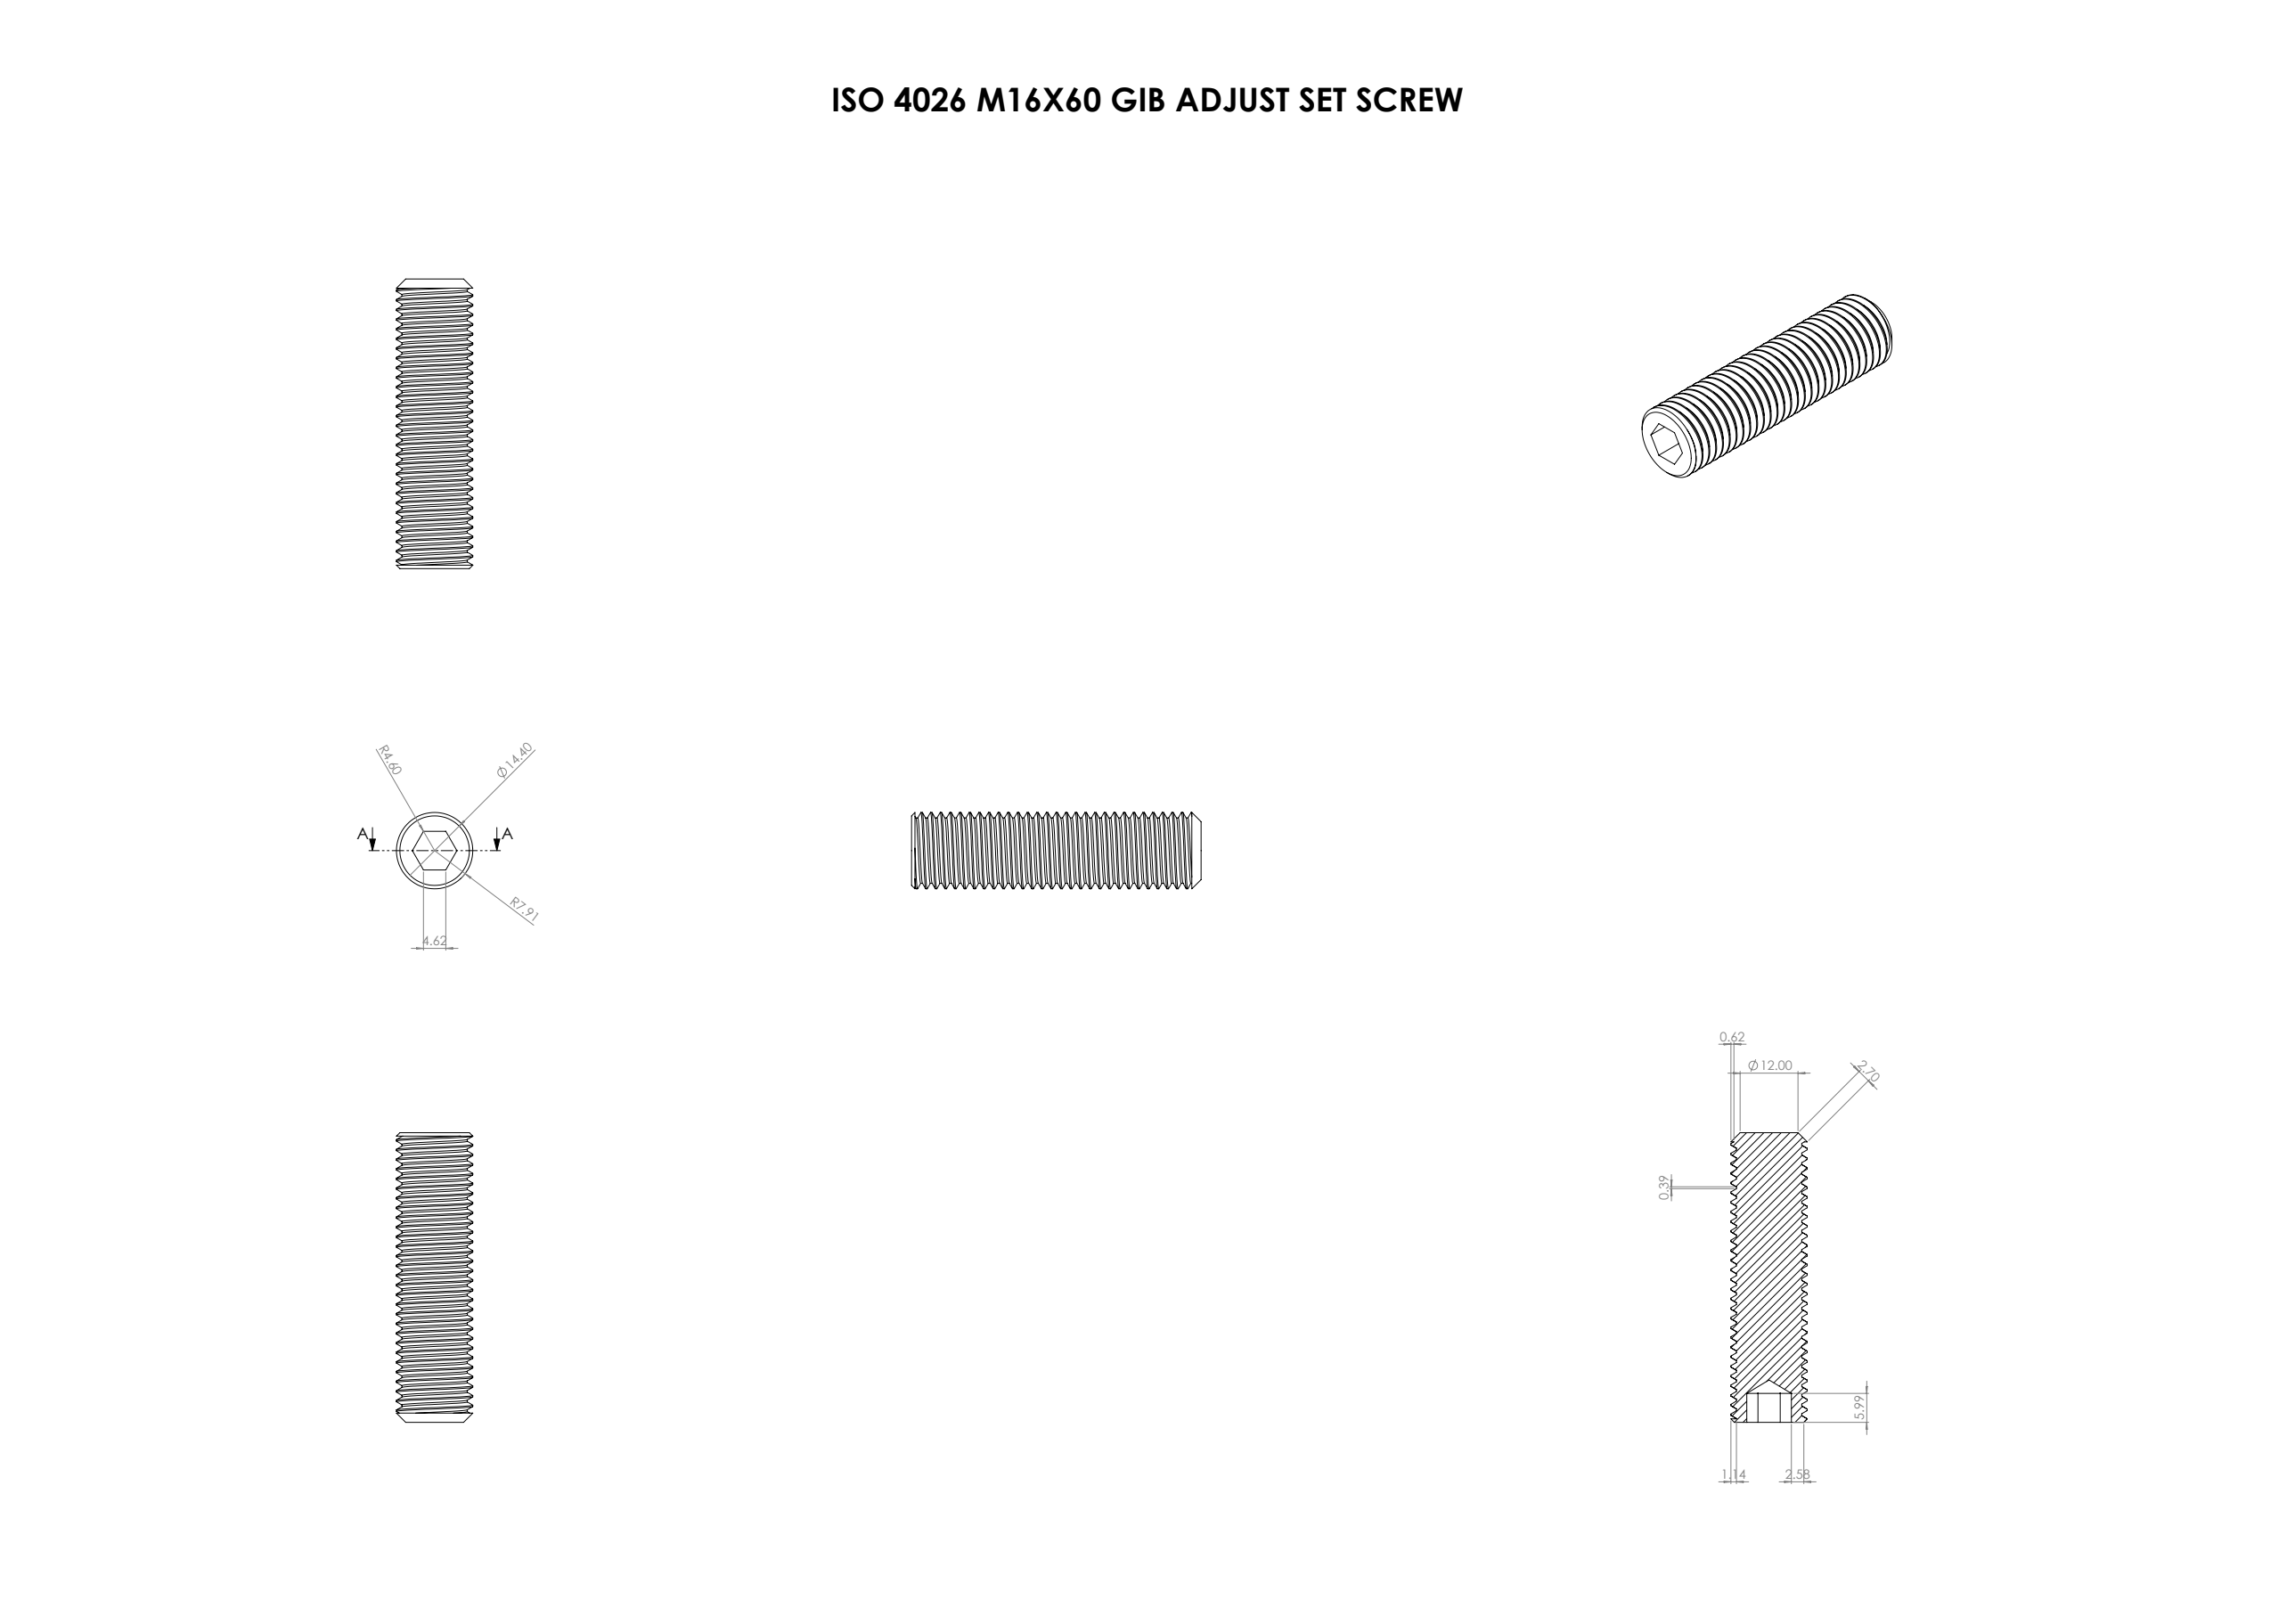
ISO-10303-21;
HEADER;
/* Generated by software containing ST-Developer
 * from STEP Tools, Inc. (www.steptools.com) 
 */

FILE_DESCRIPTION(
/* description */ (''),
/* implementation_level */ '2;1');

FILE_NAME(
/* name */ '11_ISO_4026_M16x60_Gib_Adjust_Set_Screw.step',
/* time_stamp */ '2026-10-19T23:58:09-07:00',
/* author */ (''),
/* organization */ (''),
/* preprocessor_version */ 'ST-DEVELOPER v20.2',
/* originating_system */ 'Autodesk Translation Framework v15.15.0.0',
/* authorisation */ '');

FILE_SCHEMA (('AP203_CONFIGURATION_CONTROLLED_3D_DESIGN_OF_MECHANICAL_PARTS_AND_ASSEMBLIES_MIM_LF { 1 0 10303 203 3 1 4 }',
'AUTOMOTIVE_DESIGN { 1 0 10303 214 3 1 1 }','INTEGRATED_CNC_SCHEMA','MODEL_BASED_INTEGRATED_MANUFACTURING_SCHEMA',
'PROCESS_PLANNING_SCHEMA','AP242_MANAGED_MODEL_BASED_3D_ENGINEERING_MIM_LF { 1 0 10303 442 3 1 4 }'));
ENDSEC;

DATA;
#10=MECHANICAL_DESIGN_GEOMETRIC_PRESENTATION_REPRESENTATION('',(#414),#70757);
#215=(
BOUNDED_CURVE()
B_SPLINE_CURVE(2,(#54486,#54487,#54488),.UNSPECIFIED.,.F.,.F.)
B_SPLINE_CURVE_WITH_KNOTS((3,3),(0.,0.00348603246849772),.UNSPECIFIED.)
CURVE()
GEOMETRIC_REPRESENTATION_ITEM()
RATIONAL_B_SPLINE_CURVE((1.,1.00000655818292,1.))
REPRESENTATION_ITEM('')
);
#216=(
BOUNDED_CURVE()
B_SPLINE_CURVE(2,(#54490,#54491,#54492),.UNSPECIFIED.,.F.,.F.)
B_SPLINE_CURVE_WITH_KNOTS((3,3),(0.,0.0034860324684977),.UNSPECIFIED.)
CURVE()
GEOMETRIC_REPRESENTATION_ITEM()
RATIONAL_B_SPLINE_CURVE((1.,1.00000655824651,1.))
REPRESENTATION_ITEM('')
);
#217=(
BOUNDED_CURVE()
B_SPLINE_CURVE(2,(#54495,#54496,#54497),.UNSPECIFIED.,.F.,.F.)
B_SPLINE_CURVE_WITH_KNOTS((3,3),(0.,0.00348603246849777),.UNSPECIFIED.)
CURVE()
GEOMETRIC_REPRESENTATION_ITEM()
RATIONAL_B_SPLINE_CURVE((1.,1.00000655828125,1.))
REPRESENTATION_ITEM('')
);
#218=(
BOUNDED_CURVE()
B_SPLINE_CURVE(2,(#54499,#54500,#54501),.UNSPECIFIED.,.F.,.F.)
B_SPLINE_CURVE_WITH_KNOTS((3,3),(0.,0.00348603246849785),.UNSPECIFIED.)
CURVE()
GEOMETRIC_REPRESENTATION_ITEM()
RATIONAL_B_SPLINE_CURVE((1.,1.00000655858972,1.))
REPRESENTATION_ITEM('')
);
#219=(
BOUNDED_CURVE()
B_SPLINE_CURVE(2,(#54504,#54505,#54506),.UNSPECIFIED.,.F.,.F.)
B_SPLINE_CURVE_WITH_KNOTS((3,3),(0.,0.00348603246849743),.UNSPECIFIED.)
CURVE()
GEOMETRIC_REPRESENTATION_ITEM()
RATIONAL_B_SPLINE_CURVE((1.,1.00000655826316,1.))
REPRESENTATION_ITEM('')
);
#220=(
BOUNDED_CURVE()
B_SPLINE_CURVE(2,(#54508,#54509,#54510),.UNSPECIFIED.,.F.,.F.)
B_SPLINE_CURVE_WITH_KNOTS((3,3),(0.,0.00348603246849747),.UNSPECIFIED.)
CURVE()
GEOMETRIC_REPRESENTATION_ITEM()
RATIONAL_B_SPLINE_CURVE((1.,1.00000655837246,1.))
REPRESENTATION_ITEM('')
);
#221=(
BOUNDED_CURVE()
B_SPLINE_CURVE(2,(#54513,#54514,#54515),.UNSPECIFIED.,.F.,.F.)
B_SPLINE_CURVE_WITH_KNOTS((3,3),(0.,0.00348603246849727),.UNSPECIFIED.)
CURVE()
GEOMETRIC_REPRESENTATION_ITEM()
RATIONAL_B_SPLINE_CURVE((1.,1.00000655774933,1.))
REPRESENTATION_ITEM('')
);
#222=(
BOUNDED_CURVE()
B_SPLINE_CURVE(2,(#54517,#54518,#54519),.UNSPECIFIED.,.F.,.F.)
B_SPLINE_CURVE_WITH_KNOTS((3,3),(0.,0.00348603246849747),.UNSPECIFIED.)
CURVE()
GEOMETRIC_REPRESENTATION_ITEM()
RATIONAL_B_SPLINE_CURVE((1.,1.00000655778188,1.))
REPRESENTATION_ITEM('')
);
#223=(
BOUNDED_CURVE()
B_SPLINE_CURVE(2,(#54522,#54523,#54524),.UNSPECIFIED.,.F.,.F.)
B_SPLINE_CURVE_WITH_KNOTS((3,3),(0.,0.00348603246849769),.UNSPECIFIED.)
CURVE()
GEOMETRIC_REPRESENTATION_ITEM()
RATIONAL_B_SPLINE_CURVE((1.,1.00000655825998,1.))
REPRESENTATION_ITEM('')
);
#224=(
BOUNDED_CURVE()
B_SPLINE_CURVE(2,(#54526,#54527,#54528),.UNSPECIFIED.,.F.,.F.)
B_SPLINE_CURVE_WITH_KNOTS((3,3),(0.,0.00348603246849761),.UNSPECIFIED.)
CURVE()
GEOMETRIC_REPRESENTATION_ITEM()
RATIONAL_B_SPLINE_CURVE((1.,1.00000655838487,1.))
REPRESENTATION_ITEM('')
);
#225=(
BOUNDED_CURVE()
B_SPLINE_CURVE(2,(#54531,#54532,#54533),.UNSPECIFIED.,.F.,.F.)
B_SPLINE_CURVE_WITH_KNOTS((3,3),(0.,0.00348603246849764),.UNSPECIFIED.)
CURVE()
GEOMETRIC_REPRESENTATION_ITEM()
RATIONAL_B_SPLINE_CURVE((1.,1.00000655822052,1.))
REPRESENTATION_ITEM('')
);
#226=(
BOUNDED_CURVE()
B_SPLINE_CURVE(2,(#54535,#54536,#54537),.UNSPECIFIED.,.F.,.F.)
B_SPLINE_CURVE_WITH_KNOTS((3,3),(0.,0.00348603246849749),.UNSPECIFIED.)
CURVE()
GEOMETRIC_REPRESENTATION_ITEM()
RATIONAL_B_SPLINE_CURVE((1.,1.00000655832735,1.))
REPRESENTATION_ITEM('')
);
#276=B_SPLINE_SURFACE_WITH_KNOTS('',3,3,((#51283,#51284,#51285,#51286,#51287,
#51288,#51289,#51290,#51291,#51292,#51293,#51294,#51295,#51296,#51297,#51298,
#51299,#51300,#51301,#51302,#51303,#51304,#51305,#51306,#51307,#51308,#51309,
#51310,#51311,#51312,#51313,#51314,#51315,#51316,#51317,#51318,#51319,#51320,
#51321,#51322,#51323,#51324,#51325,#51326,#51327,#51328,#51329,#51330,#51331,
#51332,#51333,#51334,#51335,#51336,#51337,#51338,#51339,#51340,#51341,#51342,
#51343,#51344,#51345,#51346,#51347,#51348,#51349,#51350,#51351,#51352,#51353,
#51354,#51355,#51356,#51357,#51358,#51359,#51360,#51361,#51362,#51363,#51364,
#51365,#51366,#51367,#51368,#51369,#51370,#51371,#51372,#51373,#51374,#51375,
#51376,#51377,#51378,#51379,#51380,#51381,#51382,#51383,#51384,#51385,#51386,
#51387,#51388,#51389,#51390,#51391,#51392,#51393,#51394,#51395,#51396,#51397,
#51398,#51399,#51400,#51401,#51402,#51403,#51404,#51405,#51406,#51407,#51408,
#51409,#51410,#51411,#51412,#51413,#51414,#51415,#51416,#51417,#51418,#51419,
#51420,#51421,#51422,#51423,#51424,#51425,#51426,#51427,#51428,#51429,#51430,
#51431,#51432,#51433,#51434,#51435,#51436,#51437,#51438,#51439,#51440,#51441,
#51442,#51443,#51444,#51445,#51446,#51447,#51448,#51449,#51450,#51451,#51452,
#51453,#51454,#51455,#51456,#51457,#51458,#51459,#51460,#51461,#51462,#51463,
#51464,#51465,#51466,#51467,#51468,#51469,#51470,#51471,#51472,#51473,#51474,
#51475,#51476,#51477,#51478,#51479,#51480,#51481,#51482,#51483,#51484,#51485,
#51486,#51487,#51488,#51489,#51490,#51491,#51492,#51493,#51494,#51495,#51496,
#51497,#51498,#51499,#51500,#51501,#51502,#51503,#51504,#51505,#51506,#51507,
#51508,#51509,#51510,#51511,#51512,#51513,#51514,#51515,#51516,#51517,#51518,
#51519,#51520,#51521,#51522,#51523,#51524,#51525,#51526,#51527,#51528,#51529,
#51530,#51531,#51532,#51533,#51534,#51535,#51536,#51537,#51538,#51539,#51540,
#51541,#51542,#51543,#51544,#51545,#51546,#51547,#51548,#51549,#51550,#51551,
#51552,#51553,#51554,#51555,#51556,#51557,#51558,#51559,#51560,#51561,#51562,
#51563,#51564,#51565,#51566,#51567,#51568,#51569,#51570,#51571,#51572,#51573,
#51574,#51575,#51576,#51577,#51578,#51579,#51580,#51581,#51582,#51583,#51584,
#51585,#51586,#51587,#51588,#51589,#51590,#51591,#51592,#51593,#51594,#51595,
#51596,#51597,#51598,#51599,#51600,#51601,#51602,#51603,#51604,#51605,#51606,
#51607,#51608,#51609,#51610,#51611,#51612,#51613,#51614,#51615,#51616,#51617,
#51618,#51619,#51620,#51621,#51622,#51623,#51624,#51625,#51626,#51627,#51628,
#51629,#51630,#51631,#51632,#51633,#51634,#51635,#51636,#51637,#51638,#51639,
#51640,#51641,#51642,#51643,#51644,#51645,#51646,#51647,#51648,#51649,#51650,
#51651),(#51652,#51653,#51654,#51655,#51656,#51657,#51658,#51659,#51660,
#51661,#51662,#51663,#51664,#51665,#51666,#51667,#51668,#51669,#51670,#51671,
#51672,#51673,#51674,#51675,#51676,#51677,#51678,#51679,#51680,#51681,#51682,
#51683,#51684,#51685,#51686,#51687,#51688,#51689,#51690,#51691,#51692,#51693,
#51694,#51695,#51696,#51697,#51698,#51699,#51700,#51701,#51702,#51703,#51704,
#51705,#51706,#51707,#51708,#51709,#51710,#51711,#51712,#51713,#51714,#51715,
#51716,#51717,#51718,#51719,#51720,#51721,#51722,#51723,#51724,#51725,#51726,
#51727,#51728,#51729,#51730,#51731,#51732,#51733,#51734,#51735,#51736,#51737,
#51738,#51739,#51740,#51741,#51742,#51743,#51744,#51745,#51746,#51747,#51748,
#51749,#51750,#51751,#51752,#51753,#51754,#51755,#51756,#51757,#51758,#51759,
#51760,#51761,#51762,#51763,#51764,#51765,#51766,#51767,#51768,#51769,#51770,
#51771,#51772,#51773,#51774,#51775,#51776,#51777,#51778,#51779,#51780,#51781,
#51782,#51783,#51784,#51785,#51786,#51787,#51788,#51789,#51790,#51791,#51792,
#51793,#51794,#51795,#51796,#51797,#51798,#51799,#51800,#51801,#51802,#51803,
#51804,#51805,#51806,#51807,#51808,#51809,#51810,#51811,#51812,#51813,#51814,
#51815,#51816,#51817,#51818,#51819,#51820,#51821,#51822,#51823,#51824,#51825,
#51826,#51827,#51828,#51829,#51830,#51831,#51832,#51833,#51834,#51835,#51836,
#51837,#51838,#51839,#51840,#51841,#51842,#51843,#51844,#51845,#51846,#51847,
#51848,#51849,#51850,#51851,#51852,#51853,#51854,#51855,#51856,#51857,#51858,
#51859,#51860,#51861,#51862,#51863,#51864,#51865,#51866,#51867,#51868,#51869,
#51870,#51871,#51872,#51873,#51874,#51875,#51876,#51877,#51878,#51879,#51880,
#51881,#51882,#51883,#51884,#51885,#51886,#51887,#51888,#51889,#51890,#51891,
#51892,#51893,#51894,#51895,#51896,#51897,#51898,#51899,#51900,#51901,#51902,
#51903,#51904,#51905,#51906,#51907,#51908,#51909,#51910,#51911,#51912,#51913,
#51914,#51915,#51916,#51917,#51918,#51919,#51920,#51921,#51922,#51923,#51924,
#51925,#51926,#51927,#51928,#51929,#51930,#51931,#51932,#51933,#51934,#51935,
#51936,#51937,#51938,#51939,#51940,#51941,#51942,#51943,#51944,#51945,#51946,
#51947,#51948,#51949,#51950,#51951,#51952,#51953,#51954,#51955,#51956,#51957,
#51958,#51959,#51960,#51961,#51962,#51963,#51964,#51965,#51966,#51967,#51968,
#51969,#51970,#51971,#51972,#51973,#51974,#51975,#51976,#51977,#51978,#51979,
#51980,#51981,#51982,#51983,#51984,#51985,#51986,#51987,#51988,#51989,#51990,
#51991,#51992,#51993,#51994,#51995,#51996,#51997,#51998,#51999,#52000,#52001,
#52002,#52003,#52004,#52005,#52006,#52007,#52008,#52009,#52010,#52011,#52012,
#52013,#52014,#52015,#52016,#52017,#52018,#52019,#52020),(#52021,#52022,
#52023,#52024,#52025,#52026,#52027,#52028,#52029,#52030,#52031,#52032,#52033,
#52034,#52035,#52036,#52037,#52038,#52039,#52040,#52041,#52042,#52043,#52044,
#52045,#52046,#52047,#52048,#52049,#52050,#52051,#52052,#52053,#52054,#52055,
#52056,#52057,#52058,#52059,#52060,#52061,#52062,#52063,#52064,#52065,#52066,
#52067,#52068,#52069,#52070,#52071,#52072,#52073,#52074,#52075,#52076,#52077,
#52078,#52079,#52080,#52081,#52082,#52083,#52084,#52085,#52086,#52087,#52088,
#52089,#52090,#52091,#52092,#52093,#52094,#52095,#52096,#52097,#52098,#52099,
#52100,#52101,#52102,#52103,#52104,#52105,#52106,#52107,#52108,#52109,#52110,
#52111,#52112,#52113,#52114,#52115,#52116,#52117,#52118,#52119,#52120,#52121,
#52122,#52123,#52124,#52125,#52126,#52127,#52128,#52129,#52130,#52131,#52132,
#52133,#52134,#52135,#52136,#52137,#52138,#52139,#52140,#52141,#52142,#52143,
#52144,#52145,#52146,#52147,#52148,#52149,#52150,#52151,#52152,#52153,#52154,
#52155,#52156,#52157,#52158,#52159,#52160,#52161,#52162,#52163,#52164,#52165,
#52166,#52167,#52168,#52169,#52170,#52171,#52172,#52173,#52174,#52175,#52176,
#52177,#52178,#52179,#52180,#52181,#52182,#52183,#52184,#52185,#52186,#52187,
#52188,#52189,#52190,#52191,#52192,#52193,#52194,#52195,#52196,#52197,#52198,
#52199,#52200,#52201,#52202,#52203,#52204,#52205,#52206,#52207,#52208,#52209,
#52210,#52211,#52212,#52213,#52214,#52215,#52216,#52217,#52218,#52219,#52220,
#52221,#52222,#52223,#52224,#52225,#52226,#52227,#52228,#52229,#52230,#52231,
#52232,#52233,#52234,#52235,#52236,#52237,#52238,#52239,#52240,#52241,#52242,
#52243,#52244,#52245,#52246,#52247,#52248,#52249,#52250,#52251,#52252,#52253,
#52254,#52255,#52256,#52257,#52258,#52259,#52260,#52261,#52262,#52263,#52264,
#52265,#52266,#52267,#52268,#52269,#52270,#52271,#52272,#52273,#52274,#52275,
#52276,#52277,#52278,#52279,#52280,#52281,#52282,#52283,#52284,#52285,#52286,
#52287,#52288,#52289,#52290,#52291,#52292,#52293,#52294,#52295,#52296,#52297,
#52298,#52299,#52300,#52301,#52302,#52303,#52304,#52305,#52306,#52307,#52308,
#52309,#52310,#52311,#52312,#52313,#52314,#52315,#52316,#52317,#52318,#52319,
#52320,#52321,#52322,#52323,#52324,#52325,#52326,#52327,#52328,#52329,#52330,
#52331,#52332,#52333,#52334,#52335,#52336,#52337,#52338,#52339,#52340,#52341,
#52342,#52343,#52344,#52345,#52346,#52347,#52348,#52349,#52350,#52351,#52352,
#52353,#52354,#52355,#52356,#52357,#52358,#52359,#52360,#52361,#52362,#52363,
#52364,#52365,#52366,#52367,#52368,#52369,#52370,#52371,#52372,#52373,#52374,
#52375,#52376,#52377,#52378,#52379,#52380,#52381,#52382,#52383,#52384,#52385,
#52386,#52387,#52388,#52389),(#52390,#52391,#52392,#52393,#52394,#52395,
#52396,#52397,#52398,#52399,#52400,#52401,#52402,#52403,#52404,#52405,#52406,
#52407,#52408,#52409,#52410,#52411,#52412,#52413,#52414,#52415,#52416,#52417,
#52418,#52419,#52420,#52421,#52422,#52423,#52424,#52425,#52426,#52427,#52428,
#52429,#52430,#52431,#52432,#52433,#52434,#52435,#52436,#52437,#52438,#52439,
#52440,#52441,#52442,#52443,#52444,#52445,#52446,#52447,#52448,#52449,#52450,
#52451,#52452,#52453,#52454,#52455,#52456,#52457,#52458,#52459,#52460,#52461,
#52462,#52463,#52464,#52465,#52466,#52467,#52468,#52469,#52470,#52471,#52472,
#52473,#52474,#52475,#52476,#52477,#52478,#52479,#52480,#52481,#52482,#52483,
#52484,#52485,#52486,#52487,#52488,#52489,#52490,#52491,#52492,#52493,#52494,
#52495,#52496,#52497,#52498,#52499,#52500,#52501,#52502,#52503,#52504,#52505,
#52506,#52507,#52508,#52509,#52510,#52511,#52512,#52513,#52514,#52515,#52516,
#52517,#52518,#52519,#52520,#52521,#52522,#52523,#52524,#52525,#52526,#52527,
#52528,#52529,#52530,#52531,#52532,#52533,#52534,#52535,#52536,#52537,#52538,
#52539,#52540,#52541,#52542,#52543,#52544,#52545,#52546,#52547,#52548,#52549,
#52550,#52551,#52552,#52553,#52554,#52555,#52556,#52557,#52558,#52559,#52560,
#52561,#52562,#52563,#52564,#52565,#52566,#52567,#52568,#52569,#52570,#52571,
#52572,#52573,#52574,#52575,#52576,#52577,#52578,#52579,#52580,#52581,#52582,
#52583,#52584,#52585,#52586,#52587,#52588,#52589,#52590,#52591,#52592,#52593,
#52594,#52595,#52596,#52597,#52598,#52599,#52600,#52601,#52602,#52603,#52604,
#52605,#52606,#52607,#52608,#52609,#52610,#52611,#52612,#52613,#52614,#52615,
#52616,#52617,#52618,#52619,#52620,#52621,#52622,#52623,#52624,#52625,#52626,
#52627,#52628,#52629,#52630,#52631,#52632,#52633,#52634,#52635,#52636,#52637,
#52638,#52639,#52640,#52641,#52642,#52643,#52644,#52645,#52646,#52647,#52648,
#52649,#52650,#52651,#52652,#52653,#52654,#52655,#52656,#52657,#52658,#52659,
#52660,#52661,#52662,#52663,#52664,#52665,#52666,#52667,#52668,#52669,#52670,
#52671,#52672,#52673,#52674,#52675,#52676,#52677,#52678,#52679,#52680,#52681,
#52682,#52683,#52684,#52685,#52686,#52687,#52688,#52689,#52690,#52691,#52692,
#52693,#52694,#52695,#52696,#52697,#52698,#52699,#52700,#52701,#52702,#52703,
#52704,#52705,#52706,#52707,#52708,#52709,#52710,#52711,#52712,#52713,#52714,
#52715,#52716,#52717,#52718,#52719,#52720,#52721,#52722,#52723,#52724,#52725,
#52726,#52727,#52728,#52729,#52730,#52731,#52732,#52733,#52734,#52735,#52736,
#52737,#52738,#52739,#52740,#52741,#52742,#52743,#52744,#52745,#52746,#52747,
#52748,#52749,#52750,#52751,#52752,#52753,#52754,#52755,#52756,#52757,#52758)),
 .UNSPECIFIED.,.F.,.F.,.F.,(4,4),(4,1,1,1,1,1,1,1,1,1,1,1,1,1,1,1,1,1,1,
1,1,1,1,1,1,1,1,1,1,1,1,1,1,1,1,1,1,1,1,1,1,1,1,1,1,1,1,1,1,1,1,1,1,1,1,
1,1,1,1,1,1,1,1,1,1,1,1,1,1,1,1,1,1,1,1,1,1,1,1,1,1,1,1,1,1,1,1,1,1,1,1,
1,1,1,1,1,1,1,1,1,1,1,1,1,1,1,1,1,1,1,1,1,1,1,1,1,1,1,1,1,1,1,1,1,1,1,1,
1,1,1,1,1,1,1,1,1,1,1,1,1,1,1,1,1,1,1,1,1,1,1,1,1,1,1,1,1,1,1,1,1,1,1,1,
1,1,1,1,1,1,1,1,1,1,1,1,1,1,1,1,1,1,1,1,1,1,1,1,1,1,1,1,1,1,1,1,1,1,1,1,
1,1,1,1,1,1,1,1,1,1,1,1,1,1,1,1,1,1,1,1,1,1,1,1,1,1,1,1,1,1,1,1,1,1,1,1,
1,1,1,1,1,1,1,1,1,1,1,1,1,1,1,1,1,1,1,1,1,1,1,1,1,1,1,1,1,1,1,1,1,1,1,1,
1,1,1,1,1,1,1,1,1,1,1,1,1,1,1,1,1,1,1,1,1,1,1,1,1,1,1,1,1,1,1,1,1,1,1,1,
1,1,1,1,1,1,1,1,1,1,1,1,1,1,1,1,1,1,1,1,1,1,1,1,1,1,1,1,1,1,1,1,1,1,1,1,
1,1,1,1,1,1,1,1,1,1,1,1,1,1,1,1,1,1,1,1,1,1,1,4),(0.,0.132097741590586),
(8.30112925462635,8.79930764192242,9.29748602921848,9.79566441651454,10.2938428038106,
10.7920211911067,11.2901995784027,11.7883779656988,12.2865563529949,12.7847347402909,
13.282913127587,13.781091514883,14.2792699021791,14.7774482894752,15.2756266767712,
15.7738050640673,16.2719834513634,16.7701618386594,17.2683402259555,17.7665186132516,
18.2646970005476,18.7628753878437,19.2610537751397,19.7592321624358,20.2574105497319,
20.7555889370279,21.253767324324,21.7519457116201,22.2501240989161,22.7483024862122,
23.2464808735082,23.7446592608043,24.2428376481004,24.7410160353964,25.2391944226925,
25.7373728099886,26.2355511972846,26.7337295845807,27.2319079718768,27.7300863591728,
28.2282647464689,28.7264431337649,29.224621521061,29.7227999083571,30.2209782956531,
30.7191566829492,31.2173350702453,31.7155134575413,32.2136918448374,32.7118702321334,
33.2100486194295,33.7082270067256,34.2064053940216,34.7045837813177,35.2027621686138,
35.7009405559098,36.1991189432059,36.697297330502,37.195475717798,37.6936541050941,
38.1918324923901,38.6900108796862,39.1881892669823,39.6863676542783,40.1845460415744,
40.6827244288705,41.1809028161665,41.6790812034626,42.1772595907587,42.6754379780547,
43.1736163653508,43.6717947526468,44.1699731399429,44.668151527239,45.166329914535,
45.6645083018311,46.1626866891272,46.6608650764232,47.1590434637193,47.6572218510153,
48.1554002383114,48.6535786256075,49.1517570129035,49.6499354001996,50.1481137874957,
50.6462921747917,51.1444705620878,51.6426489493839,52.1408273366799,52.639005723976,
53.137184111272,53.6353624985681,54.1335408858642,54.6317192731602,55.1298976604563,
55.6280760477524,56.1262544350484,56.6244328223445,57.1226112096405,57.6207895969366,
58.1189679842327,58.6171463715287,59.1153247588248,59.6135031461209,60.1116815334169,
60.609859920713,61.108038308009,61.6062166953051,62.1043950826012,62.6025734698972,
63.1007518571933,63.5989302444894,64.0971086317854,64.5952870190815,65.0934654063776,
65.5916437936736,66.0898221809697,66.5880005682658,67.0861789555618,67.5843573428579,
68.0825357301539,68.58071411745,69.0788925047461,69.5770708920421,70.0752492793382,
70.5734276666342,71.0716060539303,71.5697844412264,72.0679628285224,72.5661412158185,
73.0643196031146,73.5624979904106,74.0606763777067,74.5588547650028,75.0570331522988,
75.5552115395949,76.053389926891,76.551568314187,77.0497467014831,77.5479250887791,
78.0461034760752,78.5442818633713,79.0424602506673,79.5406386379634,80.0388170252594,
80.5369954125555,81.0351737998516,81.5333521871476,82.0315305744437,82.5297089617398,
83.0278873490358,83.5260657363319,84.024244123628,84.522422510924,85.0206008982201,
85.5187792855161,86.0169576728122,86.5151360601083,87.0133144474043,87.5114928347004,
88.0096712219965,88.5078496092925,89.0060279965886,89.5042063838847,90.0023847711807,
90.5005631584768,90.9987415457728,91.4969199330689,91.995098320365,92.493276707661,
92.9914550949571,93.4896334822532,93.9878118695492,94.4859902568453,94.9841686441413,
95.4823470314374,95.9805254187335,96.4787038060295,96.9768821933256,97.4750605806217,
97.9732389679177,98.4714173552138,98.9695957425099,99.4677741298059,99.965952517102,
100.464130904398,100.962309291694,101.46048767899,101.958666066286,102.456844453582,
102.955022840878,103.453201228174,103.95137961547,104.449558002767,104.947736390063,
105.445914777359,105.944093164655,106.442271551951,106.940449939247,107.438628326543,
107.936806713839,108.434985101135,108.933163488431,109.431341875727,109.929520263023,
110.427698650319,110.925877037615,111.424055424911,111.922233812207,112.420412199504,
112.9185905868,113.416768974096,113.914947361392,114.413125748688,114.911304135984,
115.40948252328,115.907660910576,116.405839297872,116.904017685168,117.402196072464,
117.90037445976,118.398552847056,118.896731234352,119.394909621648,119.893088008945,
120.391266396241,120.889444783537,121.387623170833,121.885801558129,122.383979945425,
122.882158332721,123.380336720017,123.878515107313,124.376693494609,124.874871881905,
125.373050269201,125.871228656497,126.369407043793,126.867585431089,127.365763818385,
127.863942205682,128.362120592978,128.860298980274,129.35847736757,129.856655754866,
130.354834142162,130.853012529458,131.351190916754,131.84936930405,132.347547691346,
132.845726078642,133.343904465938,133.842082853234,134.34026124053,134.838439627826,
135.336618015122,135.834796402419,136.332974789715,136.831153177011,137.329331564307,
137.827509951603,138.325688338899,138.823866726195,139.322045113491,139.820223500787,
140.318401888083,140.816580275379,141.314758662675,141.812937049971,142.311115437267,
142.809293824563,143.307472211859,143.805650599156,144.303828986452,144.802007373748,
145.300185761044,145.79836414834,146.296542535636,146.794720922932,147.292899310228,
147.791077697524,148.28925608482,148.787434472116,149.285612859412,149.783791246708,
150.281969634004,150.7801480213,151.278326408596,151.776504795893,152.274683183189,
152.772861570485,153.271039957781,153.769218345077,154.267396732373,154.765575119669,
155.263753506965,155.761931894261,156.260110281557,156.758288668853,157.256467056149,
157.754645443445,158.252823830741,158.751002218037,159.249180605333,159.74735899263,
160.245537379926,160.743715767222,161.241894154518,161.740072541814,162.23825092911,
162.736429316406,163.234607703702,163.732786090998,164.230964478294,164.72914286559,
165.227321252886,165.725499640182,166.223678027478,166.721856414774,167.220034802071,
167.718213189367,168.216391576663,168.714569963959,169.212748351255,169.710926738551,
170.209105125847,170.707283513143,171.205461900439,171.703640287735,172.201818675031,
172.699997062327,173.198175449623,173.696353836919,174.194532224215,174.692710611511,
175.190888998808,175.689067386104,176.1872457734,176.685424160696,177.183602547992,
177.681780935288,178.179959322584,178.67813770988,179.176316097176,179.674494484472,
180.172672871768,180.670851259064,181.16902964636,181.667208033656,182.165386420952,
182.663564808248,183.161743195545,183.659921582841,184.158099970137,184.656278357433,
185.154456744729,185.652635132025,186.150813519321,186.648991906617,187.147170293913,
187.645348681209,188.143527068505,188.641705455801,189.139883843097,189.638062230393,
190.136240617689,190.634419004985),.UNSPECIFIED.);
#277=B_SPLINE_SURFACE_WITH_KNOTS('',3,3,((#52964,#52965,#52966,#52967,#52968,
#52969,#52970,#52971,#52972,#52973,#52974,#52975,#52976,#52977,#52978,#52979,
#52980,#52981,#52982,#52983,#52984,#52985,#52986,#52987,#52988,#52989,#52990,
#52991,#52992,#52993,#52994,#52995,#52996,#52997,#52998,#52999,#53000,#53001,
#53002,#53003,#53004,#53005,#53006,#53007,#53008,#53009,#53010,#53011,#53012,
#53013,#53014,#53015,#53016,#53017,#53018,#53019,#53020,#53021,#53022,#53023,
#53024,#53025,#53026,#53027,#53028,#53029,#53030,#53031,#53032,#53033,#53034,
#53035,#53036,#53037,#53038,#53039,#53040,#53041,#53042,#53043,#53044,#53045,
#53046,#53047,#53048,#53049,#53050,#53051,#53052,#53053,#53054,#53055,#53056,
#53057,#53058,#53059,#53060,#53061,#53062,#53063,#53064,#53065,#53066,#53067,
#53068,#53069,#53070,#53071,#53072,#53073,#53074,#53075,#53076,#53077,#53078,
#53079,#53080,#53081,#53082,#53083,#53084,#53085,#53086,#53087,#53088,#53089,
#53090,#53091,#53092,#53093,#53094,#53095,#53096,#53097,#53098,#53099,#53100,
#53101,#53102,#53103,#53104,#53105,#53106,#53107,#53108,#53109,#53110,#53111,
#53112,#53113,#53114,#53115,#53116,#53117,#53118,#53119,#53120,#53121,#53122,
#53123,#53124,#53125,#53126,#53127,#53128,#53129,#53130,#53131,#53132,#53133,
#53134,#53135,#53136,#53137,#53138,#53139,#53140,#53141,#53142,#53143,#53144,
#53145,#53146,#53147,#53148,#53149,#53150,#53151,#53152,#53153,#53154,#53155,
#53156,#53157,#53158,#53159,#53160,#53161,#53162,#53163,#53164,#53165,#53166,
#53167,#53168,#53169,#53170,#53171,#53172,#53173,#53174,#53175,#53176,#53177,
#53178,#53179,#53180,#53181,#53182,#53183,#53184,#53185,#53186,#53187,#53188,
#53189,#53190,#53191,#53192,#53193,#53194,#53195,#53196,#53197,#53198,#53199,
#53200,#53201,#53202,#53203,#53204,#53205,#53206,#53207,#53208,#53209,#53210,
#53211,#53212,#53213,#53214,#53215,#53216,#53217,#53218,#53219,#53220,#53221,
#53222,#53223,#53224,#53225,#53226,#53227,#53228,#53229,#53230,#53231,#53232,
#53233,#53234,#53235,#53236,#53237,#53238,#53239,#53240,#53241,#53242,#53243,
#53244,#53245,#53246,#53247,#53248,#53249,#53250,#53251,#53252,#53253,#53254,
#53255,#53256,#53257,#53258,#53259,#53260,#53261,#53262,#53263,#53264,#53265,
#53266,#53267,#53268,#53269,#53270,#53271,#53272,#53273,#53274,#53275,#53276,
#53277,#53278,#53279,#53280,#53281,#53282,#53283,#53284,#53285,#53286,#53287,
#53288,#53289,#53290,#53291,#53292,#53293,#53294,#53295,#53296,#53297,#53298,
#53299,#53300,#53301,#53302,#53303,#53304,#53305,#53306,#53307,#53308,#53309,
#53310,#53311,#53312,#53313,#53314,#53315,#53316,#53317,#53318,#53319,#53320,
#53321,#53322,#53323,#53324,#53325,#53326,#53327,#53328,#53329,#53330,#53331,
#53332),(#53333,#53334,#53335,#53336,#53337,#53338,#53339,#53340,#53341,
#53342,#53343,#53344,#53345,#53346,#53347,#53348,#53349,#53350,#53351,#53352,
#53353,#53354,#53355,#53356,#53357,#53358,#53359,#53360,#53361,#53362,#53363,
#53364,#53365,#53366,#53367,#53368,#53369,#53370,#53371,#53372,#53373,#53374,
#53375,#53376,#53377,#53378,#53379,#53380,#53381,#53382,#53383,#53384,#53385,
#53386,#53387,#53388,#53389,#53390,#53391,#53392,#53393,#53394,#53395,#53396,
#53397,#53398,#53399,#53400,#53401,#53402,#53403,#53404,#53405,#53406,#53407,
#53408,#53409,#53410,#53411,#53412,#53413,#53414,#53415,#53416,#53417,#53418,
#53419,#53420,#53421,#53422,#53423,#53424,#53425,#53426,#53427,#53428,#53429,
#53430,#53431,#53432,#53433,#53434,#53435,#53436,#53437,#53438,#53439,#53440,
#53441,#53442,#53443,#53444,#53445,#53446,#53447,#53448,#53449,#53450,#53451,
#53452,#53453,#53454,#53455,#53456,#53457,#53458,#53459,#53460,#53461,#53462,
#53463,#53464,#53465,#53466,#53467,#53468,#53469,#53470,#53471,#53472,#53473,
#53474,#53475,#53476,#53477,#53478,#53479,#53480,#53481,#53482,#53483,#53484,
#53485,#53486,#53487,#53488,#53489,#53490,#53491,#53492,#53493,#53494,#53495,
#53496,#53497,#53498,#53499,#53500,#53501,#53502,#53503,#53504,#53505,#53506,
#53507,#53508,#53509,#53510,#53511,#53512,#53513,#53514,#53515,#53516,#53517,
#53518,#53519,#53520,#53521,#53522,#53523,#53524,#53525,#53526,#53527,#53528,
#53529,#53530,#53531,#53532,#53533,#53534,#53535,#53536,#53537,#53538,#53539,
#53540,#53541,#53542,#53543,#53544,#53545,#53546,#53547,#53548,#53549,#53550,
#53551,#53552,#53553,#53554,#53555,#53556,#53557,#53558,#53559,#53560,#53561,
#53562,#53563,#53564,#53565,#53566,#53567,#53568,#53569,#53570,#53571,#53572,
#53573,#53574,#53575,#53576,#53577,#53578,#53579,#53580,#53581,#53582,#53583,
#53584,#53585,#53586,#53587,#53588,#53589,#53590,#53591,#53592,#53593,#53594,
#53595,#53596,#53597,#53598,#53599,#53600,#53601,#53602,#53603,#53604,#53605,
#53606,#53607,#53608,#53609,#53610,#53611,#53612,#53613,#53614,#53615,#53616,
#53617,#53618,#53619,#53620,#53621,#53622,#53623,#53624,#53625,#53626,#53627,
#53628,#53629,#53630,#53631,#53632,#53633,#53634,#53635,#53636,#53637,#53638,
#53639,#53640,#53641,#53642,#53643,#53644,#53645,#53646,#53647,#53648,#53649,
#53650,#53651,#53652,#53653,#53654,#53655,#53656,#53657,#53658,#53659,#53660,
#53661,#53662,#53663,#53664,#53665,#53666,#53667,#53668,#53669,#53670,#53671,
#53672,#53673,#53674,#53675,#53676,#53677,#53678,#53679,#53680,#53681,#53682,
#53683,#53684,#53685,#53686,#53687,#53688,#53689,#53690,#53691,#53692,#53693,
#53694,#53695,#53696,#53697,#53698,#53699,#53700,#53701),(#53702,#53703,
#53704,#53705,#53706,#53707,#53708,#53709,#53710,#53711,#53712,#53713,#53714,
#53715,#53716,#53717,#53718,#53719,#53720,#53721,#53722,#53723,#53724,#53725,
#53726,#53727,#53728,#53729,#53730,#53731,#53732,#53733,#53734,#53735,#53736,
#53737,#53738,#53739,#53740,#53741,#53742,#53743,#53744,#53745,#53746,#53747,
#53748,#53749,#53750,#53751,#53752,#53753,#53754,#53755,#53756,#53757,#53758,
#53759,#53760,#53761,#53762,#53763,#53764,#53765,#53766,#53767,#53768,#53769,
#53770,#53771,#53772,#53773,#53774,#53775,#53776,#53777,#53778,#53779,#53780,
#53781,#53782,#53783,#53784,#53785,#53786,#53787,#53788,#53789,#53790,#53791,
#53792,#53793,#53794,#53795,#53796,#53797,#53798,#53799,#53800,#53801,#53802,
#53803,#53804,#53805,#53806,#53807,#53808,#53809,#53810,#53811,#53812,#53813,
#53814,#53815,#53816,#53817,#53818,#53819,#53820,#53821,#53822,#53823,#53824,
#53825,#53826,#53827,#53828,#53829,#53830,#53831,#53832,#53833,#53834,#53835,
#53836,#53837,#53838,#53839,#53840,#53841,#53842,#53843,#53844,#53845,#53846,
#53847,#53848,#53849,#53850,#53851,#53852,#53853,#53854,#53855,#53856,#53857,
#53858,#53859,#53860,#53861,#53862,#53863,#53864,#53865,#53866,#53867,#53868,
#53869,#53870,#53871,#53872,#53873,#53874,#53875,#53876,#53877,#53878,#53879,
#53880,#53881,#53882,#53883,#53884,#53885,#53886,#53887,#53888,#53889,#53890,
#53891,#53892,#53893,#53894,#53895,#53896,#53897,#53898,#53899,#53900,#53901,
#53902,#53903,#53904,#53905,#53906,#53907,#53908,#53909,#53910,#53911,#53912,
#53913,#53914,#53915,#53916,#53917,#53918,#53919,#53920,#53921,#53922,#53923,
#53924,#53925,#53926,#53927,#53928,#53929,#53930,#53931,#53932,#53933,#53934,
#53935,#53936,#53937,#53938,#53939,#53940,#53941,#53942,#53943,#53944,#53945,
#53946,#53947,#53948,#53949,#53950,#53951,#53952,#53953,#53954,#53955,#53956,
#53957,#53958,#53959,#53960,#53961,#53962,#53963,#53964,#53965,#53966,#53967,
#53968,#53969,#53970,#53971,#53972,#53973,#53974,#53975,#53976,#53977,#53978,
#53979,#53980,#53981,#53982,#53983,#53984,#53985,#53986,#53987,#53988,#53989,
#53990,#53991,#53992,#53993,#53994,#53995,#53996,#53997,#53998,#53999,#54000,
#54001,#54002,#54003,#54004,#54005,#54006,#54007,#54008,#54009,#54010,#54011,
#54012,#54013,#54014,#54015,#54016,#54017,#54018,#54019,#54020,#54021,#54022,
#54023,#54024,#54025,#54026,#54027,#54028,#54029,#54030,#54031,#54032,#54033,
#54034,#54035,#54036,#54037,#54038,#54039,#54040,#54041,#54042,#54043,#54044,
#54045,#54046,#54047,#54048,#54049,#54050,#54051,#54052,#54053,#54054,#54055,
#54056,#54057,#54058,#54059,#54060,#54061,#54062,#54063,#54064,#54065,#54066,
#54067,#54068,#54069,#54070),(#54071,#54072,#54073,#54074,#54075,#54076,
#54077,#54078,#54079,#54080,#54081,#54082,#54083,#54084,#54085,#54086,#54087,
#54088,#54089,#54090,#54091,#54092,#54093,#54094,#54095,#54096,#54097,#54098,
#54099,#54100,#54101,#54102,#54103,#54104,#54105,#54106,#54107,#54108,#54109,
#54110,#54111,#54112,#54113,#54114,#54115,#54116,#54117,#54118,#54119,#54120,
#54121,#54122,#54123,#54124,#54125,#54126,#54127,#54128,#54129,#54130,#54131,
#54132,#54133,#54134,#54135,#54136,#54137,#54138,#54139,#54140,#54141,#54142,
#54143,#54144,#54145,#54146,#54147,#54148,#54149,#54150,#54151,#54152,#54153,
#54154,#54155,#54156,#54157,#54158,#54159,#54160,#54161,#54162,#54163,#54164,
#54165,#54166,#54167,#54168,#54169,#54170,#54171,#54172,#54173,#54174,#54175,
#54176,#54177,#54178,#54179,#54180,#54181,#54182,#54183,#54184,#54185,#54186,
#54187,#54188,#54189,#54190,#54191,#54192,#54193,#54194,#54195,#54196,#54197,
#54198,#54199,#54200,#54201,#54202,#54203,#54204,#54205,#54206,#54207,#54208,
#54209,#54210,#54211,#54212,#54213,#54214,#54215,#54216,#54217,#54218,#54219,
#54220,#54221,#54222,#54223,#54224,#54225,#54226,#54227,#54228,#54229,#54230,
#54231,#54232,#54233,#54234,#54235,#54236,#54237,#54238,#54239,#54240,#54241,
#54242,#54243,#54244,#54245,#54246,#54247,#54248,#54249,#54250,#54251,#54252,
#54253,#54254,#54255,#54256,#54257,#54258,#54259,#54260,#54261,#54262,#54263,
#54264,#54265,#54266,#54267,#54268,#54269,#54270,#54271,#54272,#54273,#54274,
#54275,#54276,#54277,#54278,#54279,#54280,#54281,#54282,#54283,#54284,#54285,
#54286,#54287,#54288,#54289,#54290,#54291,#54292,#54293,#54294,#54295,#54296,
#54297,#54298,#54299,#54300,#54301,#54302,#54303,#54304,#54305,#54306,#54307,
#54308,#54309,#54310,#54311,#54312,#54313,#54314,#54315,#54316,#54317,#54318,
#54319,#54320,#54321,#54322,#54323,#54324,#54325,#54326,#54327,#54328,#54329,
#54330,#54331,#54332,#54333,#54334,#54335,#54336,#54337,#54338,#54339,#54340,
#54341,#54342,#54343,#54344,#54345,#54346,#54347,#54348,#54349,#54350,#54351,
#54352,#54353,#54354,#54355,#54356,#54357,#54358,#54359,#54360,#54361,#54362,
#54363,#54364,#54365,#54366,#54367,#54368,#54369,#54370,#54371,#54372,#54373,
#54374,#54375,#54376,#54377,#54378,#54379,#54380,#54381,#54382,#54383,#54384,
#54385,#54386,#54387,#54388,#54389,#54390,#54391,#54392,#54393,#54394,#54395,
#54396,#54397,#54398,#54399,#54400,#54401,#54402,#54403,#54404,#54405,#54406,
#54407,#54408,#54409,#54410,#54411,#54412,#54413,#54414,#54415,#54416,#54417,
#54418,#54419,#54420,#54421,#54422,#54423,#54424,#54425,#54426,#54427,#54428,
#54429,#54430,#54431,#54432,#54433,#54434,#54435,#54436,#54437,#54438,#54439)),
 .UNSPECIFIED.,.F.,.F.,.F.,(4,4),(4,1,1,1,1,1,1,1,1,1,1,1,1,1,1,1,1,1,1,
1,1,1,1,1,1,1,1,1,1,1,1,1,1,1,1,1,1,1,1,1,1,1,1,1,1,1,1,1,1,1,1,1,1,1,1,
1,1,1,1,1,1,1,1,1,1,1,1,1,1,1,1,1,1,1,1,1,1,1,1,1,1,1,1,1,1,1,1,1,1,1,1,
1,1,1,1,1,1,1,1,1,1,1,1,1,1,1,1,1,1,1,1,1,1,1,1,1,1,1,1,1,1,1,1,1,1,1,1,
1,1,1,1,1,1,1,1,1,1,1,1,1,1,1,1,1,1,1,1,1,1,1,1,1,1,1,1,1,1,1,1,1,1,1,1,
1,1,1,1,1,1,1,1,1,1,1,1,1,1,1,1,1,1,1,1,1,1,1,1,1,1,1,1,1,1,1,1,1,1,1,1,
1,1,1,1,1,1,1,1,1,1,1,1,1,1,1,1,1,1,1,1,1,1,1,1,1,1,1,1,1,1,1,1,1,1,1,1,
1,1,1,1,1,1,1,1,1,1,1,1,1,1,1,1,1,1,1,1,1,1,1,1,1,1,1,1,1,1,1,1,1,1,1,1,
1,1,1,1,1,1,1,1,1,1,1,1,1,1,1,1,1,1,1,1,1,1,1,1,1,1,1,1,1,1,1,1,1,1,1,1,
1,1,1,1,1,1,1,1,1,1,1,1,1,1,1,1,1,1,1,1,1,1,1,1,1,1,1,1,1,1,1,1,1,1,1,1,
1,1,1,1,1,1,1,1,1,1,1,1,1,1,1,1,1,1,1,1,1,1,1,4),(0.,0.132097741590586),
(11.6150328478184,12.1132112351144,12.6113896224105,13.1095680097066,13.6077463970026,
14.1059247842987,14.6041031715948,15.1022815588908,15.6004599461869,16.0986383334829,
16.596816720779,17.0949951080751,17.5931734953711,18.0913518826672,18.5895302699633,
19.0877086572593,19.5858870445554,20.0840654318515,20.5822438191475,21.0804222064436,
21.5786005937396,22.0767789810357,22.5749573683318,23.0731357556278,23.5713141429239,
24.06949253022,24.567670917516,25.0658493048121,25.5640276921081,26.0622060794042,
26.5603844667003,27.0585628539963,27.5567412412924,28.0549196285885,28.5530980158845,
29.0512764031806,29.5494547904767,30.0476331777727,30.5458115650688,31.0439899523648,
31.5421683396609,32.040346726957,32.538525114253,33.0367035015491,33.5348818888452,
34.0330602761412,34.5312386634373,35.0294170507333,35.5275954380294,36.0257738253255,
36.5239522126215,37.0221305999176,37.5203089872137,38.0184873745097,38.5166657618058,
39.0148441491019,39.5130225363979,40.011200923694,40.50937931099,41.0075576982861,
41.5057360855822,42.0039144728782,42.5020928601743,43.0002712474704,43.4984496347664,
43.9966280220625,44.4948064093585,44.9929847966546,45.4911631839507,45.9893415712467,
46.4875199585428,46.9856983458389,47.4838767331349,47.982055120431,48.480233507727,
48.9784118950231,49.4765902823192,49.9747686696152,50.4729470569113,50.9711254442074,
51.4693038315034,51.9674822187995,52.4656606060956,52.9638389933916,53.4620173806877,
53.9601957679837,54.4583741552798,54.9565525425759,55.4547309298719,55.952909317168,
56.4510877044641,56.9492660917601,57.4474444790562,57.9456228663523,58.4438012536483,
58.9419796409444,59.4401580282404,59.9383364155365,60.4365148028326,60.9346931901286,
61.4328715774247,61.9310499647208,62.4292283520168,62.9274067393129,63.425585126609,
63.923763513905,64.4219419012011,64.9201202884971,65.4182986757932,65.9164770630893,
66.4146554503853,66.9128338376814,67.4110122249775,67.9091906122735,68.4073689995696,
68.9055473868656,69.4037257741617,69.9019041614578,70.4000825487538,70.8982609360499,
71.396439323346,71.894617710642,72.3927960979381,72.8909744852342,73.3891528725302,
73.8873312598263,74.3855096471223,74.8836880344184,75.3818664217145,75.8800448090105,
76.3782231963066,76.8764015836027,77.3745799708987,77.8727583581948,78.3709367454909,
78.8691151327869,79.367293520083,79.865471907379,80.3636502946751,80.8618286819712,
81.3600070692672,81.8581854565633,82.3563638438594,82.8545422311554,83.3527206184515,
83.8508990057476,84.3490773930436,84.8472557803397,85.3454341676357,85.8436125549318,
86.3417909422279,86.8399693295239,87.33814771682,87.8363261041161,88.3345044914121,
88.8326828787082,89.3308612660042,89.8290396533003,90.3272180405964,90.8253964278924,
91.3235748151885,91.8217532024846,92.3199315897806,92.8181099770767,93.3162883643727,
93.8144667516688,94.3126451389649,94.8108235262609,95.309001913557,95.8071803008531,
96.3053586881491,96.8035370754452,97.3017154627413,97.7998938500373,98.2980722373334,
98.7962506246294,99.2944290119255,99.7926073992216,100.290785786518,100.788964173814,
101.28714256111,101.785320948406,102.283499335702,102.781677722998,103.279856110294,
103.77803449759,104.276212884886,104.774391272182,105.272569659478,105.770748046774,
106.26892643407,106.767104821366,107.265283208663,107.763461595959,108.261639983255,
108.759818370551,109.257996757847,109.756175145143,110.254353532439,110.752531919735,
111.250710307031,111.748888694327,112.247067081623,112.745245468919,113.243423856215,
113.741602243511,114.239780630807,114.737959018103,115.2361374054,115.734315792696,
116.232494179992,116.730672567288,117.228850954584,117.72702934188,118.225207729176,
118.723386116472,119.221564503768,119.719742891064,120.21792127836,120.716099665656,
121.214278052952,121.712456440248,122.210634827544,122.70881321484,123.206991602137,
123.705169989433,124.203348376729,124.701526764025,125.199705151321,125.697883538617,
126.196061925913,126.694240313209,127.192418700505,127.690597087801,128.188775475097,
128.686953862393,129.185132249689,129.683310636985,130.181489024281,130.679667411577,
131.177845798874,131.67602418617,132.174202573466,132.672380960762,133.170559348058,
133.668737735354,134.16691612265,134.665094509946,135.163272897242,135.661451284538,
136.159629671834,136.65780805913,137.155986446426,137.654164833722,138.152343221018,
138.650521608314,139.148699995611,139.646878382907,140.145056770203,140.643235157499,
141.141413544795,141.639591932091,142.137770319387,142.635948706683,143.134127093979,
143.632305481275,144.130483868571,144.628662255867,145.126840643163,145.625019030459,
146.123197417755,146.621375805052,147.119554192348,147.617732579644,148.11591096694,
148.614089354236,149.112267741532,149.610446128828,150.108624516124,150.60680290342,
151.104981290716,151.603159678012,152.101338065308,152.599516452604,153.0976948399,
153.595873227196,154.094051614492,154.592230001789,155.090408389085,155.588586776381,
156.086765163677,156.584943550973,157.083121938269,157.581300325565,158.079478712861,
158.577657100157,159.075835487453,159.574013874749,160.072192262045,160.570370649341,
161.068549036637,161.566727423933,162.064905811229,162.563084198526,163.061262585822,
163.559440973118,164.057619360414,164.55579774771,165.053976135006,165.552154522302,
166.050332909598,166.548511296894,167.04668968419,167.544868071486,168.043046458782,
168.541224846078,169.039403233374,169.53758162067,170.035760007966,170.533938395263,
171.032116782559,171.530295169855,172.028473557151,172.526651944447,173.024830331743,
173.523008719039,174.021187106335,174.519365493631,175.017543880927,175.515722268223,
176.013900655519,176.512079042815,177.010257430111,177.508435817407,178.006614204703,
178.504792592,179.002970979296,179.501149366592,179.999327753888,180.497506141184,
180.99568452848,181.493862915776,181.992041303072,182.490219690368,182.988398077664,
183.48657646496,183.984754852256,184.482933239552,184.981111626848,185.479290014144,
185.97746840144,186.475646788737,186.973825176033,187.472003563329,187.970181950625,
188.468360337921,188.966538725217,189.464717112513,189.962895499809,190.461073887105,
190.959252274401,191.457430661697,191.955609048993,192.453787436289,192.951965823585,
193.450144210881,193.948322598177),.UNSPECIFIED.);
#384=SHAPE_REPRESENTATION_RELATIONSHIP('SRR','None',#70825,#399);
#399=ADVANCED_BREP_SHAPE_REPRESENTATION('',(#474),#70749);
#414=STYLED_ITEM('',(#71054),#474);
#474=MANIFOLD_SOLID_BREP('Set screw',#26879);
#622=CYLINDRICAL_SURFACE('',#27548,0.7911);
#623=CYLINDRICAL_SURFACE('',#27550,0.7911);
#624=CYLINDRICAL_SURFACE('',#27551,0.7911);
#625=CYLINDRICAL_SURFACE('',#27552,0.7911);
#626=CYLINDRICAL_SURFACE('',#27553,0.7911);
#627=CYLINDRICAL_SURFACE('',#27554,0.7911);
#628=CYLINDRICAL_SURFACE('',#27555,0.7911);
#629=CYLINDRICAL_SURFACE('',#27556,0.7911);
#630=CYLINDRICAL_SURFACE('',#27557,0.7911);
#631=CYLINDRICAL_SURFACE('',#27558,0.7911);
#632=CYLINDRICAL_SURFACE('',#27559,0.7911);
#633=CYLINDRICAL_SURFACE('',#27560,0.7911);
#634=CYLINDRICAL_SURFACE('',#27561,0.7911);
#635=CYLINDRICAL_SURFACE('',#27562,0.7911);
#636=CYLINDRICAL_SURFACE('',#27563,0.7911);
#637=CYLINDRICAL_SURFACE('',#27564,0.7911);
#638=CYLINDRICAL_SURFACE('',#27565,0.7911);
#639=CYLINDRICAL_SURFACE('',#27566,0.7911);
#640=CYLINDRICAL_SURFACE('',#27567,0.7911);
#641=CYLINDRICAL_SURFACE('',#27568,0.7911);
#642=CYLINDRICAL_SURFACE('',#27569,0.7911);
#643=CYLINDRICAL_SURFACE('',#27570,0.7911);
#644=CYLINDRICAL_SURFACE('',#27571,0.7911);
#645=CYLINDRICAL_SURFACE('',#27572,0.7911);
#646=CYLINDRICAL_SURFACE('',#27573,0.7911);
#647=CYLINDRICAL_SURFACE('',#27574,0.7911);
#648=CYLINDRICAL_SURFACE('',#27575,0.7911);
#649=CYLINDRICAL_SURFACE('',#27576,0.7911);
#650=CYLINDRICAL_SURFACE('',#27577,0.7911);
#651=CYLINDRICAL_SURFACE('',#27578,0.6767);
#652=CYLINDRICAL_SURFACE('',#27580,0.6767);
#653=CYLINDRICAL_SURFACE('',#27582,0.6767);
#654=CYLINDRICAL_SURFACE('',#27583,0.6767);
#655=CYLINDRICAL_SURFACE('',#27584,0.6767);
#656=CYLINDRICAL_SURFACE('',#27585,0.6767);
#657=CYLINDRICAL_SURFACE('',#27586,0.6767);
#658=CYLINDRICAL_SURFACE('',#27587,0.6767);
#659=CYLINDRICAL_SURFACE('',#27588,0.6767);
#660=CYLINDRICAL_SURFACE('',#27589,0.6767);
#661=CYLINDRICAL_SURFACE('',#27590,0.6767);
#662=CYLINDRICAL_SURFACE('',#27591,0.6767);
#663=CYLINDRICAL_SURFACE('',#27592,0.6767);
#664=CYLINDRICAL_SURFACE('',#27593,0.6767);
#665=CYLINDRICAL_SURFACE('',#27594,0.6767);
#666=CYLINDRICAL_SURFACE('',#27595,0.6767);
#667=CYLINDRICAL_SURFACE('',#27596,0.6767);
#668=CYLINDRICAL_SURFACE('',#27597,0.6767);
#669=CYLINDRICAL_SURFACE('',#27598,0.6767);
#670=CYLINDRICAL_SURFACE('',#27599,0.6767);
#671=CYLINDRICAL_SURFACE('',#27600,0.6767);
#672=CYLINDRICAL_SURFACE('',#27601,0.6767);
#673=CYLINDRICAL_SURFACE('',#27602,0.6767);
#674=CYLINDRICAL_SURFACE('',#27603,0.6767);
#675=CYLINDRICAL_SURFACE('',#27604,0.6767);
#676=CYLINDRICAL_SURFACE('',#27605,0.6767);
#677=CYLINDRICAL_SURFACE('',#27606,0.6767);
#678=CYLINDRICAL_SURFACE('',#27607,0.6767);
#679=CYLINDRICAL_SURFACE('',#27608,0.6767);
#680=CYLINDRICAL_SURFACE('',#27616,0.6767);
#681=CYLINDRICAL_SURFACE('',#27664,0.7911);
#864=FACE_BOUND('',#4519,.T.);
#1170=B_SPLINE_CURVE_WITH_KNOTS('',3,(#47594,#47595,#47596,#47597,#47598,
#47599,#47600,#47601,#47602,#47603,#47604,#47605,#47606,#47607,#47608,#47609),
 .UNSPECIFIED.,.F.,.F.,(4,3,3,3,3,4),(-4.09293042013069,-3.98542709836851,
-3.48724871107244,-2.98907032377638,-2.49089193648032,-2.07498647268394),
 .UNSPECIFIED.);
#1171=B_SPLINE_CURVE_WITH_KNOTS('',3,(#47612,#47613,#47614,#47615,#47616,
#47617,#47618,#47619,#47620,#47621),.UNSPECIFIED.,.F.,.F.,(4,3,3,4),(0.,
0.498178387296066,0.996356774592132,1.1236487061432),.UNSPECIFIED.);
#1172=B_SPLINE_CURVE_WITH_KNOTS('',3,(#47626,#47627,#47628,#47629,#47630,
#47631,#47632,#47633,#47634,#47635,#47636,#47637,#47638,#47639,#47640,#47641,
#47642,#47643,#47644,#47645,#47646,#47647,#47648,#47649,#47650,#47651,#47652,
#47653,#47654,#47655,#47656,#47657,#47658,#47659,#47660,#47661,#47662,#47663,
#47664,#47665),.UNSPECIFIED.,.F.,.F.,(4,3,3,3,3,3,3,3,3,3,3,3,3,4),(-10.3761157273103,
-9.96356774592127,-9.4653893586252,-8.96721097132914,-8.46903258403308,
-7.97085419673701,-7.47267580944095,-6.97449742214489,-6.47631903484883,
-5.97814064755276,-5.4799622602567,-4.98178387296063,-4.48360548566457,
-4.09293042013069),.UNSPECIFIED.);
#1173=B_SPLINE_CURVE_WITH_KNOTS('',3,(#47666,#47667,#47668,#47669,#47670,
#47671,#47672,#47673,#47674,#47675,#47676,#47677,#47678,#47679,#47680,#47681,
#47682,#47683,#47684,#47685,#47686,#47687,#47688,#47689,#47690,#47691,#47692,
#47693,#47694,#47695,#47696,#47697,#47698,#47699,#47700,#47701,#47702,#47703,
#47704,#47705),.UNSPECIFIED.,.F.,.F.,(4,3,3,3,3,3,3,3,3,3,3,3,3,4),(1.1236487061432,
1.4945351618882,1.99271354918426,2.49089193648032,2.98907032377638,3.48724871107245,
3.98542709836851,4.48360548566457,4.98178387296063,5.4799622602567,5.97814064755276,
6.47631903484882,6.97449742214488,7.40683401332279),.UNSPECIFIED.);
#1174=B_SPLINE_CURVE_WITH_KNOTS('',3,(#47710,#47711,#47712,#47713,#47714,
#47715,#47716,#47717,#47718,#47719,#47720,#47721,#47722,#47723,#47724,#47725,
#47726,#47727,#47728,#47729,#47730,#47731,#47732,#47733,#47734,#47735,#47736,
#47737,#47738,#47739,#47740,#47741,#47742,#47743,#47744,#47745,#47746,#47747,
#47748,#47749,#47750,#47751,#47752),.UNSPECIFIED.,.F.,.F.,(4,3,3,3,3,3,
3,3,3,3,3,3,3,3,4),(-16.6593010344898,-16.4398867807701,-15.941708393474,
-15.443530006178,-14.9453516188819,-14.4471732315858,-13.9489948442898,
-13.4508164569937,-12.9526380696976,-12.4544596824016,-11.9562812951055,
-11.4581029078095,-10.9599245205134,-10.4617461332173,-10.3761157273103),
 .UNSPECIFIED.);
#1175=B_SPLINE_CURVE_WITH_KNOTS('',3,(#47753,#47754,#47755,#47756,#47757,
#47758,#47759,#47760,#47761,#47762,#47763,#47764,#47765,#47766,#47767,#47768,
#47769,#47770,#47771,#47772,#47773,#47774,#47775,#47776,#47777,#47778,#47779,
#47780,#47781,#47782,#47783,#47784,#47785,#47786,#47787,#47788,#47789,#47790,
#47791,#47792,#47793,#47794,#47795),.UNSPECIFIED.,.F.,.F.,(4,3,3,3,3,3,
3,3,3,3,3,3,3,3,4),(7.40683401332279,7.47267580944095,7.97085419673701,
8.46903258403307,8.96721097132914,9.4653893586252,9.96356774592126,10.4617461332173,
10.9599245205134,11.4581029078095,11.9562812951055,12.4544596824016,12.9526380696976,
13.4508164569937,13.6900193205024),.UNSPECIFIED.);
#1176=B_SPLINE_CURVE_WITH_KNOTS('',3,(#47800,#47801,#47802,#47803,#47804,
#47805,#47806,#47807,#47808,#47809,#47810,#47811,#47812,#47813,#47814,#47815,
#47816,#47817,#47818,#47819,#47820,#47821,#47822,#47823,#47824,#47825,#47826,
#47827,#47828,#47829,#47830,#47831,#47832,#47833,#47834,#47835,#47836,#47837,
#47838,#47839,#47840,#47841,#47842),.UNSPECIFIED.,.F.,.F.,(4,3,3,3,3,3,
3,3,3,3,3,3,3,3,4),(-22.9424863416694,-22.9162058156189,-22.4180274283228,
-21.9198490410268,-21.4216706537307,-20.9234922664347,-20.4253138791386,
-19.9271354918425,-19.4289571045465,-18.9307787172504,-18.4326003299543,
-17.9344219426583,-17.4362435553622,-16.9380651680661,-16.6593010344898),
 .UNSPECIFIED.);
#1177=B_SPLINE_CURVE_WITH_KNOTS('',3,(#47843,#47844,#47845,#47846,#47847,
#47848,#47849,#47850,#47851,#47852,#47853,#47854,#47855,#47856,#47857,#47858,
#47859,#47860,#47861,#47862,#47863,#47864,#47865,#47866,#47867,#47868,#47869,
#47870,#47871,#47872,#47873,#47874,#47875,#47876,#47877,#47878,#47879,#47880,
#47881,#47882,#47883,#47884,#47885),.UNSPECIFIED.,.F.,.F.,(4,3,3,3,3,3,
3,3,3,3,3,3,3,3,4),(13.6900193205024,13.9489948442898,14.4471732315858,
14.9453516188819,15.443530006178,15.941708393474,16.4398867807701,16.9380651680661,
17.4362435553622,17.9344219426583,18.4326003299543,18.9307787172504,19.4289571045465,
19.9271354918425,19.9732046276819),.UNSPECIFIED.);
#1178=B_SPLINE_CURVE_WITH_KNOTS('',3,(#47890,#47891,#47892,#47893,#47894,
#47895,#47896,#47897,#47898,#47899,#47900,#47901,#47902,#47903,#47904,#47905,
#47906,#47907,#47908,#47909,#47910,#47911,#47912,#47913,#47914,#47915,#47916,
#47917,#47918,#47919,#47920,#47921,#47922,#47923,#47924,#47925,#47926,#47927,
#47928,#47929),.UNSPECIFIED.,.F.,.F.,(4,3,3,3,3,3,3,3,3,3,3,3,3,4),(-29.225671648849,
-28.8943464631717,-28.3961680758756,-27.8979896885795,-27.3998113012835,
-26.9016329139874,-26.4034545266914,-25.9052761393953,-25.4070977520992,
-24.9089193648032,-24.4107409775071,-23.912562590211,-23.414384202915,-22.9424863416694),
 .UNSPECIFIED.);
#1179=B_SPLINE_CURVE_WITH_KNOTS('',3,(#47930,#47931,#47932,#47933,#47934,
#47935,#47936,#47937,#47938,#47939,#47940,#47941,#47942,#47943,#47944,#47945,
#47946,#47947,#47948,#47949,#47950,#47951,#47952,#47953,#47954,#47955,#47956,
#47957,#47958,#47959,#47960,#47961,#47962,#47963,#47964,#47965,#47966,#47967,
#47968,#47969),.UNSPECIFIED.,.F.,.F.,(4,3,3,3,3,3,3,3,3,3,3,3,3,4),(19.9732046276819,
20.4253138791386,20.9234922664346,21.4216706537307,21.9198490410268,22.4180274283228,
22.9162058156189,23.414384202915,23.912562590211,24.4107409775071,24.9089193648032,
25.4070977520992,25.9052761393953,26.2563899348615),.UNSPECIFIED.);
#1180=B_SPLINE_CURVE_WITH_KNOTS('',3,(#47974,#47975,#47976,#47977,#47978,
#47979,#47980,#47981,#47982,#47983,#47984,#47985,#47986,#47987,#47988,#47989,
#47990,#47991,#47992,#47993,#47994,#47995,#47996,#47997,#47998,#47999,#48000,
#48001,#48002,#48003,#48004,#48005,#48006,#48007,#48008,#48009,#48010,#48011,
#48012,#48013,#48014,#48015,#48016),.UNSPECIFIED.,.F.,.F.,(4,3,3,3,3,3,
3,3,3,3,3,3,3,3,4),(-35.5088569560286,-35.3706654980205,-34.8724871107244,
-34.3743087234284,-33.8761303361323,-33.3779519488362,-32.8797735615402,
-32.3815951742441,-31.883416786948,-31.385238399652,-30.8870600123559,-30.3888816250599,
-29.8907032377638,-29.3925248504677,-29.225671648849),.UNSPECIFIED.);
#1181=B_SPLINE_CURVE_WITH_KNOTS('',3,(#48017,#48018,#48019,#48020,#48021,
#48022,#48023,#48024,#48025,#48026,#48027,#48028,#48029,#48030,#48031,#48032,
#48033,#48034,#48035,#48036,#48037,#48038,#48039,#48040,#48041,#48042,#48043,
#48044,#48045,#48046,#48047,#48048,#48049,#48050,#48051,#48052,#48053,#48054,
#48055,#48056,#48057,#48058,#48059),.UNSPECIFIED.,.F.,.F.,(4,3,3,3,3,3,
3,3,3,3,3,3,3,3,4),(26.2563899348615,26.4034545266914,26.9016329139874,
27.3998113012835,27.8979896885795,28.3961680758756,28.8943464631717,29.3925248504677,
29.8907032377638,30.3888816250599,30.8870600123559,31.385238399652,31.883416786948,
32.3815951742441,32.5395752420411),.UNSPECIFIED.);
#1182=B_SPLINE_CURVE_WITH_KNOTS('',3,(#48064,#48065,#48066,#48067,#48068,
#48069,#48070,#48071,#48072,#48073,#48074,#48075,#48076,#48077,#48078,#48079,
#48080,#48081,#48082,#48083,#48084,#48085,#48086,#48087,#48088,#48089,#48090,
#48091,#48092,#48093,#48094,#48095,#48096,#48097,#48098,#48099,#48100,#48101,
#48102,#48103),.UNSPECIFIED.,.F.,.F.,(4,3,3,3,3,3,3,3,3,3,3,3,3,4),(-41.7920422632082,
-41.3488061455732,-40.8506277582772,-40.3524493709811,-39.8542709836851,
-39.356092596389,-38.8579142090929,-38.3597358217969,-37.8615574345008,
-37.3633790472047,-36.8652006599087,-36.3670222726126,-35.8688438853166,
-35.5088569560286),.UNSPECIFIED.);
#1183=B_SPLINE_CURVE_WITH_KNOTS('',3,(#48104,#48105,#48106,#48107,#48108,
#48109,#48110,#48111,#48112,#48113,#48114,#48115,#48116,#48117,#48118,#48119,
#48120,#48121,#48122,#48123,#48124,#48125,#48126,#48127,#48128,#48129,#48130,
#48131,#48132,#48133,#48134,#48135,#48136,#48137,#48138,#48139,#48140,#48141,
#48142,#48143),.UNSPECIFIED.,.F.,.F.,(4,3,3,3,3,3,3,3,3,3,3,3,3,4),(32.5395752420411,
32.8797735615402,33.3779519488362,33.8761303361323,34.3743087234284,34.8724871107244,
35.3706654980205,35.8688438853165,36.3670222726126,36.8652006599087,37.3633790472047,
37.8615574345008,38.3597358217969,38.8227605492207),.UNSPECIFIED.);
#1184=B_SPLINE_CURVE_WITH_KNOTS('',3,(#48148,#48149,#48150,#48151,#48152,
#48153,#48154,#48155,#48156,#48157,#48158,#48159,#48160,#48161,#48162,#48163,
#48164,#48165,#48166,#48167,#48168,#48169,#48170,#48171,#48172,#48173,#48174,
#48175,#48176,#48177,#48178,#48179,#48180,#48181,#48182,#48183,#48184,#48185,
#48186,#48187,#48188,#48189,#48190),.UNSPECIFIED.,.F.,.F.,(4,3,3,3,3,3,
3,3,3,3,3,3,3,3,4),(-48.0752275703878,-47.8251251804221,-47.326946793126,
-46.8287684058299,-46.3305900185339,-45.8324116312378,-45.3342332439418,
-44.8360548566457,-44.3378764693496,-43.8396980820536,-43.3415196947575,
-42.8433413074614,-42.3451629201654,-41.8469845328693,-41.7920422632082),
 .UNSPECIFIED.);
#1185=B_SPLINE_CURVE_WITH_KNOTS('',3,(#48191,#48192,#48193,#48194,#48195,
#48196,#48197,#48198,#48199,#48200,#48201,#48202,#48203,#48204,#48205,#48206,
#48207,#48208,#48209,#48210,#48211,#48212,#48213,#48214,#48215,#48216,#48217,
#48218,#48219,#48220,#48221,#48222,#48223,#48224,#48225,#48226,#48227,#48228,
#48229,#48230,#48231,#48232,#48233),.UNSPECIFIED.,.F.,.F.,(4,3,3,3,3,3,
3,3,3,3,3,3,3,3,4),(38.8227605492207,38.8579142090929,39.356092596389,39.8542709836851,
40.3524493709811,40.8506277582772,41.3488061455732,41.8469845328693,42.3451629201654,
42.8433413074614,43.3415196947575,43.8396980820536,44.3378764693496,44.8360548566457,
45.1059458564003),.UNSPECIFIED.);
#1186=B_SPLINE_CURVE_WITH_KNOTS('',3,(#48238,#48239,#48240,#48241,#48242,
#48243,#48244,#48245,#48246,#48247,#48248,#48249,#48250,#48251,#48252,#48253,
#48254,#48255,#48256,#48257,#48258,#48259,#48260,#48261,#48262,#48263,#48264,
#48265,#48266,#48267,#48268,#48269,#48270,#48271,#48272,#48273,#48274,#48275,
#48276,#48277,#48278,#48279,#48280),.UNSPECIFIED.,.F.,.F.,(4,3,3,3,3,3,
3,3,3,3,3,3,3,3,4),(-54.3584128775674,-54.3014442152709,-53.8032658279748,
-53.3050874406788,-52.8069090533827,-52.3087306660866,-51.8105522787906,
-51.3123738914945,-50.8141955041984,-50.3160171169024,-49.8178387296063,
-49.3196603423103,-48.8214819550142,-48.3233035677181,-48.0752275703878),
 .UNSPECIFIED.);
#1187=B_SPLINE_CURVE_WITH_KNOTS('',3,(#48281,#48282,#48283,#48284,#48285,
#48286,#48287,#48288,#48289,#48290,#48291,#48292,#48293,#48294,#48295,#48296,
#48297,#48298,#48299,#48300,#48301,#48302,#48303,#48304,#48305,#48306,#48307,
#48308,#48309,#48310,#48311,#48312,#48313,#48314,#48315,#48316,#48317,#48318,
#48319,#48320,#48321,#48322,#48323),.UNSPECIFIED.,.F.,.F.,(4,3,3,3,3,3,
3,3,3,3,3,3,3,3,4),(45.1059458564003,45.3342332439418,45.8324116312378,
46.3305900185339,46.8287684058299,47.326946793126,47.8251251804221,48.3233035677181,
48.8214819550142,49.3196603423102,49.8178387296063,50.3160171169024,50.8141955041984,
51.3123738914945,51.3891311635799),.UNSPECIFIED.);
#1188=B_SPLINE_CURVE_WITH_KNOTS('',3,(#48328,#48329,#48330,#48331,#48332,
#48333,#48334,#48335,#48336,#48337,#48338,#48339,#48340,#48341,#48342,#48343,
#48344,#48345,#48346,#48347,#48348,#48349,#48350,#48351,#48352,#48353,#48354,
#48355,#48356,#48357,#48358,#48359,#48360,#48361,#48362,#48363,#48364,#48365,
#48366,#48367),.UNSPECIFIED.,.F.,.F.,(4,3,3,3,3,3,3,3,3,3,3,3,3,4),(-60.641598184747,
-60.2795848628236,-59.7814064755276,-59.2832280882315,-58.7850497009355,
-58.2868713136394,-57.7886929263433,-57.2905145390473,-56.7923361517512,
-56.2941577644551,-55.7959793771591,-55.297800989863,-54.7996226025669,
-54.3584128775674),.UNSPECIFIED.);
#1189=B_SPLINE_CURVE_WITH_KNOTS('',3,(#48368,#48369,#48370,#48371,#48372,
#48373,#48374,#48375,#48376,#48377,#48378,#48379,#48380,#48381,#48382,#48383,
#48384,#48385,#48386,#48387,#48388,#48389,#48390,#48391,#48392,#48393,#48394,
#48395,#48396,#48397,#48398,#48399,#48400,#48401,#48402,#48403,#48404,#48405,
#48406,#48407),.UNSPECIFIED.,.F.,.F.,(4,3,3,3,3,3,3,3,3,3,3,3,3,4),(51.3891311635799,
51.8105522787905,52.3087306660866,52.8069090533827,53.3050874406787,53.8032658279748,
54.3014442152709,54.7996226025669,55.297800989863,55.7959793771591,56.2941577644551,
56.7923361517512,57.2905145390473,57.6723164707595),.UNSPECIFIED.);
#1190=B_SPLINE_CURVE_WITH_KNOTS('',3,(#48412,#48413,#48414,#48415,#48416,
#48417,#48418,#48419,#48420,#48421,#48422,#48423,#48424,#48425,#48426,#48427,
#48428,#48429,#48430,#48431,#48432,#48433,#48434,#48435,#48436,#48437,#48438,
#48439,#48440,#48441,#48442,#48443,#48444,#48445,#48446,#48447,#48448,#48449,
#48450,#48451,#48452,#48453,#48454),.UNSPECIFIED.,.F.,.F.,(4,3,3,3,3,3,
3,3,3,3,3,3,3,3,4),(-66.9247834919266,-66.7559038976725,-66.2577255103764,
-65.7595471230803,-65.2613687357843,-64.7631903484882,-64.2650119611921,
-63.7668335738961,-63.2686551866,-62.770476799304,-62.2722984120079,-61.7741200247118,
-61.2759416374158,-60.7777632501197,-60.641598184747),.UNSPECIFIED.);
#1191=B_SPLINE_CURVE_WITH_KNOTS('',3,(#48455,#48456,#48457,#48458,#48459,
#48460,#48461,#48462,#48463,#48464,#48465,#48466,#48467,#48468,#48469,#48470,
#48471,#48472,#48473,#48474,#48475,#48476,#48477,#48478,#48479,#48480,#48481,
#48482,#48483,#48484,#48485,#48486,#48487,#48488,#48489,#48490,#48491,#48492,
#48493,#48494,#48495,#48496,#48497),.UNSPECIFIED.,.F.,.F.,(4,3,3,3,3,3,
3,3,3,3,3,3,3,3,4),(57.6723164707595,57.7886929263433,58.2868713136394,
58.7850497009355,59.2832280882315,59.7814064755276,60.2795848628236,60.7777632501197,
61.2759416374158,61.7741200247118,62.2722984120079,62.770476799304,63.2686551866,
63.7668335738961,63.9555017779391),.UNSPECIFIED.);
#1192=B_SPLINE_CURVE_WITH_KNOTS('',3,(#48502,#48503,#48504,#48505,#48506,
#48507,#48508,#48509,#48510,#48511,#48512,#48513,#48514,#48515,#48516,#48517,
#48518,#48519,#48520,#48521,#48522,#48523,#48524,#48525,#48526,#48527,#48528,
#48529,#48530,#48531,#48532,#48533,#48534,#48535,#48536,#48537,#48538,#48539,
#48540,#48541),.UNSPECIFIED.,.F.,.F.,(4,3,3,3,3,3,3,3,3,3,3,3,3,4),(-73.2079687991062,
-72.7340445452252,-72.2358661579292,-71.7376877706331,-71.239509383337,
-70.741330996041,-70.2431526087449,-69.7449742214488,-69.2467958341528,
-68.7486174468567,-68.2504390595606,-67.7522606722646,-67.2540822849685,
-66.9247834919266),.UNSPECIFIED.);
#1193=B_SPLINE_CURVE_WITH_KNOTS('',3,(#48542,#48543,#48544,#48545,#48546,
#48547,#48548,#48549,#48550,#48551,#48552,#48553,#48554,#48555,#48556,#48557,
#48558,#48559,#48560,#48561,#48562,#48563,#48564,#48565,#48566,#48567,#48568,
#48569,#48570,#48571,#48572,#48573,#48574,#48575,#48576,#48577,#48578,#48579,
#48580,#48581),.UNSPECIFIED.,.F.,.F.,(4,3,3,3,3,3,3,3,3,3,3,3,3,4),(63.9555017779391,
64.2650119611922,64.7631903484882,65.2613687357843,65.7595471230804,66.2577255103764,
66.7559038976725,67.2540822849685,67.7522606722646,68.2504390595607,68.7486174468567,
69.2467958341528,69.7449742214488,70.2386870851187),.UNSPECIFIED.);
#1194=B_SPLINE_CURVE_WITH_KNOTS('',3,(#48586,#48587,#48588,#48589,#48590,
#48591,#48592,#48593,#48594,#48595,#48596,#48597,#48598,#48599,#48600,#48601,
#48602,#48603,#48604,#48605,#48606,#48607,#48608,#48609,#48610,#48611,#48612,
#48613,#48614,#48615,#48616,#48617,#48618,#48619,#48620,#48621,#48622,#48623,
#48624,#48625,#48626,#48627,#48628),.UNSPECIFIED.,.F.,.F.,(4,3,3,3,3,3,
3,3,3,3,3,3,3,3,4),(-79.4911541062858,-79.2103635800741,-78.712185192778,
-78.2140068054819,-77.7158284181859,-77.2176500308898,-76.7194716435937,
-76.2212932562977,-75.7231148690016,-75.2249364817055,-74.7267580944095,
-74.2285797071134,-73.7304013198173,-73.2322229325213,-73.2079687991062),
 .UNSPECIFIED.);
#1195=B_SPLINE_CURVE_WITH_KNOTS('',3,(#48629,#48630,#48631,#48632,#48633,
#48634,#48635,#48636,#48637,#48638,#48639,#48640,#48641,#48642,#48643,#48644,
#48645,#48646,#48647,#48648,#48649,#48650,#48651,#48652,#48653,#48654,#48655,
#48656,#48657,#48658,#48659,#48660,#48661,#48662,#48663,#48664,#48665,#48666,
#48667,#48668,#48669,#48670,#48671),.UNSPECIFIED.,.F.,.F.,(4,3,3,3,3,3,
3,3,3,3,3,3,3,3,4),(70.2386870851187,70.2431526087449,70.741330996041,71.239509383337,
71.7376877706331,72.2358661579292,72.7340445452252,73.2322229325213,73.7304013198174,
74.2285797071134,74.7267580944095,75.2249364817056,75.7231148690016,76.2212932562977,
76.5218723922983),.UNSPECIFIED.);
#1196=B_SPLINE_CURVE_WITH_KNOTS('',3,(#48676,#48677,#48678,#48679,#48680,
#48681,#48682,#48683,#48684,#48685,#48686,#48687,#48688,#48689,#48690,#48691,
#48692,#48693,#48694,#48695,#48696,#48697,#48698,#48699,#48700,#48701,#48702,
#48703,#48704,#48705,#48706,#48707,#48708,#48709,#48710,#48711,#48712,#48713,
#48714,#48715,#48716,#48717,#48718),.UNSPECIFIED.,.F.,.F.,(4,3,3,3,3,3,
3,3,3,3,3,3,3,3,4),(-85.7743394134654,-85.6866826149229,-85.1885042276268,
-84.6903258403307,-84.1921474530347,-83.6939690657386,-83.1957906784425,
-82.6976122911465,-82.1994339038504,-81.7012555165544,-81.2030771292583,
-80.7048987419623,-80.2067203546662,-79.7085419673701,-79.4911541062858),
 .UNSPECIFIED.);
#1197=B_SPLINE_CURVE_WITH_KNOTS('',3,(#48719,#48720,#48721,#48722,#48723,
#48724,#48725,#48726,#48727,#48728,#48729,#48730,#48731,#48732,#48733,#48734,
#48735,#48736,#48737,#48738,#48739,#48740,#48741,#48742,#48743,#48744,#48745,
#48746,#48747,#48748,#48749,#48750,#48751,#48752,#48753,#48754,#48755,#48756,
#48757,#48758,#48759,#48760,#48761),.UNSPECIFIED.,.F.,.F.,(4,3,3,3,3,3,
3,3,3,3,3,3,3,3,4),(76.5218723922983,76.7194716435937,77.2176500308898,
77.7158284181859,78.2140068054819,78.712185192778,79.210363580074,79.7085419673701,
80.2067203546662,80.7048987419622,81.2030771292583,81.7012555165544,82.1994339038504,
82.6976122911465,82.8050576994779),.UNSPECIFIED.);
#1198=B_SPLINE_CURVE_WITH_KNOTS('',3,(#48766,#48767,#48768,#48769,#48770,
#48771,#48772,#48773,#48774,#48775,#48776,#48777,#48778,#48779,#48780,#48781,
#48782,#48783,#48784,#48785,#48786,#48787,#48788,#48789,#48790,#48791,#48792,
#48793,#48794,#48795,#48796,#48797,#48798,#48799,#48800,#48801,#48802,#48803,
#48804,#48805),.UNSPECIFIED.,.F.,.F.,(4,3,3,3,3,3,3,3,3,3,3,3,3,4),(-92.0575247206449,
-91.6648232624756,-91.1666448751796,-90.6684664878835,-90.1702881005874,
-89.6721097132914,-89.1739313259953,-88.6757529386992,-88.1775745514032,
-87.6793961641071,-87.1812177768111,-86.683039389515,-86.1848610022189,
-85.7743394134654),.UNSPECIFIED.);
#1199=B_SPLINE_CURVE_WITH_KNOTS('',3,(#48806,#48807,#48808,#48809,#48810,
#48811,#48812,#48813,#48814,#48815,#48816,#48817,#48818,#48819,#48820,#48821,
#48822,#48823,#48824,#48825,#48826,#48827,#48828,#48829,#48830,#48831,#48832,
#48833,#48834,#48835,#48836,#48837,#48838,#48839,#48840,#48841,#48842,#48843,
#48844,#48845),.UNSPECIFIED.,.F.,.F.,(4,3,3,3,3,3,3,3,3,3,3,3,3,4),(82.8050576994779,
83.1957906784425,83.6939690657386,84.1921474530347,84.6903258403308,85.1885042276268,
85.6866826149229,86.1848610022189,86.683039389515,87.1812177768111,87.6793961641071,
88.1775745514032,88.6757529386992,89.0882430066575),.UNSPECIFIED.);
#1200=B_SPLINE_CURVE_WITH_KNOTS('',3,(#48850,#48851,#48852,#48853,#48854,
#48855,#48856,#48857,#48858,#48859,#48860,#48861,#48862,#48863,#48864,#48865,
#48866,#48867,#48868,#48869,#48870,#48871,#48872,#48873,#48874,#48875,#48876,
#48877,#48878,#48879,#48880,#48881,#48882,#48883,#48884,#48885,#48886,#48887,
#48888,#48889,#48890,#48891,#48892),.UNSPECIFIED.,.F.,.F.,(4,3,3,3,3,3,
3,3,3,3,3,3,3,3,4),(-98.3407100278245,-98.1411422973244,-97.6429639100284,
-97.1447855227323,-96.6466071354363,-96.1484287481402,-95.6502503608441,
-95.1520719735481,-94.653893586252,-94.1557151989559,-93.6575368116599,
-93.1593584243638,-92.6611800370678,-92.1630016497717,-92.0575247206449),
 .UNSPECIFIED.);
#1201=B_SPLINE_CURVE_WITH_KNOTS('',3,(#48893,#48894,#48895,#48896,#48897,
#48898,#48899,#48900,#48901,#48902,#48903,#48904,#48905,#48906,#48907,#48908,
#48909,#48910,#48911,#48912,#48913,#48914,#48915,#48916,#48917,#48918,#48919,
#48920,#48921,#48922,#48923,#48924,#48925,#48926,#48927,#48928,#48929,#48930,
#48931,#48932,#48933,#48934,#48935),.UNSPECIFIED.,.F.,.F.,(4,3,3,3,3,3,
3,3,3,3,3,3,3,3,4),(89.0882430066575,89.1739313259953,89.6721097132914,
90.1702881005874,90.6684664878835,91.1666448751796,91.6648232624756,92.1630016497717,
92.6611800370678,93.1593584243638,93.6575368116599,94.1557151989559,94.653893586252,
95.1520719735481,95.371428313837),.UNSPECIFIED.);
#1202=B_SPLINE_CURVE_WITH_KNOTS('',3,(#48940,#48941,#48942,#48943,#48944,
#48945,#48946,#48947,#48948,#48949,#48950,#48951,#48952,#48953,#48954,#48955,
#48956,#48957,#48958,#48959,#48960,#48961,#48962,#48963,#48964,#48965,#48966,
#48967,#48968,#48969,#48970,#48971,#48972,#48973,#48974,#48975,#48976,#48977,
#48978,#48979,#48980,#48981,#48982),.UNSPECIFIED.,.F.,.F.,(4,3,3,3,3,3,
3,3,3,3,3,3,3,3,4),(-104.623895335004,-104.617461332173,-104.119282944877,
-103.621104557581,-103.122926170285,-102.624747782989,-102.126569395693,
-101.628391008397,-101.130212621101,-100.632034233805,-100.133855846509,
-99.6356774592126,-99.1374990719166,-98.6393206846205,-98.3407100278245),
 .UNSPECIFIED.);
#1203=B_SPLINE_CURVE_WITH_KNOTS('',3,(#48983,#48984,#48985,#48986,#48987,
#48988,#48989,#48990,#48991,#48992,#48993,#48994,#48995,#48996,#48997,#48998,
#48999,#49000,#49001,#49002,#49003,#49004,#49005,#49006,#49007,#49008,#49009,
#49010,#49011,#49012,#49013,#49014,#49015,#49016,#49017,#49018,#49019,#49020,
#49021,#49022,#49023,#49024,#49025),.UNSPECIFIED.,.F.,.F.,(4,3,3,3,3,3,
3,3,3,3,3,3,3,3,4),(95.371428313837,95.6502503608441,96.1484287481402,96.6466071354362,
97.1447855227323,97.6429639100284,98.1411422973244,98.6393206846205,99.1374990719166,
99.6356774592126,100.133855846509,100.632034233805,101.130212621101,101.628391008397,
101.654613621017),.UNSPECIFIED.);
#1204=B_SPLINE_CURVE_WITH_KNOTS('',3,(#49030,#49031,#49032,#49033,#49034,
#49035,#49036,#49037,#49038,#49039,#49040,#49041,#49042,#49043,#49044,#49045,
#49046,#49047,#49048,#49049,#49050,#49051,#49052,#49053,#49054,#49055,#49056,
#49057,#49058,#49059,#49060,#49061,#49062,#49063,#49064,#49065,#49066,#49067,
#49068,#49069),.UNSPECIFIED.,.F.,.F.,(4,3,3,3,3,3,3,3,3,3,3,3,3,4),(-110.907080642184,
-110.595601979726,-110.09742359243,-109.599245205134,-109.101066817838,
-108.602888430542,-108.104710043246,-107.60653165595,-107.108353268654,
-106.610174881358,-106.111996494061,-105.613818106765,-105.115639719469,
-104.623895335004),.UNSPECIFIED.);
#1205=B_SPLINE_CURVE_WITH_KNOTS('',3,(#49070,#49071,#49072,#49073,#49074,
#49075,#49076,#49077,#49078,#49079,#49080,#49081,#49082,#49083,#49084,#49085,
#49086,#49087,#49088,#49089,#49090,#49091,#49092,#49093,#49094,#49095,#49096,
#49097,#49098,#49099,#49100,#49101,#49102,#49103,#49104,#49105,#49106,#49107,
#49108,#49109),.UNSPECIFIED.,.F.,.F.,(4,3,3,3,3,3,3,3,3,3,3,3,3,4),(101.654613621017,
102.126569395693,102.624747782989,103.122926170285,103.621104557581,104.119282944877,
104.617461332173,105.115639719469,105.613818106765,106.111996494061,106.610174881358,
107.108353268654,107.60653165595,107.937798928196),.UNSPECIFIED.);
#1206=B_SPLINE_CURVE_WITH_KNOTS('',3,(#49114,#49115,#49116,#49117,#49118,
#49119,#49120,#49121,#49122,#49123,#49124,#49125,#49126,#49127,#49128,#49129,
#49130,#49131,#49132,#49133,#49134,#49135,#49136,#49137,#49138,#49139,#49140,
#49141,#49142,#49143,#49144,#49145,#49146,#49147,#49148,#49149,#49150,#49151,
#49152,#49153,#49154,#49155,#49156),.UNSPECIFIED.,.F.,.F.,(4,3,3,3,3,3,
3,3,3,3,3,3,3,3,4),(-117.190265949363,-117.071921014575,-116.573742627279,
-116.075564239983,-115.577385852687,-115.079207465391,-114.581029078095,
-114.082850690798,-113.584672303502,-113.086493916206,-112.58831552891,
-112.090137141614,-111.591958754318,-111.093780367022,-110.907080642184),
 .UNSPECIFIED.);
#1207=B_SPLINE_CURVE_WITH_KNOTS('',3,(#49157,#49158,#49159,#49160,#49161,
#49162,#49163,#49164,#49165,#49166,#49167,#49168,#49169,#49170,#49171,#49172,
#49173,#49174,#49175,#49176,#49177,#49178,#49179,#49180,#49181,#49182,#49183,
#49184,#49185,#49186,#49187,#49188,#49189,#49190,#49191,#49192,#49193,#49194,
#49195,#49196,#49197,#49198,#49199),.UNSPECIFIED.,.F.,.F.,(4,3,3,3,3,3,
3,3,3,3,3,3,3,3,4),(107.937798928196,108.104710043246,108.602888430542,
109.101066817838,109.599245205134,110.09742359243,110.595601979726,111.093780367022,
111.591958754318,112.090137141614,112.58831552891,113.086493916206,113.584672303502,
114.082850690798,114.220984235376),.UNSPECIFIED.);
#1208=B_SPLINE_CURVE_WITH_KNOTS('',3,(#49204,#49205,#49206,#49207,#49208,
#49209,#49210,#49211,#49212,#49213,#49214,#49215,#49216,#49217,#49218,#49219,
#49220,#49221,#49222,#49223,#49224,#49225,#49226,#49227,#49228,#49229,#49230,
#49231,#49232,#49233,#49234,#49235,#49236,#49237,#49238,#49239,#49240,#49241,
#49242,#49243),.UNSPECIFIED.,.F.,.F.,(4,3,3,3,3,3,3,3,3,3,3,3,3,4),(-123.473451256543,
-123.050061662128,-122.551883274832,-122.053704887536,-121.555526500239,
-121.057348112943,-120.559169725647,-120.060991338351,-119.562812951055,
-119.064634563759,-118.566456176463,-118.068277789167,-117.570099401871,
-117.190265949363),.UNSPECIFIED.);
#1209=B_SPLINE_CURVE_WITH_KNOTS('',3,(#49244,#49245,#49246,#49247,#49248,
#49249,#49250,#49251,#49252,#49253,#49254,#49255,#49256,#49257,#49258,#49259,
#49260,#49261,#49262,#49263,#49264,#49265,#49266,#49267,#49268,#49269,#49270,
#49271,#49272,#49273,#49274,#49275,#49276,#49277,#49278,#49279,#49280,#49281,
#49282,#49283),.UNSPECIFIED.,.F.,.F.,(4,3,3,3,3,3,3,3,3,3,3,3,3,4),(114.220984235376,
114.581029078095,115.079207465391,115.577385852687,116.075564239983,116.573742627279,
117.071921014575,117.570099401871,118.068277789167,118.566456176463,119.064634563759,
119.562812951055,120.060991338351,120.504169542555),.UNSPECIFIED.);
#1210=B_SPLINE_CURVE_WITH_KNOTS('',3,(#49288,#49289,#49290,#49291,#49292,
#49293,#49294,#49295,#49296,#49297,#49298,#49299,#49300,#49301,#49302,#49303,
#49304,#49305,#49306,#49307,#49308,#49309,#49310,#49311,#49312,#49313,#49314,
#49315,#49316,#49317,#49318,#49319,#49320,#49321,#49322,#49323,#49324,#49325,
#49326,#49327,#49328,#49329,#49330),.UNSPECIFIED.,.F.,.F.,(4,3,3,3,3,3,
3,3,3,3,3,3,3,3,4),(-129.756636563722,-129.526380696976,-129.02820230968,
-128.530023922384,-128.031845535088,-127.533667147792,-127.035488760496,
-126.5373103732,-126.039131985904,-125.540953598608,-125.042775211312,-124.544596824016,
-124.04641843672,-123.548240049424,-123.473451256543),.UNSPECIFIED.);
#1211=B_SPLINE_CURVE_WITH_KNOTS('',3,(#49331,#49332,#49333,#49334,#49335,
#49336,#49337,#49338,#49339,#49340,#49341,#49342,#49343,#49344,#49345,#49346,
#49347,#49348,#49349,#49350,#49351,#49352,#49353,#49354,#49355,#49356,#49357,
#49358,#49359,#49360,#49361,#49362,#49363,#49364,#49365,#49366,#49367,#49368,
#49369,#49370,#49371,#49372,#49373),.UNSPECIFIED.,.F.,.F.,(4,3,3,3,3,3,
3,3,3,3,3,3,3,3,4),(120.504169542555,120.559169725647,121.057348112943,
121.555526500239,122.053704887535,122.551883274832,123.050061662128,123.548240049424,
124.04641843672,124.544596824016,125.042775211312,125.540953598608,126.039131985904,
126.5373103732,126.787354849735),.UNSPECIFIED.);
#1212=B_SPLINE_CURVE_WITH_KNOTS('',3,(#49378,#49379,#49380,#49381,#49382,
#49383,#49384,#49385,#49386,#49387,#49388,#49389,#49390,#49391,#49392,#49393,
#49394,#49395,#49396,#49397,#49398,#49399,#49400,#49401,#49402,#49403,#49404,
#49405,#49406,#49407,#49408,#49409,#49410,#49411,#49412,#49413,#49414,#49415,
#49416,#49417,#49418,#49419,#49420),.UNSPECIFIED.,.F.,.F.,(4,3,3,3,3,3,
3,3,3,3,3,3,3,3,4),(-136.039821870902,-136.002699731825,-135.504521344529,
-135.006342957233,-134.508164569937,-134.009986182641,-133.511807795345,
-133.013629408049,-132.515451020753,-132.017272633457,-131.519094246161,
-131.020915858865,-130.522737471569,-130.024559084273,-129.756636563722),
 .UNSPECIFIED.);
#1213=B_SPLINE_CURVE_WITH_KNOTS('',3,(#49421,#49422,#49423,#49424,#49425,
#49426,#49427,#49428,#49429,#49430,#49431,#49432,#49433,#49434,#49435,#49436,
#49437,#49438,#49439,#49440,#49441,#49442,#49443,#49444,#49445,#49446,#49447,
#49448,#49449,#49450,#49451,#49452,#49453,#49454,#49455,#49456,#49457,#49458,
#49459,#49460,#49461,#49462,#49463),.UNSPECIFIED.,.F.,.F.,(4,3,3,3,3,3,
3,3,3,3,3,3,3,3,4),(126.787354849735,127.035488760496,127.533667147792,
128.031845535088,128.530023922384,129.02820230968,129.526380696976,130.024559084273,
130.522737471569,131.020915858865,131.519094246161,132.017272633457,132.515451020753,
133.013629408049,133.070540156915),.UNSPECIFIED.);
#1214=B_SPLINE_CURVE_WITH_KNOTS('',3,(#49468,#49469,#49470,#49471,#49472,
#49473,#49474,#49475,#49476,#49477,#49478,#49479,#49480,#49481,#49482,#49483,
#49484,#49485,#49486,#49487,#49488,#49489,#49490,#49491,#49492,#49493,#49494,
#49495,#49496,#49497,#49498,#49499,#49500,#49501,#49502,#49503,#49504,#49505,
#49506,#49507),.UNSPECIFIED.,.F.,.F.,(4,3,3,3,3,3,3,3,3,3,3,3,3,4),(-142.323007178082,
-141.980840379378,-141.482661992082,-140.984483604786,-140.48630521749,
-139.988126830194,-139.489948442898,-138.991770055602,-138.493591668306,
-137.995413281009,-137.497234893713,-136.999056506417,-136.500878119121,
-136.039821870902),.UNSPECIFIED.);
#1215=B_SPLINE_CURVE_WITH_KNOTS('',3,(#49508,#49509,#49510,#49511,#49512,
#49513,#49514,#49515,#49516,#49517,#49518,#49519,#49520,#49521,#49522,#49523,
#49524,#49525,#49526,#49527,#49528,#49529,#49530,#49531,#49532,#49533,#49534,
#49535,#49536,#49537,#49538,#49539,#49540,#49541,#49542,#49543,#49544,#49545,
#49546,#49547),.UNSPECIFIED.,.F.,.F.,(4,3,3,3,3,3,3,3,3,3,3,3,3,4),(133.070540156915,
133.511807795345,134.009986182641,134.508164569937,135.006342957233,135.504521344529,
136.002699731825,136.500878119121,136.999056506417,137.497234893713,137.995413281009,
138.493591668306,138.991770055602,139.353725464094),.UNSPECIFIED.);
#1216=B_SPLINE_CURVE_WITH_KNOTS('',3,(#49552,#49553,#49554,#49555,#49556,
#49557,#49558,#49559,#49560,#49561,#49562,#49563,#49564,#49565,#49566,#49567,
#49568,#49569,#49570,#49571,#49572,#49573,#49574,#49575,#49576,#49577,#49578,
#49579,#49580,#49581,#49582,#49583,#49584,#49585,#49586,#49587,#49588,#49589,
#49590,#49591,#49592,#49593,#49594),.UNSPECIFIED.,.F.,.F.,(4,3,3,3,3,3,
3,3,3,3,3,3,3,3,4),(-148.606192485261,-148.457159414227,-147.958981026931,
-147.460802639635,-146.962624252339,-146.464445865043,-145.966267477746,
-145.46808909045,-144.969910703154,-144.471732315858,-143.973553928562,
-143.475375541266,-142.97719715397,-142.479018766674,-142.323007178082),
 .UNSPECIFIED.);
#1217=B_SPLINE_CURVE_WITH_KNOTS('',3,(#49595,#49596,#49597,#49598,#49599,
#49600,#49601,#49602,#49603,#49604,#49605,#49606,#49607,#49608,#49609,#49610,
#49611,#49612,#49613,#49614,#49615,#49616,#49617,#49618,#49619,#49620,#49621,
#49622,#49623,#49624,#49625,#49626,#49627,#49628,#49629,#49630,#49631,#49632,
#49633,#49634,#49635,#49636,#49637),.UNSPECIFIED.,.F.,.F.,(4,3,3,3,3,3,
3,3,3,3,3,3,3,3,4),(139.353725464094,139.489948442898,139.988126830194,
140.48630521749,140.984483604786,141.482661992082,141.980840379378,142.479018766674,
142.97719715397,143.475375541266,143.973553928562,144.471732315858,144.969910703154,
145.46808909045,145.636910771274),.UNSPECIFIED.);
#1218=B_SPLINE_CURVE_WITH_KNOTS('',3,(#49642,#49643,#49644,#49645,#49646,
#49647,#49648,#49649,#49650,#49651,#49652,#49653,#49654,#49655,#49656,#49657,
#49658,#49659,#49660,#49661,#49662,#49663,#49664,#49665,#49666,#49667,#49668,
#49669,#49670,#49671,#49672,#49673,#49674,#49675,#49676,#49677,#49678,#49679,
#49680,#49681),.UNSPECIFIED.,.F.,.F.,(4,3,3,3,3,3,3,3,3,3,3,3,3,4),(-154.889377792441,
-154.43530006178,-153.937121674484,-153.438943287187,-152.940764899891,
-152.442586512595,-151.944408125299,-151.446229738003,-150.948051350707,
-150.449872963411,-149.951694576115,-149.453516188819,-148.955337801523,
-148.606192485261),.UNSPECIFIED.);
#1219=B_SPLINE_CURVE_WITH_KNOTS('',3,(#49682,#49683,#49684,#49685,#49686,
#49687,#49688,#49689,#49690,#49691,#49692,#49693,#49694,#49695,#49696,#49697,
#49698,#49699,#49700,#49701,#49702,#49703,#49704,#49705,#49706,#49707,#49708,
#49709,#49710,#49711,#49712,#49713,#49714,#49715,#49716,#49717,#49718,#49719,
#49720,#49721),.UNSPECIFIED.,.F.,.F.,(4,3,3,3,3,3,3,3,3,3,3,3,3,4),(145.636910771274,
145.966267477746,146.464445865043,146.962624252339,147.460802639635,147.958981026931,
148.457159414227,148.955337801523,149.453516188819,149.951694576115,150.449872963411,
150.948051350707,151.446229738003,151.920096078453),.UNSPECIFIED.);
#1220=B_SPLINE_CURVE_WITH_KNOTS('',3,(#49726,#49727,#49728,#49729,#49730,
#49731,#49732,#49733,#49734,#49735,#49736,#49737,#49738,#49739,#49740,#49741,
#49742,#49743,#49744,#49745,#49746,#49747,#49748,#49749,#49750,#49751,#49752,
#49753,#49754,#49755,#49756,#49757,#49758,#49759,#49760,#49761,#49762,#49763,
#49764,#49765,#49766,#49767,#49768),.UNSPECIFIED.,.F.,.F.,(4,3,3,3,3,3,
3,3,3,3,3,3,3,3,4),(-161.17256309962,-160.911619096628,-160.413440709332,
-159.915262322036,-159.41708393474,-158.918905547444,-158.420727160148,
-157.922548772852,-157.424370385556,-156.92619199826,-156.428013610964,
-155.929835223668,-155.431656836372,-154.933478449076,-154.889377792441),
 .UNSPECIFIED.);
#1221=B_SPLINE_CURVE_WITH_KNOTS('',3,(#49769,#49770,#49771,#49772,#49773,
#49774,#49775,#49776,#49777,#49778,#49779,#49780,#49781,#49782,#49783,#49784,
#49785,#49786,#49787,#49788,#49789,#49790,#49791,#49792,#49793,#49794,#49795,
#49796,#49797,#49798,#49799,#49800,#49801,#49802,#49803,#49804,#49805,#49806,
#49807,#49808,#49809,#49810,#49811),.UNSPECIFIED.,.F.,.F.,(4,3,3,3,3,3,
3,3,3,3,3,3,3,3,4),(151.920096078453,151.944408125299,152.442586512595,
152.940764899891,153.438943287187,153.937121674484,154.43530006178,154.933478449076,
155.431656836372,155.929835223668,156.428013610964,156.92619199826,157.424370385556,
157.922548772852,158.203281385633),.UNSPECIFIED.);
#1222=B_SPLINE_CURVE_WITH_KNOTS('',3,(#49816,#49817,#49818,#49819,#49820,
#49821,#49822,#49823,#49824,#49825,#49826,#49827,#49828,#49829,#49830,#49831,
#49832,#49833,#49834,#49835,#49836,#49837,#49838,#49839,#49840,#49841,#49842,
#49843,#49844,#49845,#49846,#49847,#49848,#49849,#49850,#49851,#49852,#49853,
#49854,#49855,#49856,#49857,#49858),.UNSPECIFIED.,.F.,.F.,(4,3,3,3,3,3,
3,3,3,3,3,3,3,3,4),(-167.4557484068,-167.387938131477,-166.889759744181,
-166.391581356885,-165.893402969589,-165.395224582293,-164.897046194997,
-164.398867807701,-163.900689420405,-163.402511033109,-162.904332645813,
-162.406154258517,-161.907975871221,-161.409797483924,-161.17256309962),
 .UNSPECIFIED.);
#1223=B_SPLINE_CURVE_WITH_KNOTS('',3,(#49859,#49860,#49861,#49862,#49863,
#49864,#49865,#49866,#49867,#49868,#49869,#49870,#49871,#49872,#49873,#49874,
#49875,#49876,#49877,#49878,#49879,#49880,#49881,#49882,#49883,#49884,#49885,
#49886,#49887,#49888,#49889,#49890,#49891,#49892,#49893,#49894,#49895,#49896,
#49897,#49898,#49899,#49900,#49901),.UNSPECIFIED.,.F.,.F.,(4,3,3,3,3,3,
3,3,3,3,3,3,3,3,4),(158.203281385633,158.420727160148,158.918905547444,
159.41708393474,159.915262322036,160.413440709332,160.911619096628,161.409797483924,
161.907975871221,162.406154258517,162.904332645813,163.402511033109,163.900689420405,
164.398867807701,164.486466692812),.UNSPECIFIED.);
#1224=B_SPLINE_CURVE_WITH_KNOTS('',3,(#49906,#49907,#49908,#49909,#49910,
#49911,#49912,#49913,#49914,#49915,#49916,#49917,#49918,#49919,#49920,#49921,
#49922,#49923,#49924,#49925,#49926,#49927,#49928,#49929,#49930,#49931,#49932,
#49933,#49934,#49935,#49936,#49937,#49938,#49939,#49940,#49941,#49942,#49943,
#49944,#49945),.UNSPECIFIED.,.F.,.F.,(4,3,3,3,3,3,3,3,3,3,3,3,3,4),(-173.738933713979,
-173.36607877903,-172.867900391734,-172.369722004438,-171.871543617142,
-171.373365229846,-170.87518684255,-170.377008455254,-169.878830067958,
-169.380651680662,-168.882473293365,-168.384294906069,-167.886116518773,
-167.4557484068),.UNSPECIFIED.);
#1225=B_SPLINE_CURVE_WITH_KNOTS('',3,(#49946,#49947,#49948,#49949,#49950,
#49951,#49952,#49953,#49954,#49955,#49956,#49957,#49958,#49959,#49960,#49961,
#49962,#49963,#49964,#49965,#49966,#49967,#49968,#49969,#49970,#49971,#49972,
#49973,#49974,#49975,#49976,#49977,#49978,#49979,#49980,#49981,#49982,#49983,
#49984,#49985),.UNSPECIFIED.,.F.,.F.,(4,3,3,3,3,3,3,3,3,3,3,3,3,4),(164.486466692812,
164.897046194997,165.395224582293,165.893402969589,166.391581356885,166.889759744181,
167.387938131477,167.886116518773,168.384294906069,168.882473293365,169.380651680661,
169.878830067958,170.377008455254,170.769651999992),.UNSPECIFIED.);
#1226=B_SPLINE_CURVE_WITH_KNOTS('',3,(#49990,#49991,#49992,#49993,#49994,
#49995,#49996,#49997,#49998,#49999,#50000,#50001,#50002,#50003,#50004,#50005,
#50006,#50007,#50008,#50009,#50010,#50011,#50012,#50013,#50014,#50015,#50016,
#50017,#50018,#50019,#50020,#50021,#50022,#50023,#50024,#50025,#50026,#50027,
#50028,#50029,#50030,#50031,#50032),.UNSPECIFIED.,.F.,.F.,(4,3,3,3,3,3,
3,3,3,3,3,3,3,3,4),(-180.022119021159,-179.842397813879,-179.344219426583,
-178.846041039287,-178.347862651991,-177.849684264695,-177.351505877398,
-176.853327490102,-176.355149102806,-175.85697071551,-175.358792328214,
-174.860613940918,-174.362435553622,-173.864257166326,-173.738933713979),
 .UNSPECIFIED.);
#1227=B_SPLINE_CURVE_WITH_KNOTS('',3,(#50033,#50034,#50035,#50036,#50037,
#50038,#50039,#50040,#50041,#50042,#50043,#50044,#50045,#50046,#50047,#50048,
#50049,#50050,#50051,#50052,#50053,#50054,#50055,#50056,#50057,#50058,#50059,
#50060,#50061,#50062,#50063,#50064,#50065,#50066,#50067,#50068,#50069,#50070,
#50071,#50072,#50073,#50074,#50075),.UNSPECIFIED.,.F.,.F.,(4,3,3,3,3,3,
3,3,3,3,3,3,3,3,4),(170.769651999992,170.87518684255,171.373365229846,171.871543617142,
172.369722004438,172.867900391734,173.36607877903,173.864257166326,174.362435553622,
174.860613940918,175.358792328214,175.85697071551,176.355149102806,176.853327490102,
177.052837307172),.UNSPECIFIED.);
#1228=B_SPLINE_CURVE_WITH_KNOTS('',3,(#50081,#50082,#50083,#50084),
 .UNSPECIFIED.,.F.,.F.,(4,4),(191.637151868977,191.873336125493),
 .UNSPECIFIED.);
#1229=B_SPLINE_CURVE_WITH_KNOTS('',3,(#50090,#50091,#50092,#50093,#50094,
#50095,#50096,#50097,#50098,#50099,#50100,#50101,#50102,#50103,#50104,#50105,
#50106),.UNSPECIFIED.,.F.,.F.,(4,1,1,1,1,1,1,1,1,1,1,1,1,1,4),(185.353966561798,
185.479290014144,185.97746840144,186.475646788737,186.973825176033,187.472003563329,
187.970181950625,188.468360337921,188.966538725217,189.464717112513,189.962895499809,
190.461073887105,190.959252274401,191.457430661697,191.637151868977),
 .UNSPECIFIED.);
#1230=B_SPLINE_CURVE_WITH_KNOTS('',3,(#50109,#50110,#50111,#50112,#50113,
#50114,#50115,#50116,#50117,#50118,#50119,#50120,#50121,#50122),
 .UNSPECIFIED.,.F.,.F.,(4,1,1,1,1,1,1,1,1,1,1,4),(185.353966561798,185.652635132025,
186.150813519321,186.648991906617,187.147170293913,187.645348681209,188.143527068505,
188.641705455801,189.139883843097,189.638062230393,190.136240617689,190.634419004985),
 .UNSPECIFIED.);
#1231=B_SPLINE_CURVE_WITH_KNOTS('',3,(#50127,#50128,#50129,#50130,#50131,
#50132,#50133,#50134,#50135,#50136,#50137,#50138,#50139,#50140,#50141,#50142),
 .UNSPECIFIED.,.F.,.F.,(4,1,1,1,1,1,1,1,1,1,1,1,1,4),(179.070781254618,
179.501149366592,179.999327753888,180.497506141184,180.99568452848,181.493862915776,
181.992041303072,182.490219690368,182.988398077664,183.48657646496,183.984754852256,
184.482933239552,184.981111626848,185.353966561798),.UNSPECIFIED.);
#1232=B_SPLINE_CURVE_WITH_KNOTS('',3,(#50143,#50144,#50145,#50146,#50147,
#50148,#50149,#50150,#50151,#50152,#50153,#50154,#50155,#50156,#50157,#50158,
#50159),.UNSPECIFIED.,.F.,.F.,(4,1,1,1,1,1,1,1,1,1,1,1,1,1,4),(179.070781254618,
179.176316097176,179.674494484472,180.172672871768,180.670851259064,181.16902964636,
181.667208033656,182.165386420952,182.663564808248,183.161743195545,183.659921582841,
184.158099970137,184.656278357433,185.154456744729,185.353966561798),
 .UNSPECIFIED.);
#1233=B_SPLINE_CURVE_WITH_KNOTS('',3,(#50164,#50165,#50166,#50167,#50168,
#50169,#50170,#50171,#50172,#50173,#50174,#50175,#50176,#50177,#50178,#50179,
#50180),.UNSPECIFIED.,.F.,.F.,(4,1,1,1,1,1,1,1,1,1,1,1,1,1,4),(172.787595947439,
173.024830331743,173.523008719039,174.021187106335,174.519365493631,175.017543880927,
175.515722268223,176.013900655519,176.512079042815,177.010257430111,177.508435817407,
178.006614204703,178.504792592,179.002970979296,179.070781254618),
 .UNSPECIFIED.);
#1234=B_SPLINE_CURVE_WITH_KNOTS('',3,(#50181,#50182,#50183,#50184,#50185,
#50186,#50187,#50188,#50189,#50190,#50191,#50192,#50193,#50194,#50195,#50196),
 .UNSPECIFIED.,.F.,.F.,(4,1,1,1,1,1,1,1,1,1,1,1,1,4),(172.787595947439,
173.198175449623,173.696353836919,174.194532224215,174.692710611511,175.190888998808,
175.689067386104,176.1872457734,176.685424160696,177.183602547992,177.681780935288,
178.179959322584,178.67813770988,179.070781254618),.UNSPECIFIED.);
#1235=B_SPLINE_CURVE_WITH_KNOTS('',3,(#50201,#50202,#50203,#50204,#50205,
#50206,#50207,#50208,#50209,#50210,#50211,#50212,#50213,#50214,#50215,#50216,
#50217),.UNSPECIFIED.,.F.,.F.,(4,1,1,1,1,1,1,1,1,1,1,1,1,1,4),(166.504410640259,
166.548511296894,167.04668968419,167.544868071486,168.043046458782,168.541224846078,
169.039403233374,169.53758162067,170.035760007966,170.533938395263,171.032116782559,
171.530295169855,172.028473557151,172.526651944447,172.787595947439),
 .UNSPECIFIED.);
#1236=B_SPLINE_CURVE_WITH_KNOTS('',3,(#50218,#50219,#50220,#50221,#50222,
#50223,#50224,#50225,#50226,#50227,#50228,#50229,#50230,#50231,#50232,#50233,
#50234),.UNSPECIFIED.,.F.,.F.,(4,1,1,1,1,1,1,1,1,1,1,1,1,1,4),(166.504410640259,
166.721856414774,167.220034802071,167.718213189367,168.216391576663,168.714569963959,
169.212748351255,169.710926738551,170.209105125847,170.707283513143,171.205461900439,
171.703640287735,172.201818675031,172.699997062327,172.787595947439),
 .UNSPECIFIED.);
#1237=B_SPLINE_CURVE_WITH_KNOTS('',3,(#50239,#50240,#50241,#50242,#50243,
#50244,#50245,#50246,#50247,#50248,#50249,#50250,#50251,#50252,#50253,#50254),
 .UNSPECIFIED.,.F.,.F.,(4,1,1,1,1,1,1,1,1,1,1,1,1,4),(160.22122533308,160.570370649341,
161.068549036637,161.566727423933,162.064905811229,162.563084198526,163.061262585822,
163.559440973118,164.057619360414,164.55579774771,165.053976135006,165.552154522302,
166.050332909598,166.504410640259),.UNSPECIFIED.);
#1238=B_SPLINE_CURVE_WITH_KNOTS('',3,(#50255,#50256,#50257,#50258,#50259,
#50260,#50261,#50262,#50263,#50264,#50265,#50266,#50267,#50268,#50269,#50270,
#50271),.UNSPECIFIED.,.F.,.F.,(4,1,1,1,1,1,1,1,1,1,1,1,1,1,4),(160.22122533308,
160.245537379926,160.743715767222,161.241894154518,161.740072541814,162.23825092911,
162.736429316406,163.234607703702,163.732786090998,164.230964478294,164.72914286559,
165.227321252886,165.725499640182,166.223678027478,166.504410640259),
 .UNSPECIFIED.);
#1239=B_SPLINE_CURVE_WITH_KNOTS('',3,(#50276,#50277,#50278,#50279,#50280,
#50281,#50282,#50283,#50284,#50285,#50286,#50287,#50288,#50289,#50290,#50291,
#50292),.UNSPECIFIED.,.F.,.F.,(4,1,1,1,1,1,1,1,1,1,1,1,1,1,4),(153.9380400259,
154.094051614492,154.592230001789,155.090408389085,155.588586776381,156.086765163677,
156.584943550973,157.083121938269,157.581300325565,158.079478712861,158.577657100157,
159.075835487453,159.574013874749,160.072192262045,160.22122533308),
 .UNSPECIFIED.);
#1240=B_SPLINE_CURVE_WITH_KNOTS('',3,(#50293,#50294,#50295,#50296,#50297,
#50298,#50299,#50300,#50301,#50302,#50303,#50304,#50305,#50306,#50307,#50308),
 .UNSPECIFIED.,.F.,.F.,(4,1,1,1,1,1,1,1,1,1,1,1,1,4),(153.9380400259,154.267396732373,
154.765575119669,155.263753506965,155.761931894261,156.260110281557,156.758288668853,
157.256467056149,157.754645443445,158.252823830741,158.751002218037,159.249180605333,
159.74735899263,160.22122533308),.UNSPECIFIED.);
#1241=B_SPLINE_CURVE_WITH_KNOTS('',3,(#50313,#50314,#50315,#50316,#50317,
#50318,#50319,#50320,#50321,#50322,#50323,#50324,#50325,#50326,#50327,#50328),
 .UNSPECIFIED.,.F.,.F.,(4,1,1,1,1,1,1,1,1,1,1,1,1,4),(147.65485471872,148.11591096694,
148.614089354236,149.112267741532,149.610446128828,150.108624516124,150.60680290342,
151.104981290716,151.603159678012,152.101338065308,152.599516452604,153.0976948399,
153.595873227196,153.9380400259),.UNSPECIFIED.);
#1242=B_SPLINE_CURVE_WITH_KNOTS('',3,(#50329,#50330,#50331,#50332,#50333,
#50334,#50335,#50336,#50337,#50338,#50339,#50340,#50341,#50342,#50343,#50344,
#50345),.UNSPECIFIED.,.F.,.F.,(4,1,1,1,1,1,1,1,1,1,1,1,1,1,4),(147.65485471872,
147.791077697524,148.28925608482,148.787434472116,149.285612859412,149.783791246708,
150.281969634004,150.7801480213,151.278326408596,151.776504795893,152.274683183189,
152.772861570485,153.271039957781,153.769218345077,153.9380400259),
 .UNSPECIFIED.);
#1243=B_SPLINE_CURVE_WITH_KNOTS('',3,(#50350,#50351,#50352,#50353,#50354,
#50355,#50356,#50357,#50358,#50359,#50360,#50361,#50362,#50363,#50364,#50365,
#50366),.UNSPECIFIED.,.F.,.F.,(4,1,1,1,1,1,1,1,1,1,1,1,1,1,4),(141.371669411541,
141.639591932091,142.137770319387,142.635948706683,143.134127093979,143.632305481275,
144.130483868571,144.628662255867,145.126840643163,145.625019030459,146.123197417755,
146.621375805052,147.119554192348,147.617732579644,147.65485471872),
 .UNSPECIFIED.);
#1244=B_SPLINE_CURVE_WITH_KNOTS('',3,(#50367,#50368,#50369,#50370,#50371,
#50372,#50373,#50374,#50375,#50376,#50377,#50378,#50379,#50380,#50381,#50382),
 .UNSPECIFIED.,.F.,.F.,(4,1,1,1,1,1,1,1,1,1,1,1,1,4),(141.371669411541,
141.812937049971,142.311115437267,142.809293824563,143.307472211859,143.805650599156,
144.303828986452,144.802007373748,145.300185761044,145.79836414834,146.296542535636,
146.794720922932,147.292899310228,147.65485471872),.UNSPECIFIED.);
#1245=B_SPLINE_CURVE_WITH_KNOTS('',3,(#50387,#50388,#50389,#50390,#50391,
#50392,#50393,#50394,#50395,#50396,#50397,#50398,#50399,#50400,#50401,#50402,
#50403),.UNSPECIFIED.,.F.,.F.,(4,1,1,1,1,1,1,1,1,1,1,1,1,1,4),(135.088484104361,
135.163272897242,135.661451284538,136.159629671834,136.65780805913,137.155986446426,
137.654164833722,138.152343221018,138.650521608314,139.148699995611,139.646878382907,
140.145056770203,140.643235157499,141.141413544795,141.371669411541),
 .UNSPECIFIED.);
#1246=B_SPLINE_CURVE_WITH_KNOTS('',3,(#50404,#50405,#50406,#50407,#50408,
#50409,#50410,#50411,#50412,#50413,#50414,#50415,#50416,#50417,#50418,#50419,
#50420),.UNSPECIFIED.,.F.,.F.,(4,1,1,1,1,1,1,1,1,1,1,1,1,1,4),(135.088484104361,
135.336618015122,135.834796402419,136.332974789715,136.831153177011,137.329331564307,
137.827509951603,138.325688338899,138.823866726195,139.322045113491,139.820223500787,
140.318401888083,140.816580275379,141.314758662675,141.371669411541),
 .UNSPECIFIED.);
#1247=B_SPLINE_CURVE_WITH_KNOTS('',3,(#50425,#50426,#50427,#50428,#50429,
#50430,#50431,#50432,#50433,#50434,#50435,#50436,#50437,#50438,#50439,#50440),
 .UNSPECIFIED.,.F.,.F.,(4,1,1,1,1,1,1,1,1,1,1,1,1,4),(128.805298797182,
129.185132249689,129.683310636985,130.181489024281,130.679667411577,131.177845798874,
131.67602418617,132.174202573466,132.672380960762,133.170559348058,133.668737735354,
134.16691612265,134.665094509946,135.088484104361),.UNSPECIFIED.);
#1248=B_SPLINE_CURVE_WITH_KNOTS('',3,(#50441,#50442,#50443,#50444,#50445,
#50446,#50447,#50448,#50449,#50450,#50451,#50452,#50453,#50454,#50455,#50456,
#50457),.UNSPECIFIED.,.F.,.F.,(4,1,1,1,1,1,1,1,1,1,1,1,1,1,4),(128.805298797182,
128.860298980274,129.35847736757,129.856655754866,130.354834142162,130.853012529458,
131.351190916754,131.84936930405,132.347547691346,132.845726078642,133.343904465938,
133.842082853234,134.34026124053,134.838439627826,135.088484104361),
 .UNSPECIFIED.);
#1249=B_SPLINE_CURVE_WITH_KNOTS('',3,(#50462,#50463,#50464,#50465,#50466,
#50467,#50468,#50469,#50470,#50471,#50472,#50473,#50474,#50475,#50476,#50477,
#50478),.UNSPECIFIED.,.F.,.F.,(4,1,1,1,1,1,1,1,1,1,1,1,1,1,4),(122.522113490002,
122.70881321484,123.206991602137,123.705169989433,124.203348376729,124.701526764025,
125.199705151321,125.697883538617,126.196061925913,126.694240313209,127.192418700505,
127.690597087801,128.188775475097,128.686953862393,128.805298797182),
 .UNSPECIFIED.);
#1250=B_SPLINE_CURVE_WITH_KNOTS('',3,(#50479,#50480,#50481,#50482,#50483,
#50484,#50485,#50486,#50487,#50488,#50489,#50490,#50491,#50492,#50493,#50494),
 .UNSPECIFIED.,.F.,.F.,(4,1,1,1,1,1,1,1,1,1,1,1,1,4),(122.522113490002,
122.882158332721,123.380336720017,123.878515107313,124.376693494609,124.874871881905,
125.373050269201,125.871228656497,126.369407043793,126.867585431089,127.365763818385,
127.863942205682,128.362120592978,128.805298797182),.UNSPECIFIED.);
#1251=B_SPLINE_CURVE_WITH_KNOTS('',3,(#50499,#50500,#50501,#50502,#50503,
#50504,#50505,#50506,#50507,#50508,#50509,#50510,#50511,#50512,#50513,#50514),
 .UNSPECIFIED.,.F.,.F.,(4,1,1,1,1,1,1,1,1,1,1,1,1,4),(116.238928182823,
116.730672567288,117.228850954584,117.72702934188,118.225207729176,118.723386116472,
119.221564503768,119.719742891064,120.21792127836,120.716099665656,121.214278052952,
121.712456440248,122.210634827544,122.522113490002),.UNSPECIFIED.);
#1252=B_SPLINE_CURVE_WITH_KNOTS('',3,(#50515,#50516,#50517,#50518,#50519,
#50520,#50521,#50522,#50523,#50524,#50525,#50526,#50527,#50528,#50529,#50530,
#50531),.UNSPECIFIED.,.F.,.F.,(4,1,1,1,1,1,1,1,1,1,1,1,1,1,4),(116.238928182823,
116.405839297872,116.904017685168,117.402196072464,117.90037445976,118.398552847056,
118.896731234352,119.394909621648,119.893088008945,120.391266396241,120.889444783537,
121.387623170833,121.885801558129,122.383979945425,122.522113490002),
 .UNSPECIFIED.);
#1253=B_SPLINE_CURVE_WITH_KNOTS('',3,(#50536,#50537,#50538,#50539,#50540,
#50541,#50542,#50543,#50544,#50545,#50546,#50547,#50548,#50549,#50550,#50551,
#50552),.UNSPECIFIED.,.F.,.F.,(4,1,1,1,1,1,1,1,1,1,1,1,1,1,4),(109.955742875643,
110.254353532439,110.752531919735,111.250710307031,111.748888694327,112.247067081623,
112.745245468919,113.243423856215,113.741602243511,114.239780630807,114.737959018103,
115.2361374054,115.734315792696,116.232494179992,116.238928182823),
 .UNSPECIFIED.);
#1254=B_SPLINE_CURVE_WITH_KNOTS('',3,(#50553,#50554,#50555,#50556,#50557,
#50558,#50559,#50560,#50561,#50562,#50563,#50564,#50565,#50566,#50567,#50568),
 .UNSPECIFIED.,.F.,.F.,(4,1,1,1,1,1,1,1,1,1,1,1,1,4),(109.955742875643,
110.427698650319,110.925877037615,111.424055424911,111.922233812207,112.420412199504,
112.9185905868,113.416768974096,113.914947361392,114.413125748688,114.911304135984,
115.40948252328,115.907660910576,116.238928182823),.UNSPECIFIED.);
#1255=B_SPLINE_CURVE_WITH_KNOTS('',3,(#50573,#50574,#50575,#50576,#50577,
#50578,#50579,#50580,#50581,#50582,#50583,#50584,#50585,#50586,#50587,#50588,
#50589),.UNSPECIFIED.,.F.,.F.,(4,1,1,1,1,1,1,1,1,1,1,1,1,1,4),(103.672557568463,
103.77803449759,104.276212884886,104.774391272182,105.272569659478,105.770748046774,
106.26892643407,106.767104821366,107.265283208663,107.763461595959,108.261639983255,
108.759818370551,109.257996757847,109.756175145143,109.955742875643),
 .UNSPECIFIED.);
#1256=B_SPLINE_CURVE_WITH_KNOTS('',3,(#50590,#50591,#50592,#50593,#50594,
#50595,#50596,#50597,#50598,#50599,#50600,#50601,#50602,#50603,#50604,#50605,
#50606),.UNSPECIFIED.,.F.,.F.,(4,1,1,1,1,1,1,1,1,1,1,1,1,1,4),(103.672557568463,
103.95137961547,104.449558002767,104.947736390063,105.445914777359,105.944093164655,
106.442271551951,106.940449939247,107.438628326543,107.936806713839,108.434985101135,
108.933163488431,109.431341875727,109.929520263023,109.955742875643),
 .UNSPECIFIED.);
#1257=B_SPLINE_CURVE_WITH_KNOTS('',3,(#50611,#50612,#50613,#50614,#50615,
#50616,#50617,#50618,#50619,#50620,#50621,#50622,#50623,#50624,#50625,#50626),
 .UNSPECIFIED.,.F.,.F.,(4,1,1,1,1,1,1,1,1,1,1,1,1,4),(97.3893722612837,
97.7998938500373,98.2980722373334,98.7962506246294,99.2944290119255,99.7926073992216,
100.290785786518,100.788964173814,101.28714256111,101.785320948406,102.283499335702,
102.781677722998,103.279856110294,103.672557568463),.UNSPECIFIED.);
#1258=B_SPLINE_CURVE_WITH_KNOTS('',3,(#50627,#50628,#50629,#50630,#50631,
#50632,#50633,#50634,#50635,#50636,#50637,#50638,#50639,#50640,#50641,#50642,
#50643),.UNSPECIFIED.,.F.,.F.,(4,1,1,1,1,1,1,1,1,1,1,1,1,1,4),(97.3893722612837,
97.4750605806217,97.9732389679177,98.4714173552138,98.9695957425099,99.4677741298059,
99.965952517102,100.464130904398,100.962309291694,101.46048767899,101.958666066286,
102.456844453582,102.955022840878,103.453201228174,103.672557568463),
 .UNSPECIFIED.);
#1259=B_SPLINE_CURVE_WITH_KNOTS('',3,(#50648,#50649,#50650,#50651,#50652,
#50653,#50654,#50655,#50656,#50657,#50658,#50659,#50660,#50661,#50662,#50663,
#50664),.UNSPECIFIED.,.F.,.F.,(4,1,1,1,1,1,1,1,1,1,1,1,1,1,4),(91.1061869541041,
91.3235748151885,91.8217532024846,92.3199315897806,92.8181099770767,93.3162883643727,
93.8144667516688,94.3126451389649,94.8108235262609,95.309001913557,95.8071803008531,
96.3053586881491,96.8035370754452,97.3017154627413,97.3893722612837),
 .UNSPECIFIED.);
#1260=B_SPLINE_CURVE_WITH_KNOTS('',3,(#50665,#50666,#50667,#50668,#50669,
#50670,#50671,#50672,#50673,#50674,#50675,#50676,#50677,#50678,#50679,#50680),
 .UNSPECIFIED.,.F.,.F.,(4,1,1,1,1,1,1,1,1,1,1,1,1,4),(91.1061869541041,
91.4969199330689,91.995098320365,92.493276707661,92.9914550949571,93.4896334822532,
93.9878118695492,94.4859902568453,94.9841686441413,95.4823470314374,95.9805254187335,
96.4787038060295,96.9768821933256,97.3893722612837),.UNSPECIFIED.);
#1261=B_SPLINE_CURVE_WITH_KNOTS('',3,(#50685,#50686,#50687,#50688,#50689,
#50690,#50691,#50692,#50693,#50694,#50695,#50696,#50697,#50698,#50699,#50700,
#50701),.UNSPECIFIED.,.F.,.F.,(4,1,1,1,1,1,1,1,1,1,1,1,1,1,4),(84.8230016469245,
84.8472557803397,85.3454341676357,85.8436125549318,86.3417909422279,86.8399693295239,
87.33814771682,87.8363261041161,88.3345044914121,88.8326828787082,89.3308612660042,
89.8290396533003,90.3272180405964,90.8253964278924,91.1061869541041),
 .UNSPECIFIED.);
#1262=B_SPLINE_CURVE_WITH_KNOTS('',3,(#50702,#50703,#50704,#50705,#50706,
#50707,#50708,#50709,#50710,#50711,#50712,#50713,#50714,#50715,#50716,#50717,
#50718),.UNSPECIFIED.,.F.,.F.,(4,1,1,1,1,1,1,1,1,1,1,1,1,1,4),(84.8230016469245,
85.0206008982201,85.5187792855161,86.0169576728122,86.5151360601083,87.0133144474043,
87.5114928347004,88.0096712219965,88.5078496092925,89.0060279965886,89.5042063838847,
90.0023847711807,90.5005631584768,90.9987415457728,91.1061869541041),
 .UNSPECIFIED.);
#1263=B_SPLINE_CURVE_WITH_KNOTS('',3,(#50723,#50724,#50725,#50726,#50727,
#50728,#50729,#50730,#50731,#50732,#50733,#50734,#50735,#50736,#50737,#50738),
 .UNSPECIFIED.,.F.,.F.,(4,1,1,1,1,1,1,1,1,1,1,1,1,4),(78.539816339745,78.8691151327869,
79.367293520083,79.865471907379,80.3636502946751,80.8618286819712,81.3600070692672,
81.8581854565633,82.3563638438594,82.8545422311554,83.3527206184515,83.8508990057476,
84.3490773930436,84.8230016469245),.UNSPECIFIED.);
#1264=B_SPLINE_CURVE_WITH_KNOTS('',3,(#50739,#50740,#50741,#50742,#50743,
#50744,#50745,#50746,#50747,#50748,#50749,#50750,#50751,#50752,#50753,#50754,
#50755),.UNSPECIFIED.,.F.,.F.,(4,1,1,1,1,1,1,1,1,1,1,1,1,1,4),(78.539816339745,
78.5442818633713,79.0424602506673,79.5406386379634,80.0388170252594,80.5369954125555,
81.0351737998516,81.5333521871476,82.0315305744437,82.5297089617398,83.0278873490358,
83.5260657363319,84.024244123628,84.522422510924,84.8230016469245),
 .UNSPECIFIED.);
#1265=B_SPLINE_CURVE_WITH_KNOTS('',3,(#50760,#50761,#50762,#50763,#50764,
#50765,#50766,#50767,#50768,#50769,#50770,#50771,#50772,#50773,#50774,#50775,
#50776),.UNSPECIFIED.,.F.,.F.,(4,1,1,1,1,1,1,1,1,1,1,1,1,1,4),(72.2566310325654,
72.3927960979381,72.8909744852342,73.3891528725302,73.8873312598263,74.3855096471223,
74.8836880344184,75.3818664217145,75.8800448090105,76.3782231963066,76.8764015836027,
77.3745799708987,77.8727583581948,78.3709367454909,78.539816339745),
 .UNSPECIFIED.);
#1266=B_SPLINE_CURVE_WITH_KNOTS('',3,(#50777,#50778,#50779,#50780,#50781,
#50782,#50783,#50784,#50785,#50786,#50787,#50788,#50789,#50790,#50791,#50792),
 .UNSPECIFIED.,.F.,.F.,(4,1,1,1,1,1,1,1,1,1,1,1,1,4),(72.2566310325654,
72.5661412158185,73.0643196031146,73.5624979904106,74.0606763777067,74.5588547650028,
75.0570331522988,75.5552115395949,76.053389926891,76.551568314187,77.0497467014831,
77.5479250887791,78.0461034760752,78.539816339745),.UNSPECIFIED.);
#1267=B_SPLINE_CURVE_WITH_KNOTS('',3,(#50797,#50798,#50799,#50800,#50801,
#50802,#50803,#50804,#50805,#50806,#50807,#50808,#50809,#50810,#50811,#50812),
 .UNSPECIFIED.,.F.,.F.,(4,1,1,1,1,1,1,1,1,1,1,1,1,4),(65.9734457253858,
66.4146554503853,66.9128338376814,67.4110122249775,67.9091906122735,68.4073689995696,
68.9055473868656,69.4037257741617,69.9019041614578,70.4000825487538,70.8982609360499,
71.396439323346,71.894617710642,72.2566310325654),.UNSPECIFIED.);
#1268=B_SPLINE_CURVE_WITH_KNOTS('',3,(#50813,#50814,#50815,#50816,#50817,
#50818,#50819,#50820,#50821,#50822,#50823,#50824,#50825,#50826,#50827,#50828,
#50829),.UNSPECIFIED.,.F.,.F.,(4,1,1,1,1,1,1,1,1,1,1,1,1,1,4),(65.9734457253858,
66.0898221809697,66.5880005682658,67.0861789555618,67.5843573428579,68.0825357301539,
68.58071411745,69.0788925047461,69.5770708920421,70.0752492793382,70.5734276666342,
71.0716060539303,71.5697844412264,72.0679628285224,72.2566310325654),
 .UNSPECIFIED.);
#1269=B_SPLINE_CURVE_WITH_KNOTS('',3,(#50834,#50835,#50836,#50837,#50838,
#50839,#50840,#50841,#50842,#50843,#50844,#50845,#50846,#50847,#50848,#50849,
#50850),.UNSPECIFIED.,.F.,.F.,(4,1,1,1,1,1,1,1,1,1,1,1,1,1,4),(59.6902604182062,
59.9383364155365,60.4365148028326,60.9346931901286,61.4328715774247,61.9310499647208,
62.4292283520168,62.9274067393129,63.425585126609,63.923763513905,64.4219419012011,
64.9201202884971,65.4182986757932,65.9164770630893,65.9734457253858),
 .UNSPECIFIED.);
#1270=B_SPLINE_CURVE_WITH_KNOTS('',3,(#50851,#50852,#50853,#50854,#50855,
#50856,#50857,#50858,#50859,#50860,#50861,#50862,#50863,#50864,#50865,#50866),
 .UNSPECIFIED.,.F.,.F.,(4,1,1,1,1,1,1,1,1,1,1,1,1,4),(59.6902604182062,
60.1116815334169,60.609859920713,61.108038308009,61.6062166953051,62.1043950826012,
62.6025734698972,63.1007518571933,63.5989302444894,64.0971086317854,64.5952870190815,
65.0934654063776,65.5916437936736,65.9734457253858),.UNSPECIFIED.);
#1271=B_SPLINE_CURVE_WITH_KNOTS('',3,(#50871,#50872,#50873,#50874,#50875,
#50876,#50877,#50878,#50879,#50880,#50881,#50882,#50883,#50884,#50885,#50886,
#50887),.UNSPECIFIED.,.F.,.F.,(4,1,1,1,1,1,1,1,1,1,1,1,1,1,4),(53.4070751110266,
53.4620173806877,53.9601957679837,54.4583741552798,54.9565525425759,55.4547309298719,
55.952909317168,56.4510877044641,56.9492660917601,57.4474444790562,57.9456228663523,
58.4438012536483,58.9419796409444,59.4401580282404,59.6902604182062),
 .UNSPECIFIED.);
#1272=B_SPLINE_CURVE_WITH_KNOTS('',3,(#50888,#50889,#50890,#50891,#50892,
#50893,#50894,#50895,#50896,#50897,#50898,#50899,#50900,#50901,#50902,#50903,
#50904),.UNSPECIFIED.,.F.,.F.,(4,1,1,1,1,1,1,1,1,1,1,1,1,1,4),(53.4070751110266,
53.6353624985681,54.1335408858642,54.6317192731602,55.1298976604563,55.6280760477524,
56.1262544350484,56.6244328223445,57.1226112096405,57.6207895969366,58.1189679842327,
58.6171463715287,59.1153247588248,59.6135031461209,59.6902604182062),
 .UNSPECIFIED.);
#1273=B_SPLINE_CURVE_WITH_KNOTS('',3,(#50909,#50910,#50911,#50912,#50913,
#50914,#50915,#50916,#50917,#50918,#50919,#50920,#50921,#50922,#50923,#50924),
 .UNSPECIFIED.,.F.,.F.,(4,1,1,1,1,1,1,1,1,1,1,1,1,4),(47.123889803847,47.4838767331349,
47.982055120431,48.480233507727,48.9784118950231,49.4765902823192,49.9747686696152,
50.4729470569113,50.9711254442074,51.4693038315034,51.9674822187995,52.4656606060956,
52.9638389933916,53.4070751110266),.UNSPECIFIED.);
#1274=B_SPLINE_CURVE_WITH_KNOTS('',3,(#50925,#50926,#50927,#50928,#50929,
#50930,#50931,#50932,#50933,#50934,#50935,#50936,#50937,#50938,#50939,#50940,
#50941),.UNSPECIFIED.,.F.,.F.,(4,1,1,1,1,1,1,1,1,1,1,1,1,1,4),(47.123889803847,
47.1590434637193,47.6572218510153,48.1554002383114,48.6535786256075,49.1517570129035,
49.6499354001996,50.1481137874957,50.6462921747917,51.1444705620878,51.6426489493839,
52.1408273366799,52.639005723976,53.137184111272,53.4070751110266),
 .UNSPECIFIED.);
#1275=B_SPLINE_CURVE_WITH_KNOTS('',3,(#50946,#50947,#50948,#50949,#50950,
#50951,#50952,#50953,#50954,#50955,#50956,#50957,#50958,#50959,#50960,#50961,
#50962),.UNSPECIFIED.,.F.,.F.,(4,1,1,1,1,1,1,1,1,1,1,1,1,1,4),(40.8407044966674,
41.0075576982861,41.5057360855822,42.0039144728782,42.5020928601743,43.0002712474704,
43.4984496347664,43.9966280220625,44.4948064093585,44.9929847966546,45.4911631839507,
45.9893415712467,46.4875199585428,46.9856983458389,47.123889803847),
 .UNSPECIFIED.);
#1276=B_SPLINE_CURVE_WITH_KNOTS('',3,(#50963,#50964,#50965,#50966,#50967,
#50968,#50969,#50970,#50971,#50972,#50973,#50974,#50975,#50976,#50977,#50978),
 .UNSPECIFIED.,.F.,.F.,(4,1,1,1,1,1,1,1,1,1,1,1,1,4),(40.8407044966674,
41.1809028161665,41.6790812034626,42.1772595907587,42.6754379780547,43.1736163653508,
43.6717947526468,44.1699731399429,44.668151527239,45.166329914535,45.6645083018311,
46.1626866891272,46.6608650764232,47.123889803847),.UNSPECIFIED.);
#1277=B_SPLINE_CURVE_WITH_KNOTS('',3,(#50983,#50984,#50985,#50986,#50987,
#50988,#50989,#50990,#50991,#50992,#50993,#50994,#50995,#50996,#50997,#50998),
 .UNSPECIFIED.,.F.,.F.,(4,1,1,1,1,1,1,1,1,1,1,1,1,4),(34.5575191894878,
35.0294170507333,35.5275954380294,36.0257738253255,36.5239522126215,37.0221305999176,
37.5203089872137,38.0184873745097,38.5166657618058,39.0148441491019,39.5130225363979,
40.011200923694,40.50937931099,40.8407044966674),.UNSPECIFIED.);
#1278=B_SPLINE_CURVE_WITH_KNOTS('',3,(#50999,#51000,#51001,#51002,#51003,
#51004,#51005,#51006,#51007,#51008,#51009,#51010,#51011,#51012,#51013,#51014,
#51015),.UNSPECIFIED.,.F.,.F.,(4,1,1,1,1,1,1,1,1,1,1,1,1,1,4),(34.5575191894878,
34.7045837813177,35.2027621686138,35.7009405559098,36.1991189432059,36.697297330502,
37.195475717798,37.6936541050941,38.1918324923901,38.6900108796862,39.1881892669823,
39.6863676542783,40.1845460415744,40.6827244288705,40.8407044966674),
 .UNSPECIFIED.);
#1279=B_SPLINE_CURVE_WITH_KNOTS('',3,(#51020,#51021,#51022,#51023,#51024,
#51025,#51026,#51027,#51028,#51029,#51030,#51031,#51032,#51033,#51034,#51035,
#51036),.UNSPECIFIED.,.F.,.F.,(4,1,1,1,1,1,1,1,1,1,1,1,1,1,4),(28.2743338823082,
28.5530980158845,29.0512764031806,29.5494547904767,30.0476331777727,30.5458115650688,
31.0439899523648,31.5421683396609,32.040346726957,32.538525114253,33.0367035015491,
33.5348818888452,34.0330602761412,34.5312386634373,34.5575191894878),
 .UNSPECIFIED.);
#1280=B_SPLINE_CURVE_WITH_KNOTS('',3,(#51037,#51038,#51039,#51040,#51041,
#51042,#51043,#51044,#51045,#51046,#51047,#51048,#51049,#51050,#51051,#51052),
 .UNSPECIFIED.,.F.,.F.,(4,1,1,1,1,1,1,1,1,1,1,1,1,4),(28.2743338823082,
28.7264431337649,29.224621521061,29.7227999083571,30.2209782956531,30.7191566829492,
31.2173350702453,31.7155134575413,32.2136918448374,32.7118702321334,33.2100486194295,
33.7082270067256,34.2064053940216,34.5575191894878),.UNSPECIFIED.);
#1281=B_SPLINE_CURVE_WITH_KNOTS('',3,(#51057,#51058,#51059,#51060,#51061,
#51062,#51063,#51064,#51065,#51066,#51067,#51068,#51069,#51070,#51071,#51072,
#51073),.UNSPECIFIED.,.F.,.F.,(4,1,1,1,1,1,1,1,1,1,1,1,1,1,4),(21.9911485751286,
22.0767789810357,22.5749573683318,23.0731357556278,23.5713141429239,24.06949253022,
24.567670917516,25.0658493048121,25.5640276921081,26.0622060794042,26.5603844667003,
27.0585628539963,27.5567412412924,28.0549196285885,28.2743338823082),
 .UNSPECIFIED.);
#1282=B_SPLINE_CURVE_WITH_KNOTS('',3,(#51074,#51075,#51076,#51077,#51078,
#51079,#51080,#51081,#51082,#51083,#51084,#51085,#51086,#51087,#51088,#51089,
#51090),.UNSPECIFIED.,.F.,.F.,(4,1,1,1,1,1,1,1,1,1,1,1,1,1,4),(21.9911485751286,
22.2501240989161,22.7483024862122,23.2464808735082,23.7446592608043,24.2428376481004,
24.7410160353964,25.2391944226925,25.7373728099886,26.2355511972846,26.7337295845807,
27.2319079718768,27.7300863591728,28.2282647464689,28.2743338823082),
 .UNSPECIFIED.);
#1283=B_SPLINE_CURVE_WITH_KNOTS('',3,(#51095,#51096,#51097,#51098,#51099,
#51100,#51101,#51102,#51103,#51104,#51105,#51106,#51107,#51108,#51109,#51110),
 .UNSPECIFIED.,.F.,.F.,(4,1,1,1,1,1,1,1,1,1,1,1,1,4),(15.707963267949,16.0986383334829,
16.596816720779,17.0949951080751,17.5931734953711,18.0913518826672,18.5895302699633,
19.0877086572593,19.5858870445554,20.0840654318515,20.5822438191475,21.0804222064436,
21.5786005937396,21.9911485751286),.UNSPECIFIED.);
#1284=B_SPLINE_CURVE_WITH_KNOTS('',3,(#51111,#51112,#51113,#51114,#51115,
#51116,#51117,#51118,#51119,#51120,#51121,#51122,#51123,#51124,#51125,#51126,
#51127),.UNSPECIFIED.,.F.,.F.,(4,1,1,1,1,1,1,1,1,1,1,1,1,1,4),(15.707963267949,
15.7738050640673,16.2719834513634,16.7701618386594,17.2683402259555,17.7665186132516,
18.2646970005476,18.7628753878437,19.2610537751397,19.7592321624358,20.2574105497319,
20.7555889370279,21.253767324324,21.7519457116201,21.9911485751286),
 .UNSPECIFIED.);
#1285=B_SPLINE_CURVE_WITH_KNOTS('',3,(#51130,#51131,#51132,#51133,#51134,
#51135,#51136,#51137,#51138,#51139,#51140,#51141,#51142,#51143,#51144,#51145,
#51146,#51147,#51148,#51149,#51150,#51151,#51152,#51153,#51154,#51155,#51156,
#51157,#51158,#51159,#51160,#51161,#51162,#51163,#51164,#51165,#51166,#51167,
#51168,#51169,#51170,#51171,#51172,#51173,#51174,#51175,#51176,#51177,#51178,
#51179,#51180,#51181,#51182,#51183,#51184,#51185,#51186,#51187,#51188,#51189,
#51190,#51191,#51192,#51193,#51194,#51195,#51196,#51197,#51198,#51199,#51200,
#51201,#51202),.UNSPECIFIED.,.F.,.F.,(4,3,3,3,3,3,3,3,3,3,3,3,3,3,3,3,3,
3,3,3,3,3,3,3,4),(-1.53373699248756,-1.47747305975871,-1.39029021397083,
-1.35774868938916,-1.33203786420062,-1.23038977040391,-1.19146538006595,
-1.16614143986796,-1.1287416766072,-1.02618547124656,-0.922698333606641,
-0.889977710189035,-0.867418444292481,-0.765890607100357,-0.67180537271053,
-0.617798901068506,-0.584547425353373,-0.476585692119078,-0.389549669541049,
-0.338521028541637,-0.310950996513903,-0.288719229766344,-0.179543753119938,
-0.0694757010746949,0.),.UNSPECIFIED.);
#1286=B_SPLINE_CURVE_WITH_KNOTS('',3,(#51207,#51208,#51209,#51210,#51211,
#51212,#51213,#51214,#51215,#51216,#51217,#51218,#51219,#51220,#51221,#51222,
#51223,#51224,#51225,#51226,#51227,#51228,#51229,#51230,#51231,#51232,#51233,
#51234,#51235,#51236,#51237,#51238,#51239,#51240,#51241,#51242,#51243,#51244,
#51245,#51246,#51247,#51248,#51249,#51250,#51251,#51252,#51253,#51254,#51255,
#51256,#51257,#51258,#51259,#51260,#51261,#51262,#51263,#51264,#51265,#51266,
#51267,#51268,#51269,#51270,#51271,#51272,#51273,#51274,#51275,#51276,#51277,
#51278,#51279,#51280,#51281,#51282),.UNSPECIFIED.,.F.,.F.,(4,3,3,3,3,3,
3,3,3,3,3,3,3,3,3,3,3,3,3,3,3,3,3,3,3,4),(-1.52870610664518,-1.46376476615558,
-1.36738223521408,-1.32958326055218,-1.30288468132391,-1.19055966185675,
-1.12214938319575,-1.0961569708181,-1.07823464238959,-0.971315082094603,
-0.865333221118986,-0.833428294780767,-0.811851541586676,-0.705424835001878,
-0.615550946694521,-0.567787651690986,-0.544829757697887,-0.521800305094042,
-0.419968998263115,-0.345929281772451,-0.297699082711072,-0.272424456165966,
-0.25356076098078,-0.153489816757136,-0.0552696732558858,0.),
 .UNSPECIFIED.);
#1287=B_SPLINE_CURVE_WITH_KNOTS('',3,(#52759,#52760,#52761,#52762,#52763,
#52764,#52765,#52766,#52767,#52768,#52769,#52770,#52771,#52772,#52773,#52774,
#52775,#52776,#52777,#52778,#52779,#52780),.UNSPECIFIED.,.F.,.F.,(4,3,3,
3,3,3,3,4),(177.052837307172,177.351505877399,177.849684264695,178.347862651991,
178.846041039287,179.344219426583,179.842397813879,180.258303277675),
 .UNSPECIFIED.);
#1288=B_SPLINE_CURVE_WITH_KNOTS('',3,(#52782,#52783,#52784,#52785,#52786,
#52787,#52788,#52789,#52790,#52791,#52792,#52793,#52794,#52795,#52796,#52797,
#52798,#52799,#52800,#52801,#52802,#52803,#52804,#52805,#52806,#52807,#52808,
#52809,#52810,#52811,#52812,#52813,#52814,#52815,#52816,#52817,#52818,#52819,
#52820,#52821,#52822,#52823,#52824,#52825,#52826,#52827,#52828,#52829,#52830,
#52831,#52832,#52833,#52834,#52835,#52836,#52837,#52838,#52839,#52840,#52841,
#52842,#52843,#52844,#52845,#52846,#52847,#52848,#52849,#52850,#52851,#52852,
#52853,#52854),.UNSPECIFIED.,.F.,.F.,(4,3,3,3,3,3,3,3,3,3,3,3,3,3,3,3,3,
3,3,3,3,3,3,3,4),(-1.53373699248745,-1.47747305975858,-1.39029021397072,
-1.35774869265005,-1.3320378699845,-1.23038977329582,-1.19146538262761,
-1.16614144091151,-1.12874167660715,-1.02618546806066,-0.922698329608141,
-0.889977692654673,-0.86741844172116,-0.765890607100252,-0.671805372710442,
-0.61779890472176,-0.584547424585698,-0.476585688325599,-0.389549669541011,
-0.338521026353068,-0.310950992013572,-0.28871922610837,-0.179543774302306,
-0.0694757077851898,0.),.UNSPECIFIED.);
#1289=B_SPLINE_CURVE_WITH_KNOTS('',3,(#52855,#52856,#52857,#52858,#52859,
#52860,#52861,#52862,#52863,#52864,#52865,#52866,#52867,#52868),
 .UNSPECIFIED.,.F.,.F.,(4,1,1,1,1,1,1,1,1,1,1,4),(10.3761157273103,10.7920211911067,
11.2901995784027,11.7883779656988,12.2865563529949,12.7847347402909,13.282913127587,
13.781091514883,14.2792699021791,14.7774482894752,15.2756266767712,15.707963267949),
 .UNSPECIFIED.);
#1290=B_SPLINE_CURVE_WITH_KNOTS('',3,(#52874,#52875,#52876,#52877,#52878,
#52879,#52880,#52881,#52882,#52883,#52884,#52885,#52886,#52887,#52888,#52889,
#52890,#52891,#52892,#52893,#52894,#52895,#52896,#52897,#52898,#52899,#52900,
#52901,#52902,#52903,#52904,#52905,#52906,#52907,#52908,#52909,#52910,#52911,
#52912,#52913,#52914,#52915,#52916,#52917,#52918,#52919,#52920,#52921,#52922,
#52923,#52924,#52925,#52926,#52927,#52928,#52929,#52930,#52931,#52932,#52933,
#52934,#52935,#52936,#52937,#52938,#52939,#52940,#52941,#52942,#52943,#52944,
#52945,#52946,#52947,#52948,#52949),.UNSPECIFIED.,.F.,.F.,(4,3,3,3,3,3,
3,3,3,3,3,3,3,3,3,3,3,3,3,3,3,3,3,3,3,4),(-1.52870610664516,-1.46376476615555,
-1.36738223521406,-1.32958325854658,-1.30288467919751,-1.19055966079354,
-1.12214938313862,-1.09615697088941,-1.07823464238957,-0.971315084120084,
-0.865333237336496,-0.833428218151789,-0.81185148451087,-0.705424835001883,
-0.615550946694523,-0.567787650900965,-0.544829752438311,-0.521800302803709,
-0.419968974496642,-0.345929281772446,-0.297699074379986,-0.272424429856221,
-0.253560731563668,-0.153489786788608,-0.0552696831557091,0.),
 .UNSPECIFIED.);
#1291=B_SPLINE_CURVE_WITH_KNOTS('',3,(#52952,#52953,#52954,#52955,#52956,
#52957,#52958,#52959,#52960,#52961,#52962,#52963),.UNSPECIFIED.,.F.,.F.,
(4,1,1,1,1,1,1,1,1,4),(11.6150328478184,12.1132112351144,12.6113896224105,
13.1095680097066,13.6077463970026,14.1059247842987,14.6041031715948,15.1022815588908,
15.6004599461869,15.707963267949),.UNSPECIFIED.);
#1292=B_SPLINE_CURVE_WITH_KNOTS('',3,(#54440,#54441,#54442,#54443,#54444,
#54445,#54446,#54447,#54448,#54449,#54450,#54451,#54452,#54453,#54454,#54455),
 .UNSPECIFIED.,.F.,.F.,(4,3,3,3,3,4),(-182.333289750359,-181.835111363063,
-181.336932975767,-180.838754588471,-180.340576201175,-180.022119021159),
 .UNSPECIFIED.);
#1835=PLANE('',#27609);
#1836=PLANE('',#27612);
#1837=PLANE('',#27617);
#1838=PLANE('',#27619);
#1839=PLANE('',#27621);
#1840=PLANE('',#27623);
#1841=PLANE('',#27625);
#1842=PLANE('',#27627);
#1843=PLANE('',#27637);
#1844=PLANE('',#27638);
#1845=PLANE('',#27639);
#1846=PLANE('',#27640);
#1847=PLANE('',#27641);
#1848=PLANE('',#27642);
#1849=PLANE('',#27643);
#1850=PLANE('',#27644);
#1851=PLANE('',#27645);
#1852=PLANE('',#27646);
#1853=PLANE('',#27647);
#1854=PLANE('',#27648);
#1855=PLANE('',#27649);
#1856=PLANE('',#27650);
#1857=PLANE('',#27651);
#1858=PLANE('',#27652);
#1859=PLANE('',#27653);
#1860=PLANE('',#27654);
#1861=PLANE('',#27655);
#1862=PLANE('',#27656);
#1863=PLANE('',#27657);
#1864=PLANE('',#27658);
#1865=PLANE('',#27659);
#1866=PLANE('',#27660);
#1867=PLANE('',#27661);
#1868=PLANE('',#27668);
#2912=FACE_OUTER_BOUND('',#4420,.T.);
#2913=FACE_OUTER_BOUND('',#4421,.T.);
#2914=FACE_OUTER_BOUND('',#4422,.T.);
#2915=FACE_OUTER_BOUND('',#4423,.T.);
#2916=FACE_OUTER_BOUND('',#4424,.T.);
#2917=FACE_OUTER_BOUND('',#4425,.T.);
#2918=FACE_OUTER_BOUND('',#4426,.T.);
#2919=FACE_OUTER_BOUND('',#4427,.T.);
#2920=FACE_OUTER_BOUND('',#4428,.T.);
#2921=FACE_OUTER_BOUND('',#4429,.T.);
#2922=FACE_OUTER_BOUND('',#4430,.T.);
#2923=FACE_OUTER_BOUND('',#4431,.T.);
#2924=FACE_OUTER_BOUND('',#4432,.T.);
#2925=FACE_OUTER_BOUND('',#4433,.T.);
#2926=FACE_OUTER_BOUND('',#4434,.T.);
#2927=FACE_OUTER_BOUND('',#4435,.T.);
#2928=FACE_OUTER_BOUND('',#4436,.T.);
#2929=FACE_OUTER_BOUND('',#4437,.T.);
#2930=FACE_OUTER_BOUND('',#4438,.T.);
#2931=FACE_OUTER_BOUND('',#4439,.T.);
#2932=FACE_OUTER_BOUND('',#4440,.T.);
#2933=FACE_OUTER_BOUND('',#4441,.T.);
#2934=FACE_OUTER_BOUND('',#4442,.T.);
#2935=FACE_OUTER_BOUND('',#4443,.T.);
#2936=FACE_OUTER_BOUND('',#4444,.T.);
#2937=FACE_OUTER_BOUND('',#4445,.T.);
#2938=FACE_OUTER_BOUND('',#4446,.T.);
#2939=FACE_OUTER_BOUND('',#4447,.T.);
#2940=FACE_OUTER_BOUND('',#4448,.T.);
#2941=FACE_OUTER_BOUND('',#4449,.T.);
#2942=FACE_OUTER_BOUND('',#4450,.T.);
#2943=FACE_OUTER_BOUND('',#4451,.T.);
#2944=FACE_OUTER_BOUND('',#4452,.T.);
#2945=FACE_OUTER_BOUND('',#4453,.T.);
#2946=FACE_OUTER_BOUND('',#4454,.T.);
#2947=FACE_OUTER_BOUND('',#4455,.T.);
#2948=FACE_OUTER_BOUND('',#4456,.T.);
#2949=FACE_OUTER_BOUND('',#4457,.T.);
#2950=FACE_OUTER_BOUND('',#4458,.T.);
#2951=FACE_OUTER_BOUND('',#4459,.T.);
#2952=FACE_OUTER_BOUND('',#4460,.T.);
#2953=FACE_OUTER_BOUND('',#4461,.T.);
#2954=FACE_OUTER_BOUND('',#4462,.T.);
#2955=FACE_OUTER_BOUND('',#4463,.T.);
#2956=FACE_OUTER_BOUND('',#4464,.T.);
#2957=FACE_OUTER_BOUND('',#4465,.T.);
#2958=FACE_OUTER_BOUND('',#4466,.T.);
#2959=FACE_OUTER_BOUND('',#4467,.T.);
#2960=FACE_OUTER_BOUND('',#4468,.T.);
#2961=FACE_OUTER_BOUND('',#4469,.T.);
#2962=FACE_OUTER_BOUND('',#4470,.T.);
#2963=FACE_OUTER_BOUND('',#4471,.T.);
#2964=FACE_OUTER_BOUND('',#4472,.T.);
#2965=FACE_OUTER_BOUND('',#4473,.T.);
#2966=FACE_OUTER_BOUND('',#4474,.T.);
#2967=FACE_OUTER_BOUND('',#4475,.T.);
#2968=FACE_OUTER_BOUND('',#4476,.T.);
#2969=FACE_OUTER_BOUND('',#4477,.T.);
#2970=FACE_OUTER_BOUND('',#4478,.T.);
#2971=FACE_OUTER_BOUND('',#4479,.T.);
#2972=FACE_OUTER_BOUND('',#4480,.T.);
#2973=FACE_OUTER_BOUND('',#4481,.T.);
#2974=FACE_OUTER_BOUND('',#4482,.T.);
#2975=FACE_OUTER_BOUND('',#4483,.T.);
#2976=FACE_OUTER_BOUND('',#4484,.T.);
#2977=FACE_OUTER_BOUND('',#4485,.T.);
#2978=FACE_OUTER_BOUND('',#4486,.T.);
#2979=FACE_OUTER_BOUND('',#4487,.T.);
#2980=FACE_OUTER_BOUND('',#4488,.T.);
#2981=FACE_OUTER_BOUND('',#4489,.T.);
#2982=FACE_OUTER_BOUND('',#4490,.T.);
#2983=FACE_OUTER_BOUND('',#4491,.T.);
#2984=FACE_OUTER_BOUND('',#4492,.T.);
#2985=FACE_OUTER_BOUND('',#4493,.T.);
#2986=FACE_OUTER_BOUND('',#4494,.T.);
#2987=FACE_OUTER_BOUND('',#4495,.T.);
#2988=FACE_OUTER_BOUND('',#4496,.T.);
#2989=FACE_OUTER_BOUND('',#4497,.T.);
#2990=FACE_OUTER_BOUND('',#4498,.T.);
#2991=FACE_OUTER_BOUND('',#4499,.T.);
#2992=FACE_OUTER_BOUND('',#4500,.T.);
#2993=FACE_OUTER_BOUND('',#4501,.T.);
#2994=FACE_OUTER_BOUND('',#4502,.T.);
#2995=FACE_OUTER_BOUND('',#4503,.T.);
#2996=FACE_OUTER_BOUND('',#4504,.T.);
#2997=FACE_OUTER_BOUND('',#4505,.T.);
#2998=FACE_OUTER_BOUND('',#4506,.T.);
#2999=FACE_OUTER_BOUND('',#4507,.T.);
#3000=FACE_OUTER_BOUND('',#4508,.T.);
#3001=FACE_OUTER_BOUND('',#4509,.T.);
#3002=FACE_OUTER_BOUND('',#4510,.T.);
#3003=FACE_OUTER_BOUND('',#4511,.T.);
#3004=FACE_OUTER_BOUND('',#4512,.T.);
#3005=FACE_OUTER_BOUND('',#4513,.T.);
#3006=FACE_OUTER_BOUND('',#4514,.T.);
#3007=FACE_OUTER_BOUND('',#4515,.T.);
#3008=FACE_OUTER_BOUND('',#4516,.T.);
#3009=FACE_OUTER_BOUND('',#4517,.T.);
#3010=FACE_OUTER_BOUND('',#4518,.T.);
#4420=EDGE_LOOP('',(#19282,#19283,#19284,#19285));
#4421=EDGE_LOOP('',(#19286,#19287,#19288,#19289));
#4422=EDGE_LOOP('',(#19290,#19291,#19292,#19293));
#4423=EDGE_LOOP('',(#19294,#19295,#19296,#19297));
#4424=EDGE_LOOP('',(#19298,#19299,#19300,#19301));
#4425=EDGE_LOOP('',(#19302,#19303,#19304,#19305));
#4426=EDGE_LOOP('',(#19306,#19307,#19308,#19309));
#4427=EDGE_LOOP('',(#19310,#19311,#19312,#19313));
#4428=EDGE_LOOP('',(#19314,#19315,#19316,#19317));
#4429=EDGE_LOOP('',(#19318,#19319,#19320,#19321));
#4430=EDGE_LOOP('',(#19322,#19323,#19324,#19325));
#4431=EDGE_LOOP('',(#19326,#19327,#19328,#19329));
#4432=EDGE_LOOP('',(#19330,#19331,#19332,#19333));
#4433=EDGE_LOOP('',(#19334,#19335,#19336,#19337));
#4434=EDGE_LOOP('',(#19338,#19339,#19340,#19341));
#4435=EDGE_LOOP('',(#19342,#19343,#19344,#19345));
#4436=EDGE_LOOP('',(#19346,#19347,#19348,#19349));
#4437=EDGE_LOOP('',(#19350,#19351,#19352,#19353));
#4438=EDGE_LOOP('',(#19354,#19355,#19356,#19357));
#4439=EDGE_LOOP('',(#19358,#19359,#19360,#19361));
#4440=EDGE_LOOP('',(#19362,#19363,#19364,#19365));
#4441=EDGE_LOOP('',(#19366,#19367,#19368,#19369));
#4442=EDGE_LOOP('',(#19370,#19371,#19372,#19373));
#4443=EDGE_LOOP('',(#19374,#19375,#19376,#19377));
#4444=EDGE_LOOP('',(#19378,#19379,#19380,#19381));
#4445=EDGE_LOOP('',(#19382,#19383,#19384,#19385));
#4446=EDGE_LOOP('',(#19386,#19387,#19388,#19389));
#4447=EDGE_LOOP('',(#19390,#19391,#19392,#19393));
#4448=EDGE_LOOP('',(#19394,#19395,#19396,#19397));
#4449=EDGE_LOOP('',(#19398,#19399,#19400));
#4450=EDGE_LOOP('',(#19401,#19402,#19403,#19404,#19405));
#4451=EDGE_LOOP('',(#19406,#19407,#19408,#19409));
#4452=EDGE_LOOP('',(#19410,#19411,#19412,#19413));
#4453=EDGE_LOOP('',(#19414,#19415,#19416,#19417));
#4454=EDGE_LOOP('',(#19418,#19419,#19420,#19421));
#4455=EDGE_LOOP('',(#19422,#19423,#19424,#19425));
#4456=EDGE_LOOP('',(#19426,#19427,#19428,#19429));
#4457=EDGE_LOOP('',(#19430,#19431,#19432,#19433));
#4458=EDGE_LOOP('',(#19434,#19435,#19436,#19437));
#4459=EDGE_LOOP('',(#19438,#19439,#19440,#19441));
#4460=EDGE_LOOP('',(#19442,#19443,#19444,#19445));
#4461=EDGE_LOOP('',(#19446,#19447,#19448,#19449));
#4462=EDGE_LOOP('',(#19450,#19451,#19452,#19453));
#4463=EDGE_LOOP('',(#19454,#19455,#19456,#19457));
#4464=EDGE_LOOP('',(#19458,#19459,#19460,#19461));
#4465=EDGE_LOOP('',(#19462,#19463,#19464,#19465));
#4466=EDGE_LOOP('',(#19466,#19467,#19468,#19469));
#4467=EDGE_LOOP('',(#19470,#19471,#19472,#19473));
#4468=EDGE_LOOP('',(#19474,#19475,#19476,#19477));
#4469=EDGE_LOOP('',(#19478,#19479,#19480,#19481));
#4470=EDGE_LOOP('',(#19482,#19483,#19484,#19485));
#4471=EDGE_LOOP('',(#19486,#19487,#19488,#19489));
#4472=EDGE_LOOP('',(#19490,#19491,#19492,#19493));
#4473=EDGE_LOOP('',(#19494,#19495,#19496,#19497));
#4474=EDGE_LOOP('',(#19498,#19499,#19500,#19501));
#4475=EDGE_LOOP('',(#19502,#19503,#19504,#19505));
#4476=EDGE_LOOP('',(#19506,#19507,#19508,#19509));
#4477=EDGE_LOOP('',(#19510,#19511,#19512,#19513));
#4478=EDGE_LOOP('',(#19514,#19515,#19516,#19517,#19518,#19519));
#4479=EDGE_LOOP('',(#19520,#19521,#19522,#19523,#19524,#19525,#19526,#19527,
#19528,#19529,#19530,#19531,#19532,#19533,#19534,#19535,#19536,#19537,#19538,
#19539,#19540,#19541,#19542,#19543,#19544,#19545,#19546,#19547,#19548,#19549,
#19550,#19551,#19552,#19553,#19554,#19555,#19556,#19557,#19558,#19559,#19560,
#19561,#19562,#19563,#19564,#19565,#19566,#19567,#19568,#19569,#19570,#19571,
#19572,#19573,#19574,#19575,#19576,#19577,#19578,#19579,#19580));
#4480=EDGE_LOOP('',(#19581,#19582,#19583,#19584,#19585));
#4481=EDGE_LOOP('',(#19586,#19587,#19588,#19589));
#4482=EDGE_LOOP('',(#19590,#19591,#19592,#19593,#19594,#19595,#19596,#19597,
#19598,#19599,#19600,#19601,#19602,#19603,#19604,#19605,#19606,#19607,#19608,
#19609,#19610,#19611,#19612,#19613,#19614,#19615,#19616,#19617,#19618,#19619,
#19620,#19621,#19622,#19623,#19624,#19625,#19626,#19627,#19628,#19629,#19630,
#19631,#19632,#19633,#19634,#19635,#19636,#19637,#19638,#19639,#19640,#19641,
#19642,#19643,#19644,#19645,#19646,#19647,#19648,#19649,#19650,#19651));
#4483=EDGE_LOOP('',(#19652,#19653));
#4484=EDGE_LOOP('',(#19654,#19655));
#4485=EDGE_LOOP('',(#19656,#19657));
#4486=EDGE_LOOP('',(#19658,#19659));
#4487=EDGE_LOOP('',(#19660,#19661));
#4488=EDGE_LOOP('',(#19662,#19663));
#4489=EDGE_LOOP('',(#19664,#19665,#19666,#19667,#19668,#19669,#19670,#19671,
#19672,#19673,#19674,#19675,#19676,#19677,#19678,#19679,#19680,#19681,#19682,
#19683,#19684,#19685,#19686,#19687,#19688,#19689,#19690));
#4490=EDGE_LOOP('',(#19691,#19692,#19693,#19694));
#4491=EDGE_LOOP('',(#19695,#19696,#19697));
#4492=EDGE_LOOP('',(#19698,#19699,#19700,#19701));
#4493=EDGE_LOOP('',(#19702,#19703,#19704));
#4494=EDGE_LOOP('',(#19705,#19706,#19707));
#4495=EDGE_LOOP('',(#19708,#19709,#19710,#19711));
#4496=EDGE_LOOP('',(#19712,#19713,#19714));
#4497=EDGE_LOOP('',(#19715,#19716,#19717,#19718));
#4498=EDGE_LOOP('',(#19719,#19720,#19721));
#4499=EDGE_LOOP('',(#19722,#19723,#19724));
#4500=EDGE_LOOP('',(#19725,#19726,#19727));
#4501=EDGE_LOOP('',(#19728,#19729,#19730));
#4502=EDGE_LOOP('',(#19731,#19732,#19733));
#4503=EDGE_LOOP('',(#19734,#19735,#19736));
#4504=EDGE_LOOP('',(#19737,#19738,#19739));
#4505=EDGE_LOOP('',(#19740,#19741,#19742,#19743));
#4506=EDGE_LOOP('',(#19744,#19745,#19746,#19747));
#4507=EDGE_LOOP('',(#19748,#19749,#19750));
#4508=EDGE_LOOP('',(#19751,#19752,#19753));
#4509=EDGE_LOOP('',(#19754,#19755,#19756));
#4510=EDGE_LOOP('',(#19757,#19758,#19759,#19760));
#4511=EDGE_LOOP('',(#19761,#19762,#19763));
#4512=EDGE_LOOP('',(#19764,#19765,#19766));
#4513=EDGE_LOOP('',(#19767,#19768,#19769));
#4514=EDGE_LOOP('',(#19770));
#4515=EDGE_LOOP('',(#19771,#19772,#19773,#19774,#19775,#19776));
#4516=EDGE_LOOP('',(#19777,#19778,#19779,#19780));
#4517=EDGE_LOOP('',(#19781,#19782,#19783,#19784,#19785,#19786));
#4518=EDGE_LOOP('',(#19787));
#4519=EDGE_LOOP('',(#19788,#19789,#19790,#19791,#19792,#19793));
#6049=LINE('',#47592,#8546);
#6050=LINE('',#47625,#8547);
#6051=LINE('',#47709,#8548);
#6052=LINE('',#47799,#8549);
#6053=LINE('',#47889,#8550);
#6054=LINE('',#47973,#8551);
#6055=LINE('',#48063,#8552);
#6056=LINE('',#48147,#8553);
#6057=LINE('',#48237,#8554);
#6058=LINE('',#48327,#8555);
#6059=LINE('',#48411,#8556);
#6060=LINE('',#48501,#8557);
#6061=LINE('',#48585,#8558);
#6062=LINE('',#48675,#8559);
#6063=LINE('',#48765,#8560);
#6064=LINE('',#48849,#8561);
#6065=LINE('',#48939,#8562);
#6066=LINE('',#49029,#8563);
#6067=LINE('',#49113,#8564);
#6068=LINE('',#49203,#8565);
#6069=LINE('',#49287,#8566);
#6070=LINE('',#49377,#8567);
#6071=LINE('',#49467,#8568);
#6072=LINE('',#49551,#8569);
#6073=LINE('',#49641,#8570);
#6074=LINE('',#49725,#8571);
#6075=LINE('',#49815,#8572);
#6076=LINE('',#49905,#8573);
#6077=LINE('',#49989,#8574);
#6078=LINE('',#50079,#8575);
#6079=LINE('',#50089,#8576);
#6080=LINE('',#50126,#8577);
#6081=LINE('',#50163,#8578);
#6082=LINE('',#50200,#8579);
#6083=LINE('',#50238,#8580);
#6084=LINE('',#50275,#8581);
#6085=LINE('',#50312,#8582);
#6086=LINE('',#50349,#8583);
#6087=LINE('',#50386,#8584);
#6088=LINE('',#50424,#8585);
#6089=LINE('',#50461,#8586);
#6090=LINE('',#50498,#8587);
#6091=LINE('',#50535,#8588);
#6092=LINE('',#50572,#8589);
#6093=LINE('',#50610,#8590);
#6094=LINE('',#50647,#8591);
#6095=LINE('',#50684,#8592);
#6096=LINE('',#50722,#8593);
#6097=LINE('',#50759,#8594);
#6098=LINE('',#50796,#8595);
#6099=LINE('',#50833,#8596);
#6100=LINE('',#50870,#8597);
#6101=LINE('',#50908,#8598);
#6102=LINE('',#50945,#8599);
#6103=LINE('',#50982,#8600);
#6104=LINE('',#51019,#8601);
#6105=LINE('',#51056,#8602);
#6106=LINE('',#51094,#8603);
#6107=LINE('',#54459,#8604);
#6108=LINE('',#54463,#8605);
#6109=LINE('',#54467,#8606);
#6110=LINE('',#54471,#8607);
#6111=LINE('',#54475,#8608);
#6112=LINE('',#54478,#8609);
#6113=LINE('',#54483,#8610);
#6114=LINE('',#54541,#8611);
#6115=LINE('',#54543,#8612);
#6116=LINE('',#54544,#8613);
#6117=LINE('',#54547,#8614);
#6118=LINE('',#54548,#8615);
#6119=LINE('',#54551,#8616);
#6120=LINE('',#54552,#8617);
#6121=LINE('',#54555,#8618);
#6122=LINE('',#54556,#8619);
#6123=LINE('',#54559,#8620);
#6124=LINE('',#54560,#8621);
#6125=LINE('',#54563,#8622);
#6126=LINE('',#54564,#8623);
#6127=LINE('',#54567,#8624);
#6128=LINE('',#54568,#8625);
#6129=LINE('',#54571,#8626);
#6130=LINE('',#54572,#8627);
#6131=LINE('',#54575,#8628);
#6132=LINE('',#54576,#8629);
#6133=LINE('',#54578,#8630);
#6134=LINE('',#54580,#8631);
#6135=LINE('',#54583,#8632);
#6136=LINE('',#54586,#8633);
#6137=LINE('',#54587,#8634);
#6138=LINE('',#54589,#8635);
#6139=LINE('',#54591,#8636);
#6140=LINE('',#54594,#8637);
#6141=LINE('',#54595,#8638);
#6142=LINE('',#54597,#8639);
#6143=LINE('',#54601,#8640);
#6144=LINE('',#54609,#8641);
#6145=LINE('',#54615,#8642);
#8546=VECTOR('',#30396,0.8);
#8547=VECTOR('',#30401,0.8);
#8548=VECTOR('',#30404,0.8);
#8549=VECTOR('',#30407,0.8);
#8550=VECTOR('',#30410,0.8);
#8551=VECTOR('',#30413,0.8);
#8552=VECTOR('',#30416,0.8);
#8553=VECTOR('',#30419,0.8);
#8554=VECTOR('',#30422,0.8);
#8555=VECTOR('',#30425,0.8);
#8556=VECTOR('',#30428,0.8);
#8557=VECTOR('',#30431,0.8);
#8558=VECTOR('',#30434,0.8);
#8559=VECTOR('',#30437,0.8);
#8560=VECTOR('',#30440,0.8);
#8561=VECTOR('',#30443,0.8);
#8562=VECTOR('',#30446,0.8);
#8563=VECTOR('',#30449,0.8);
#8564=VECTOR('',#30452,0.8);
#8565=VECTOR('',#30455,0.8);
#8566=VECTOR('',#30458,0.8);
#8567=VECTOR('',#30461,0.8);
#8568=VECTOR('',#30464,0.8);
#8569=VECTOR('',#30467,0.8);
#8570=VECTOR('',#30470,0.8);
#8571=VECTOR('',#30473,0.8);
#8572=VECTOR('',#30476,0.8);
#8573=VECTOR('',#30479,0.8);
#8574=VECTOR('',#30482,0.8);
#8575=VECTOR('',#30485,0.6767);
#8576=VECTOR('',#30490,0.6767);
#8577=VECTOR('',#30495,0.6767);
#8578=VECTOR('',#30498,0.6767);
#8579=VECTOR('',#30501,0.6767);
#8580=VECTOR('',#30504,0.6767);
#8581=VECTOR('',#30507,0.6767);
#8582=VECTOR('',#30510,0.6767);
#8583=VECTOR('',#30513,0.6767);
#8584=VECTOR('',#30516,0.6767);
#8585=VECTOR('',#30519,0.6767);
#8586=VECTOR('',#30522,0.6767);
#8587=VECTOR('',#30525,0.6767);
#8588=VECTOR('',#30528,0.6767);
#8589=VECTOR('',#30531,0.6767);
#8590=VECTOR('',#30534,0.6767);
#8591=VECTOR('',#30537,0.6767);
#8592=VECTOR('',#30540,0.6767);
#8593=VECTOR('',#30543,0.6767);
#8594=VECTOR('',#30546,0.6767);
#8595=VECTOR('',#30549,0.6767);
#8596=VECTOR('',#30552,0.6767);
#8597=VECTOR('',#30555,0.6767);
#8598=VECTOR('',#30558,0.6767);
#8599=VECTOR('',#30561,0.6767);
#8600=VECTOR('',#30564,0.6767);
#8601=VECTOR('',#30567,0.6767);
#8602=VECTOR('',#30570,0.6767);
#8603=VECTOR('',#30573,0.6767);
#8604=VECTOR('',#30592,1.);
#8605=VECTOR('',#30597,1.);
#8606=VECTOR('',#30602,1.);
#8607=VECTOR('',#30607,1.);
#8608=VECTOR('',#30612,1.);
#8609=VECTOR('',#30617,1.);
#8610=VECTOR('',#30622,0.23094010767585);
#8611=VECTOR('',#30639,1.);
#8612=VECTOR('',#30640,1.);
#8613=VECTOR('',#30641,1.);
#8614=VECTOR('',#30644,1.);
#8615=VECTOR('',#30645,1.);
#8616=VECTOR('',#30648,1.);
#8617=VECTOR('',#30649,1.);
#8618=VECTOR('',#30652,1.);
#8619=VECTOR('',#30653,1.);
#8620=VECTOR('',#30656,1.);
#8621=VECTOR('',#30657,1.);
#8622=VECTOR('',#30660,1.);
#8623=VECTOR('',#30661,1.);
#8624=VECTOR('',#30664,1.);
#8625=VECTOR('',#30665,1.);
#8626=VECTOR('',#30668,1.);
#8627=VECTOR('',#30669,1.);
#8628=VECTOR('',#30672,1.);
#8629=VECTOR('',#30673,1.);
#8630=VECTOR('',#30676,1.);
#8631=VECTOR('',#30679,1.);
#8632=VECTOR('',#30684,1.);
#8633=VECTOR('',#30687,1.);
#8634=VECTOR('',#30688,1.);
#8635=VECTOR('',#30691,1.);
#8636=VECTOR('',#30694,1.);
#8637=VECTOR('',#30697,1.);
#8638=VECTOR('',#30698,1.);
#8639=VECTOR('',#30701,1.);
#8640=VECTOR('',#30708,1.);
#8641=VECTOR('',#30721,0.7);
#8642=VECTOR('',#30730,0.76);
#10810=CIRCLE('',#27549,0.7911);
#10811=CIRCLE('',#27579,0.6767);
#10812=CIRCLE('',#27581,0.6767);
#10813=CIRCLE('',#27610,0.7911);
#10814=CIRCLE('',#27611,0.7911);
#10815=CIRCLE('',#27613,0.7911);
#10816=CIRCLE('',#27614,0.7911);
#10817=CIRCLE('',#27615,0.6767);
#10818=CIRCLE('',#27618,0.461880215351701);
#10819=CIRCLE('',#27620,0.461880215351701);
#10820=CIRCLE('',#27622,0.461880215351701);
#10821=CIRCLE('',#27624,0.461880215351701);
#10822=CIRCLE('',#27626,0.461880215351701);
#10823=CIRCLE('',#27628,0.461880215351701);
#10824=CIRCLE('',#27630,0.460219541126976);
#10825=CIRCLE('',#27631,0.460219541126976);
#10826=CIRCLE('',#27632,0.460219541126976);
#10827=CIRCLE('',#27633,0.460219541126976);
#10828=CIRCLE('',#27634,0.460219541126976);
#10829=CIRCLE('',#27635,0.460219541126976);
#10830=CIRCLE('',#27636,0.460219541126976);
#10831=CIRCLE('',#27662,0.6);
#10832=CIRCLE('',#27665,0.7911);
#10833=CIRCLE('',#27667,0.72);
#11704=VERTEX_POINT('',#47590);
#11705=VERTEX_POINT('',#47591);
#11706=VERTEX_POINT('',#47593);
#11707=VERTEX_POINT('',#47610);
#11708=VERTEX_POINT('',#47623);
#11709=VERTEX_POINT('',#47624);
#11710=VERTEX_POINT('',#47707);
#11711=VERTEX_POINT('',#47708);
#11712=VERTEX_POINT('',#47797);
#11713=VERTEX_POINT('',#47798);
#11714=VERTEX_POINT('',#47887);
#11715=VERTEX_POINT('',#47888);
#11716=VERTEX_POINT('',#47971);
#11717=VERTEX_POINT('',#47972);
#11718=VERTEX_POINT('',#48061);
#11719=VERTEX_POINT('',#48062);
#11720=VERTEX_POINT('',#48145);
#11721=VERTEX_POINT('',#48146);
#11722=VERTEX_POINT('',#48235);
#11723=VERTEX_POINT('',#48236);
#11724=VERTEX_POINT('',#48325);
#11725=VERTEX_POINT('',#48326);
#11726=VERTEX_POINT('',#48409);
#11727=VERTEX_POINT('',#48410);
#11728=VERTEX_POINT('',#48499);
#11729=VERTEX_POINT('',#48500);
#11730=VERTEX_POINT('',#48583);
#11731=VERTEX_POINT('',#48584);
#11732=VERTEX_POINT('',#48673);
#11733=VERTEX_POINT('',#48674);
#11734=VERTEX_POINT('',#48763);
#11735=VERTEX_POINT('',#48764);
#11736=VERTEX_POINT('',#48847);
#11737=VERTEX_POINT('',#48848);
#11738=VERTEX_POINT('',#48937);
#11739=VERTEX_POINT('',#48938);
#11740=VERTEX_POINT('',#49027);
#11741=VERTEX_POINT('',#49028);
#11742=VERTEX_POINT('',#49111);
#11743=VERTEX_POINT('',#49112);
#11744=VERTEX_POINT('',#49201);
#11745=VERTEX_POINT('',#49202);
#11746=VERTEX_POINT('',#49285);
#11747=VERTEX_POINT('',#49286);
#11748=VERTEX_POINT('',#49375);
#11749=VERTEX_POINT('',#49376);
#11750=VERTEX_POINT('',#49465);
#11751=VERTEX_POINT('',#49466);
#11752=VERTEX_POINT('',#49549);
#11753=VERTEX_POINT('',#49550);
#11754=VERTEX_POINT('',#49639);
#11755=VERTEX_POINT('',#49640);
#11756=VERTEX_POINT('',#49723);
#11757=VERTEX_POINT('',#49724);
#11758=VERTEX_POINT('',#49813);
#11759=VERTEX_POINT('',#49814);
#11760=VERTEX_POINT('',#49903);
#11761=VERTEX_POINT('',#49904);
#11762=VERTEX_POINT('',#49987);
#11763=VERTEX_POINT('',#49988);
#11764=VERTEX_POINT('',#50077);
#11765=VERTEX_POINT('',#50078);
#11766=VERTEX_POINT('',#50080);
#11767=VERTEX_POINT('',#50087);
#11768=VERTEX_POINT('',#50088);
#11769=VERTEX_POINT('',#50107);
#11770=VERTEX_POINT('',#50124);
#11771=VERTEX_POINT('',#50125);
#11772=VERTEX_POINT('',#50161);
#11773=VERTEX_POINT('',#50162);
#11774=VERTEX_POINT('',#50198);
#11775=VERTEX_POINT('',#50199);
#11776=VERTEX_POINT('',#50236);
#11777=VERTEX_POINT('',#50237);
#11778=VERTEX_POINT('',#50273);
#11779=VERTEX_POINT('',#50274);
#11780=VERTEX_POINT('',#50310);
#11781=VERTEX_POINT('',#50311);
#11782=VERTEX_POINT('',#50347);
#11783=VERTEX_POINT('',#50348);
#11784=VERTEX_POINT('',#50384);
#11785=VERTEX_POINT('',#50385);
#11786=VERTEX_POINT('',#50422);
#11787=VERTEX_POINT('',#50423);
#11788=VERTEX_POINT('',#50459);
#11789=VERTEX_POINT('',#50460);
#11790=VERTEX_POINT('',#50496);
#11791=VERTEX_POINT('',#50497);
#11792=VERTEX_POINT('',#50533);
#11793=VERTEX_POINT('',#50534);
#11794=VERTEX_POINT('',#50570);
#11795=VERTEX_POINT('',#50571);
#11796=VERTEX_POINT('',#50608);
#11797=VERTEX_POINT('',#50609);
#11798=VERTEX_POINT('',#50645);
#11799=VERTEX_POINT('',#50646);
#11800=VERTEX_POINT('',#50682);
#11801=VERTEX_POINT('',#50683);
#11802=VERTEX_POINT('',#50720);
#11803=VERTEX_POINT('',#50721);
#11804=VERTEX_POINT('',#50757);
#11805=VERTEX_POINT('',#50758);
#11806=VERTEX_POINT('',#50794);
#11807=VERTEX_POINT('',#50795);
#11808=VERTEX_POINT('',#50831);
#11809=VERTEX_POINT('',#50832);
#11810=VERTEX_POINT('',#50868);
#11811=VERTEX_POINT('',#50869);
#11812=VERTEX_POINT('',#50906);
#11813=VERTEX_POINT('',#50907);
#11814=VERTEX_POINT('',#50943);
#11815=VERTEX_POINT('',#50944);
#11816=VERTEX_POINT('',#50980);
#11817=VERTEX_POINT('',#50981);
#11818=VERTEX_POINT('',#51017);
#11819=VERTEX_POINT('',#51018);
#11820=VERTEX_POINT('',#51054);
#11821=VERTEX_POINT('',#51055);
#11822=VERTEX_POINT('',#51092);
#11823=VERTEX_POINT('',#51093);
#11824=VERTEX_POINT('',#51129);
#11825=VERTEX_POINT('',#51203);
#11826=VERTEX_POINT('',#51205);
#11827=VERTEX_POINT('',#52781);
#11828=VERTEX_POINT('',#52870);
#11829=VERTEX_POINT('',#52873);
#11830=VERTEX_POINT('',#54457);
#11831=VERTEX_POINT('',#54458);
#11832=VERTEX_POINT('',#54462);
#11833=VERTEX_POINT('',#54466);
#11834=VERTEX_POINT('',#54470);
#11835=VERTEX_POINT('',#54474);
#11836=VERTEX_POINT('',#54481);
#11837=VERTEX_POINT('',#54482);
#11838=VERTEX_POINT('',#54484);
#11839=VERTEX_POINT('',#54489);
#11840=VERTEX_POINT('',#54493);
#11841=VERTEX_POINT('',#54498);
#11842=VERTEX_POINT('',#54502);
#11843=VERTEX_POINT('',#54507);
#11844=VERTEX_POINT('',#54511);
#11845=VERTEX_POINT('',#54516);
#11846=VERTEX_POINT('',#54520);
#11847=VERTEX_POINT('',#54525);
#11848=VERTEX_POINT('',#54529);
#11849=VERTEX_POINT('',#54534);
#11850=VERTEX_POINT('',#54540);
#11851=VERTEX_POINT('',#54542);
#11852=VERTEX_POINT('',#54546);
#11853=VERTEX_POINT('',#54550);
#11854=VERTEX_POINT('',#54554);
#11855=VERTEX_POINT('',#54558);
#11856=VERTEX_POINT('',#54562);
#11857=VERTEX_POINT('',#54566);
#11858=VERTEX_POINT('',#54570);
#11859=VERTEX_POINT('',#54574);
#11860=VERTEX_POINT('',#54585);
#11861=VERTEX_POINT('',#54593);
#11862=VERTEX_POINT('',#54606);
#11863=VERTEX_POINT('',#54613);
#14494=EDGE_CURVE('',#11704,#11705,#6049,.T.);
#14495=EDGE_CURVE('',#11704,#11706,#1170,.T.);
#14496=EDGE_CURVE('',#11706,#11707,#10810,.T.);
#14497=EDGE_CURVE('',#11707,#11705,#1171,.T.);
#14498=EDGE_CURVE('',#11708,#11709,#6050,.T.);
#14499=EDGE_CURVE('',#11708,#11704,#1172,.T.);
#14500=EDGE_CURVE('',#11705,#11709,#1173,.T.);
#14501=EDGE_CURVE('',#11710,#11711,#6051,.T.);
#14502=EDGE_CURVE('',#11710,#11708,#1174,.T.);
#14503=EDGE_CURVE('',#11709,#11711,#1175,.T.);
#14504=EDGE_CURVE('',#11712,#11713,#6052,.T.);
#14505=EDGE_CURVE('',#11712,#11710,#1176,.T.);
#14506=EDGE_CURVE('',#11711,#11713,#1177,.T.);
#14507=EDGE_CURVE('',#11714,#11715,#6053,.T.);
#14508=EDGE_CURVE('',#11714,#11712,#1178,.T.);
#14509=EDGE_CURVE('',#11713,#11715,#1179,.T.);
#14510=EDGE_CURVE('',#11716,#11717,#6054,.T.);
#14511=EDGE_CURVE('',#11716,#11714,#1180,.T.);
#14512=EDGE_CURVE('',#11715,#11717,#1181,.T.);
#14513=EDGE_CURVE('',#11718,#11719,#6055,.T.);
#14514=EDGE_CURVE('',#11718,#11716,#1182,.T.);
#14515=EDGE_CURVE('',#11717,#11719,#1183,.T.);
#14516=EDGE_CURVE('',#11720,#11721,#6056,.T.);
#14517=EDGE_CURVE('',#11720,#11718,#1184,.T.);
#14518=EDGE_CURVE('',#11719,#11721,#1185,.T.);
#14519=EDGE_CURVE('',#11722,#11723,#6057,.T.);
#14520=EDGE_CURVE('',#11722,#11720,#1186,.T.);
#14521=EDGE_CURVE('',#11721,#11723,#1187,.T.);
#14522=EDGE_CURVE('',#11724,#11725,#6058,.T.);
#14523=EDGE_CURVE('',#11724,#11722,#1188,.T.);
#14524=EDGE_CURVE('',#11723,#11725,#1189,.T.);
#14525=EDGE_CURVE('',#11726,#11727,#6059,.T.);
#14526=EDGE_CURVE('',#11726,#11724,#1190,.T.);
#14527=EDGE_CURVE('',#11725,#11727,#1191,.T.);
#14528=EDGE_CURVE('',#11728,#11729,#6060,.T.);
#14529=EDGE_CURVE('',#11728,#11726,#1192,.T.);
#14530=EDGE_CURVE('',#11727,#11729,#1193,.T.);
#14531=EDGE_CURVE('',#11730,#11731,#6061,.T.);
#14532=EDGE_CURVE('',#11730,#11728,#1194,.T.);
#14533=EDGE_CURVE('',#11729,#11731,#1195,.T.);
#14534=EDGE_CURVE('',#11732,#11733,#6062,.T.);
#14535=EDGE_CURVE('',#11732,#11730,#1196,.T.);
#14536=EDGE_CURVE('',#11731,#11733,#1197,.T.);
#14537=EDGE_CURVE('',#11734,#11735,#6063,.T.);
#14538=EDGE_CURVE('',#11734,#11732,#1198,.T.);
#14539=EDGE_CURVE('',#11733,#11735,#1199,.T.);
#14540=EDGE_CURVE('',#11736,#11737,#6064,.T.);
#14541=EDGE_CURVE('',#11736,#11734,#1200,.T.);
#14542=EDGE_CURVE('',#11735,#11737,#1201,.T.);
#14543=EDGE_CURVE('',#11738,#11739,#6065,.T.);
#14544=EDGE_CURVE('',#11738,#11736,#1202,.T.);
#14545=EDGE_CURVE('',#11737,#11739,#1203,.T.);
#14546=EDGE_CURVE('',#11740,#11741,#6066,.T.);
#14547=EDGE_CURVE('',#11740,#11738,#1204,.T.);
#14548=EDGE_CURVE('',#11739,#11741,#1205,.T.);
#14549=EDGE_CURVE('',#11742,#11743,#6067,.T.);
#14550=EDGE_CURVE('',#11742,#11740,#1206,.T.);
#14551=EDGE_CURVE('',#11741,#11743,#1207,.T.);
#14552=EDGE_CURVE('',#11744,#11745,#6068,.T.);
#14553=EDGE_CURVE('',#11744,#11742,#1208,.T.);
#14554=EDGE_CURVE('',#11743,#11745,#1209,.T.);
#14555=EDGE_CURVE('',#11746,#11747,#6069,.T.);
#14556=EDGE_CURVE('',#11746,#11744,#1210,.T.);
#14557=EDGE_CURVE('',#11745,#11747,#1211,.T.);
#14558=EDGE_CURVE('',#11748,#11749,#6070,.T.);
#14559=EDGE_CURVE('',#11748,#11746,#1212,.T.);
#14560=EDGE_CURVE('',#11747,#11749,#1213,.T.);
#14561=EDGE_CURVE('',#11750,#11751,#6071,.T.);
#14562=EDGE_CURVE('',#11750,#11748,#1214,.T.);
#14563=EDGE_CURVE('',#11749,#11751,#1215,.T.);
#14564=EDGE_CURVE('',#11752,#11753,#6072,.T.);
#14565=EDGE_CURVE('',#11752,#11750,#1216,.T.);
#14566=EDGE_CURVE('',#11751,#11753,#1217,.T.);
#14567=EDGE_CURVE('',#11754,#11755,#6073,.T.);
#14568=EDGE_CURVE('',#11754,#11752,#1218,.T.);
#14569=EDGE_CURVE('',#11753,#11755,#1219,.T.);
#14570=EDGE_CURVE('',#11756,#11757,#6074,.T.);
#14571=EDGE_CURVE('',#11756,#11754,#1220,.T.);
#14572=EDGE_CURVE('',#11755,#11757,#1221,.T.);
#14573=EDGE_CURVE('',#11758,#11759,#6075,.T.);
#14574=EDGE_CURVE('',#11758,#11756,#1222,.T.);
#14575=EDGE_CURVE('',#11757,#11759,#1223,.T.);
#14576=EDGE_CURVE('',#11760,#11761,#6076,.T.);
#14577=EDGE_CURVE('',#11760,#11758,#1224,.T.);
#14578=EDGE_CURVE('',#11759,#11761,#1225,.T.);
#14579=EDGE_CURVE('',#11762,#11763,#6077,.T.);
#14580=EDGE_CURVE('',#11762,#11760,#1226,.T.);
#14581=EDGE_CURVE('',#11761,#11763,#1227,.T.);
#14582=EDGE_CURVE('',#11764,#11765,#6078,.T.);
#14583=EDGE_CURVE('',#11764,#11766,#1228,.T.);
#14584=EDGE_CURVE('',#11765,#11766,#10811,.T.);
#14585=EDGE_CURVE('',#11767,#11768,#6079,.T.);
#14586=EDGE_CURVE('',#11767,#11764,#1229,.T.);
#14587=EDGE_CURVE('',#11769,#11765,#10812,.T.);
#14588=EDGE_CURVE('',#11768,#11769,#1230,.T.);
#14589=EDGE_CURVE('',#11770,#11771,#6080,.T.);
#14590=EDGE_CURVE('',#11770,#11767,#1231,.T.);
#14591=EDGE_CURVE('',#11771,#11768,#1232,.T.);
#14592=EDGE_CURVE('',#11772,#11773,#6081,.T.);
#14593=EDGE_CURVE('',#11772,#11770,#1233,.T.);
#14594=EDGE_CURVE('',#11773,#11771,#1234,.T.);
#14595=EDGE_CURVE('',#11774,#11775,#6082,.T.);
#14596=EDGE_CURVE('',#11774,#11772,#1235,.T.);
#14597=EDGE_CURVE('',#11775,#11773,#1236,.T.);
#14598=EDGE_CURVE('',#11776,#11777,#6083,.T.);
#14599=EDGE_CURVE('',#11776,#11774,#1237,.T.);
#14600=EDGE_CURVE('',#11777,#11775,#1238,.T.);
#14601=EDGE_CURVE('',#11778,#11779,#6084,.T.);
#14602=EDGE_CURVE('',#11778,#11776,#1239,.T.);
#14603=EDGE_CURVE('',#11779,#11777,#1240,.T.);
#14604=EDGE_CURVE('',#11780,#11781,#6085,.T.);
#14605=EDGE_CURVE('',#11780,#11778,#1241,.T.);
#14606=EDGE_CURVE('',#11781,#11779,#1242,.T.);
#14607=EDGE_CURVE('',#11782,#11783,#6086,.T.);
#14608=EDGE_CURVE('',#11782,#11780,#1243,.T.);
#14609=EDGE_CURVE('',#11783,#11781,#1244,.T.);
#14610=EDGE_CURVE('',#11784,#11785,#6087,.T.);
#14611=EDGE_CURVE('',#11784,#11782,#1245,.T.);
#14612=EDGE_CURVE('',#11785,#11783,#1246,.T.);
#14613=EDGE_CURVE('',#11786,#11787,#6088,.T.);
#14614=EDGE_CURVE('',#11786,#11784,#1247,.T.);
#14615=EDGE_CURVE('',#11787,#11785,#1248,.T.);
#14616=EDGE_CURVE('',#11788,#11789,#6089,.T.);
#14617=EDGE_CURVE('',#11788,#11786,#1249,.T.);
#14618=EDGE_CURVE('',#11789,#11787,#1250,.T.);
#14619=EDGE_CURVE('',#11790,#11791,#6090,.T.);
#14620=EDGE_CURVE('',#11790,#11788,#1251,.T.);
#14621=EDGE_CURVE('',#11791,#11789,#1252,.T.);
#14622=EDGE_CURVE('',#11792,#11793,#6091,.T.);
#14623=EDGE_CURVE('',#11792,#11790,#1253,.T.);
#14624=EDGE_CURVE('',#11793,#11791,#1254,.T.);
#14625=EDGE_CURVE('',#11794,#11795,#6092,.T.);
#14626=EDGE_CURVE('',#11794,#11792,#1255,.T.);
#14627=EDGE_CURVE('',#11795,#11793,#1256,.T.);
#14628=EDGE_CURVE('',#11796,#11797,#6093,.T.);
#14629=EDGE_CURVE('',#11796,#11794,#1257,.T.);
#14630=EDGE_CURVE('',#11797,#11795,#1258,.T.);
#14631=EDGE_CURVE('',#11798,#11799,#6094,.T.);
#14632=EDGE_CURVE('',#11798,#11796,#1259,.T.);
#14633=EDGE_CURVE('',#11799,#11797,#1260,.T.);
#14634=EDGE_CURVE('',#11800,#11801,#6095,.T.);
#14635=EDGE_CURVE('',#11800,#11798,#1261,.T.);
#14636=EDGE_CURVE('',#11801,#11799,#1262,.T.);
#14637=EDGE_CURVE('',#11802,#11803,#6096,.T.);
#14638=EDGE_CURVE('',#11802,#11800,#1263,.T.);
#14639=EDGE_CURVE('',#11803,#11801,#1264,.T.);
#14640=EDGE_CURVE('',#11804,#11805,#6097,.T.);
#14641=EDGE_CURVE('',#11804,#11802,#1265,.T.);
#14642=EDGE_CURVE('',#11805,#11803,#1266,.T.);
#14643=EDGE_CURVE('',#11806,#11807,#6098,.T.);
#14644=EDGE_CURVE('',#11806,#11804,#1267,.T.);
#14645=EDGE_CURVE('',#11807,#11805,#1268,.T.);
#14646=EDGE_CURVE('',#11808,#11809,#6099,.T.);
#14647=EDGE_CURVE('',#11808,#11806,#1269,.T.);
#14648=EDGE_CURVE('',#11809,#11807,#1270,.T.);
#14649=EDGE_CURVE('',#11810,#11811,#6100,.T.);
#14650=EDGE_CURVE('',#11810,#11808,#1271,.T.);
#14651=EDGE_CURVE('',#11811,#11809,#1272,.T.);
#14652=EDGE_CURVE('',#11812,#11813,#6101,.T.);
#14653=EDGE_CURVE('',#11812,#11810,#1273,.T.);
#14654=EDGE_CURVE('',#11813,#11811,#1274,.T.);
#14655=EDGE_CURVE('',#11814,#11815,#6102,.T.);
#14656=EDGE_CURVE('',#11814,#11812,#1275,.T.);
#14657=EDGE_CURVE('',#11815,#11813,#1276,.T.);
#14658=EDGE_CURVE('',#11816,#11817,#6103,.T.);
#14659=EDGE_CURVE('',#11816,#11814,#1277,.T.);
#14660=EDGE_CURVE('',#11817,#11815,#1278,.T.);
#14661=EDGE_CURVE('',#11818,#11819,#6104,.T.);
#14662=EDGE_CURVE('',#11818,#11816,#1279,.T.);
#14663=EDGE_CURVE('',#11819,#11817,#1280,.T.);
#14664=EDGE_CURVE('',#11820,#11821,#6105,.T.);
#14665=EDGE_CURVE('',#11820,#11818,#1281,.T.);
#14666=EDGE_CURVE('',#11821,#11819,#1282,.T.);
#14667=EDGE_CURVE('',#11822,#11823,#6106,.T.);
#14668=EDGE_CURVE('',#11822,#11820,#1283,.T.);
#14669=EDGE_CURVE('',#11823,#11821,#1284,.T.);
#14670=EDGE_CURVE('',#11766,#11824,#1285,.T.);
#14671=EDGE_CURVE('',#11825,#11824,#10813,.F.);
#14672=EDGE_CURVE('',#11826,#11825,#10814,.F.);
#14673=EDGE_CURVE('',#11826,#11769,#1286,.T.);
#14674=EDGE_CURVE('',#11763,#11826,#1287,.T.);
#14675=EDGE_CURVE('',#11827,#11707,#1288,.T.);
#14676=EDGE_CURVE('',#11827,#11823,#1289,.T.);
#14677=EDGE_CURVE('',#11707,#11828,#10815,.T.);
#14678=EDGE_CURVE('',#11828,#11706,#10816,.T.);
#14679=EDGE_CURVE('',#11706,#11829,#1290,.T.);
#14680=EDGE_CURVE('',#11829,#11827,#10817,.T.);
#14681=EDGE_CURVE('',#11829,#11822,#1291,.T.);
#14682=EDGE_CURVE('',#11824,#11762,#1292,.T.);
#14683=EDGE_CURVE('',#11830,#11831,#6107,.T.);
#14684=EDGE_CURVE('',#11831,#11830,#10818,.T.);
#14685=EDGE_CURVE('',#11831,#11832,#6108,.T.);
#14686=EDGE_CURVE('',#11832,#11831,#10819,.T.);
#14687=EDGE_CURVE('',#11832,#11833,#6109,.T.);
#14688=EDGE_CURVE('',#11833,#11832,#10820,.T.);
#14689=EDGE_CURVE('',#11833,#11834,#6110,.T.);
#14690=EDGE_CURVE('',#11834,#11833,#10821,.T.);
#14691=EDGE_CURVE('',#11834,#11835,#6111,.T.);
#14692=EDGE_CURVE('',#11835,#11834,#10822,.T.);
#14693=EDGE_CURVE('',#11835,#11830,#6112,.T.);
#14694=EDGE_CURVE('',#11830,#11835,#10823,.T.);
#14695=EDGE_CURVE('',#11836,#11837,#6113,.T.);
#14696=EDGE_CURVE('',#11838,#11837,#10824,.T.);
#14697=EDGE_CURVE('',#11832,#11838,#215,.T.);
#14698=EDGE_CURVE('',#11839,#11831,#216,.T.);
#14699=EDGE_CURVE('',#11840,#11839,#10825,.T.);
#14700=EDGE_CURVE('',#11831,#11840,#217,.T.);
#14701=EDGE_CURVE('',#11841,#11830,#218,.T.);
#14702=EDGE_CURVE('',#11842,#11841,#10826,.T.);
#14703=EDGE_CURVE('',#11830,#11842,#219,.T.);
#14704=EDGE_CURVE('',#11843,#11835,#220,.T.);
#14705=EDGE_CURVE('',#11844,#11843,#10827,.T.);
#14706=EDGE_CURVE('',#11835,#11844,#221,.T.);
#14707=EDGE_CURVE('',#11845,#11834,#222,.T.);
#14708=EDGE_CURVE('',#11846,#11845,#10828,.T.);
#14709=EDGE_CURVE('',#11834,#11846,#223,.T.);
#14710=EDGE_CURVE('',#11847,#11833,#224,.T.);
#14711=EDGE_CURVE('',#11848,#11847,#10829,.T.);
#14712=EDGE_CURVE('',#11833,#11848,#225,.T.);
#14713=EDGE_CURVE('',#11849,#11832,#226,.T.);
#14714=EDGE_CURVE('',#11837,#11849,#10830,.T.);
#14715=EDGE_CURVE('',#11850,#11833,#6114,.T.);
#14716=EDGE_CURVE('',#11851,#11850,#6115,.T.);
#14717=EDGE_CURVE('',#11851,#11832,#6116,.T.);
#14718=EDGE_CURVE('',#11832,#11852,#6117,.T.);
#14719=EDGE_CURVE('',#11852,#11849,#6118,.T.);
#14720=EDGE_CURVE('',#11853,#11834,#6119,.T.);
#14721=EDGE_CURVE('',#11850,#11853,#6120,.T.);
#14722=EDGE_CURVE('',#11846,#11854,#6121,.T.);
#14723=EDGE_CURVE('',#11834,#11854,#6122,.T.);
#14724=EDGE_CURVE('',#11833,#11855,#6123,.T.);
#14725=EDGE_CURVE('',#11855,#11847,#6124,.T.);
#14726=EDGE_CURVE('',#11856,#11851,#6125,.T.);
#14727=EDGE_CURVE('',#11856,#11831,#6126,.T.);
#14728=EDGE_CURVE('',#11831,#11857,#6127,.T.);
#14729=EDGE_CURVE('',#11857,#11839,#6128,.T.);
#14730=EDGE_CURVE('',#11858,#11835,#6129,.T.);
#14731=EDGE_CURVE('',#11853,#11858,#6130,.T.);
#14732=EDGE_CURVE('',#11844,#11859,#6131,.T.);
#14733=EDGE_CURVE('',#11835,#11859,#6132,.T.);
#14734=EDGE_CURVE('',#11854,#11845,#6133,.T.);
#14735=EDGE_CURVE('',#11848,#11855,#6134,.T.);
#14736=EDGE_CURVE('',#11859,#11843,#6135,.T.);
#14737=EDGE_CURVE('',#11860,#11841,#6136,.T.);
#14738=EDGE_CURVE('',#11842,#11860,#6137,.T.);
#14739=EDGE_CURVE('',#11840,#11857,#6138,.T.);
#14740=EDGE_CURVE('',#11838,#11852,#6139,.T.);
#14741=EDGE_CURVE('',#11861,#11830,#6140,.T.);
#14742=EDGE_CURVE('',#11858,#11861,#6141,.T.);
#14743=EDGE_CURVE('',#11830,#11860,#6142,.T.);
#14744=EDGE_CURVE('',#11861,#11856,#6143,.T.);
#14745=EDGE_CURVE('',#11862,#11862,#10831,.T.);
#14746=EDGE_CURVE('',#11828,#11862,#6144,.T.);
#14747=EDGE_CURVE('',#11824,#11826,#10832,.F.);
#14748=EDGE_CURVE('',#11863,#11863,#10833,.T.);
#14749=EDGE_CURVE('',#11863,#11825,#6145,.T.);
#19282=ORIENTED_EDGE('',*,*,#14494,.F.);
#19283=ORIENTED_EDGE('',*,*,#14495,.T.);
#19284=ORIENTED_EDGE('',*,*,#14496,.T.);
#19285=ORIENTED_EDGE('',*,*,#14497,.T.);
#19286=ORIENTED_EDGE('',*,*,#14498,.F.);
#19287=ORIENTED_EDGE('',*,*,#14499,.T.);
#19288=ORIENTED_EDGE('',*,*,#14494,.T.);
#19289=ORIENTED_EDGE('',*,*,#14500,.T.);
#19290=ORIENTED_EDGE('',*,*,#14501,.F.);
#19291=ORIENTED_EDGE('',*,*,#14502,.T.);
#19292=ORIENTED_EDGE('',*,*,#14498,.T.);
#19293=ORIENTED_EDGE('',*,*,#14503,.T.);
#19294=ORIENTED_EDGE('',*,*,#14504,.F.);
#19295=ORIENTED_EDGE('',*,*,#14505,.T.);
#19296=ORIENTED_EDGE('',*,*,#14501,.T.);
#19297=ORIENTED_EDGE('',*,*,#14506,.T.);
#19298=ORIENTED_EDGE('',*,*,#14507,.F.);
#19299=ORIENTED_EDGE('',*,*,#14508,.T.);
#19300=ORIENTED_EDGE('',*,*,#14504,.T.);
#19301=ORIENTED_EDGE('',*,*,#14509,.T.);
#19302=ORIENTED_EDGE('',*,*,#14510,.F.);
#19303=ORIENTED_EDGE('',*,*,#14511,.T.);
#19304=ORIENTED_EDGE('',*,*,#14507,.T.);
#19305=ORIENTED_EDGE('',*,*,#14512,.T.);
#19306=ORIENTED_EDGE('',*,*,#14513,.F.);
#19307=ORIENTED_EDGE('',*,*,#14514,.T.);
#19308=ORIENTED_EDGE('',*,*,#14510,.T.);
#19309=ORIENTED_EDGE('',*,*,#14515,.T.);
#19310=ORIENTED_EDGE('',*,*,#14516,.F.);
#19311=ORIENTED_EDGE('',*,*,#14517,.T.);
#19312=ORIENTED_EDGE('',*,*,#14513,.T.);
#19313=ORIENTED_EDGE('',*,*,#14518,.T.);
#19314=ORIENTED_EDGE('',*,*,#14519,.F.);
#19315=ORIENTED_EDGE('',*,*,#14520,.T.);
#19316=ORIENTED_EDGE('',*,*,#14516,.T.);
#19317=ORIENTED_EDGE('',*,*,#14521,.T.);
#19318=ORIENTED_EDGE('',*,*,#14522,.F.);
#19319=ORIENTED_EDGE('',*,*,#14523,.T.);
#19320=ORIENTED_EDGE('',*,*,#14519,.T.);
#19321=ORIENTED_EDGE('',*,*,#14524,.T.);
#19322=ORIENTED_EDGE('',*,*,#14525,.F.);
#19323=ORIENTED_EDGE('',*,*,#14526,.T.);
#19324=ORIENTED_EDGE('',*,*,#14522,.T.);
#19325=ORIENTED_EDGE('',*,*,#14527,.T.);
#19326=ORIENTED_EDGE('',*,*,#14528,.F.);
#19327=ORIENTED_EDGE('',*,*,#14529,.T.);
#19328=ORIENTED_EDGE('',*,*,#14525,.T.);
#19329=ORIENTED_EDGE('',*,*,#14530,.T.);
#19330=ORIENTED_EDGE('',*,*,#14531,.F.);
#19331=ORIENTED_EDGE('',*,*,#14532,.T.);
#19332=ORIENTED_EDGE('',*,*,#14528,.T.);
#19333=ORIENTED_EDGE('',*,*,#14533,.T.);
#19334=ORIENTED_EDGE('',*,*,#14534,.F.);
#19335=ORIENTED_EDGE('',*,*,#14535,.T.);
#19336=ORIENTED_EDGE('',*,*,#14531,.T.);
#19337=ORIENTED_EDGE('',*,*,#14536,.T.);
#19338=ORIENTED_EDGE('',*,*,#14537,.F.);
#19339=ORIENTED_EDGE('',*,*,#14538,.T.);
#19340=ORIENTED_EDGE('',*,*,#14534,.T.);
#19341=ORIENTED_EDGE('',*,*,#14539,.T.);
#19342=ORIENTED_EDGE('',*,*,#14540,.F.);
#19343=ORIENTED_EDGE('',*,*,#14541,.T.);
#19344=ORIENTED_EDGE('',*,*,#14537,.T.);
#19345=ORIENTED_EDGE('',*,*,#14542,.T.);
#19346=ORIENTED_EDGE('',*,*,#14543,.F.);
#19347=ORIENTED_EDGE('',*,*,#14544,.T.);
#19348=ORIENTED_EDGE('',*,*,#14540,.T.);
#19349=ORIENTED_EDGE('',*,*,#14545,.T.);
#19350=ORIENTED_EDGE('',*,*,#14546,.F.);
#19351=ORIENTED_EDGE('',*,*,#14547,.T.);
#19352=ORIENTED_EDGE('',*,*,#14543,.T.);
#19353=ORIENTED_EDGE('',*,*,#14548,.T.);
#19354=ORIENTED_EDGE('',*,*,#14549,.F.);
#19355=ORIENTED_EDGE('',*,*,#14550,.T.);
#19356=ORIENTED_EDGE('',*,*,#14546,.T.);
#19357=ORIENTED_EDGE('',*,*,#14551,.T.);
#19358=ORIENTED_EDGE('',*,*,#14552,.F.);
#19359=ORIENTED_EDGE('',*,*,#14553,.T.);
#19360=ORIENTED_EDGE('',*,*,#14549,.T.);
#19361=ORIENTED_EDGE('',*,*,#14554,.T.);
#19362=ORIENTED_EDGE('',*,*,#14555,.F.);
#19363=ORIENTED_EDGE('',*,*,#14556,.T.);
#19364=ORIENTED_EDGE('',*,*,#14552,.T.);
#19365=ORIENTED_EDGE('',*,*,#14557,.T.);
#19366=ORIENTED_EDGE('',*,*,#14558,.F.);
#19367=ORIENTED_EDGE('',*,*,#14559,.T.);
#19368=ORIENTED_EDGE('',*,*,#14555,.T.);
#19369=ORIENTED_EDGE('',*,*,#14560,.T.);
#19370=ORIENTED_EDGE('',*,*,#14561,.F.);
#19371=ORIENTED_EDGE('',*,*,#14562,.T.);
#19372=ORIENTED_EDGE('',*,*,#14558,.T.);
#19373=ORIENTED_EDGE('',*,*,#14563,.T.);
#19374=ORIENTED_EDGE('',*,*,#14564,.F.);
#19375=ORIENTED_EDGE('',*,*,#14565,.T.);
#19376=ORIENTED_EDGE('',*,*,#14561,.T.);
#19377=ORIENTED_EDGE('',*,*,#14566,.T.);
#19378=ORIENTED_EDGE('',*,*,#14567,.F.);
#19379=ORIENTED_EDGE('',*,*,#14568,.T.);
#19380=ORIENTED_EDGE('',*,*,#14564,.T.);
#19381=ORIENTED_EDGE('',*,*,#14569,.T.);
#19382=ORIENTED_EDGE('',*,*,#14570,.F.);
#19383=ORIENTED_EDGE('',*,*,#14571,.T.);
#19384=ORIENTED_EDGE('',*,*,#14567,.T.);
#19385=ORIENTED_EDGE('',*,*,#14572,.T.);
#19386=ORIENTED_EDGE('',*,*,#14573,.F.);
#19387=ORIENTED_EDGE('',*,*,#14574,.T.);
#19388=ORIENTED_EDGE('',*,*,#14570,.T.);
#19389=ORIENTED_EDGE('',*,*,#14575,.T.);
#19390=ORIENTED_EDGE('',*,*,#14576,.F.);
#19391=ORIENTED_EDGE('',*,*,#14577,.T.);
#19392=ORIENTED_EDGE('',*,*,#14573,.T.);
#19393=ORIENTED_EDGE('',*,*,#14578,.T.);
#19394=ORIENTED_EDGE('',*,*,#14579,.F.);
#19395=ORIENTED_EDGE('',*,*,#14580,.T.);
#19396=ORIENTED_EDGE('',*,*,#14576,.T.);
#19397=ORIENTED_EDGE('',*,*,#14581,.T.);
#19398=ORIENTED_EDGE('',*,*,#14582,.F.);
#19399=ORIENTED_EDGE('',*,*,#14583,.T.);
#19400=ORIENTED_EDGE('',*,*,#14584,.F.);
#19401=ORIENTED_EDGE('',*,*,#14585,.F.);
#19402=ORIENTED_EDGE('',*,*,#14586,.T.);
#19403=ORIENTED_EDGE('',*,*,#14582,.T.);
#19404=ORIENTED_EDGE('',*,*,#14587,.F.);
#19405=ORIENTED_EDGE('',*,*,#14588,.F.);
#19406=ORIENTED_EDGE('',*,*,#14589,.F.);
#19407=ORIENTED_EDGE('',*,*,#14590,.T.);
#19408=ORIENTED_EDGE('',*,*,#14585,.T.);
#19409=ORIENTED_EDGE('',*,*,#14591,.F.);
#19410=ORIENTED_EDGE('',*,*,#14592,.F.);
#19411=ORIENTED_EDGE('',*,*,#14593,.T.);
#19412=ORIENTED_EDGE('',*,*,#14589,.T.);
#19413=ORIENTED_EDGE('',*,*,#14594,.F.);
#19414=ORIENTED_EDGE('',*,*,#14595,.F.);
#19415=ORIENTED_EDGE('',*,*,#14596,.T.);
#19416=ORIENTED_EDGE('',*,*,#14592,.T.);
#19417=ORIENTED_EDGE('',*,*,#14597,.F.);
#19418=ORIENTED_EDGE('',*,*,#14598,.F.);
#19419=ORIENTED_EDGE('',*,*,#14599,.T.);
#19420=ORIENTED_EDGE('',*,*,#14595,.T.);
#19421=ORIENTED_EDGE('',*,*,#14600,.F.);
#19422=ORIENTED_EDGE('',*,*,#14601,.F.);
#19423=ORIENTED_EDGE('',*,*,#14602,.T.);
#19424=ORIENTED_EDGE('',*,*,#14598,.T.);
#19425=ORIENTED_EDGE('',*,*,#14603,.F.);
#19426=ORIENTED_EDGE('',*,*,#14604,.F.);
#19427=ORIENTED_EDGE('',*,*,#14605,.T.);
#19428=ORIENTED_EDGE('',*,*,#14601,.T.);
#19429=ORIENTED_EDGE('',*,*,#14606,.F.);
#19430=ORIENTED_EDGE('',*,*,#14607,.F.);
#19431=ORIENTED_EDGE('',*,*,#14608,.T.);
#19432=ORIENTED_EDGE('',*,*,#14604,.T.);
#19433=ORIENTED_EDGE('',*,*,#14609,.F.);
#19434=ORIENTED_EDGE('',*,*,#14610,.F.);
#19435=ORIENTED_EDGE('',*,*,#14611,.T.);
#19436=ORIENTED_EDGE('',*,*,#14607,.T.);
#19437=ORIENTED_EDGE('',*,*,#14612,.F.);
#19438=ORIENTED_EDGE('',*,*,#14613,.F.);
#19439=ORIENTED_EDGE('',*,*,#14614,.T.);
#19440=ORIENTED_EDGE('',*,*,#14610,.T.);
#19441=ORIENTED_EDGE('',*,*,#14615,.F.);
#19442=ORIENTED_EDGE('',*,*,#14616,.F.);
#19443=ORIENTED_EDGE('',*,*,#14617,.T.);
#19444=ORIENTED_EDGE('',*,*,#14613,.T.);
#19445=ORIENTED_EDGE('',*,*,#14618,.F.);
#19446=ORIENTED_EDGE('',*,*,#14619,.F.);
#19447=ORIENTED_EDGE('',*,*,#14620,.T.);
#19448=ORIENTED_EDGE('',*,*,#14616,.T.);
#19449=ORIENTED_EDGE('',*,*,#14621,.F.);
#19450=ORIENTED_EDGE('',*,*,#14622,.F.);
#19451=ORIENTED_EDGE('',*,*,#14623,.T.);
#19452=ORIENTED_EDGE('',*,*,#14619,.T.);
#19453=ORIENTED_EDGE('',*,*,#14624,.F.);
#19454=ORIENTED_EDGE('',*,*,#14625,.F.);
#19455=ORIENTED_EDGE('',*,*,#14626,.T.);
#19456=ORIENTED_EDGE('',*,*,#14622,.T.);
#19457=ORIENTED_EDGE('',*,*,#14627,.F.);
#19458=ORIENTED_EDGE('',*,*,#14628,.F.);
#19459=ORIENTED_EDGE('',*,*,#14629,.T.);
#19460=ORIENTED_EDGE('',*,*,#14625,.T.);
#19461=ORIENTED_EDGE('',*,*,#14630,.F.);
#19462=ORIENTED_EDGE('',*,*,#14631,.F.);
#19463=ORIENTED_EDGE('',*,*,#14632,.T.);
#19464=ORIENTED_EDGE('',*,*,#14628,.T.);
#19465=ORIENTED_EDGE('',*,*,#14633,.F.);
#19466=ORIENTED_EDGE('',*,*,#14634,.F.);
#19467=ORIENTED_EDGE('',*,*,#14635,.T.);
#19468=ORIENTED_EDGE('',*,*,#14631,.T.);
#19469=ORIENTED_EDGE('',*,*,#14636,.F.);
#19470=ORIENTED_EDGE('',*,*,#14637,.F.);
#19471=ORIENTED_EDGE('',*,*,#14638,.T.);
#19472=ORIENTED_EDGE('',*,*,#14634,.T.);
#19473=ORIENTED_EDGE('',*,*,#14639,.F.);
#19474=ORIENTED_EDGE('',*,*,#14640,.F.);
#19475=ORIENTED_EDGE('',*,*,#14641,.T.);
#19476=ORIENTED_EDGE('',*,*,#14637,.T.);
#19477=ORIENTED_EDGE('',*,*,#14642,.F.);
#19478=ORIENTED_EDGE('',*,*,#14643,.F.);
#19479=ORIENTED_EDGE('',*,*,#14644,.T.);
#19480=ORIENTED_EDGE('',*,*,#14640,.T.);
#19481=ORIENTED_EDGE('',*,*,#14645,.F.);
#19482=ORIENTED_EDGE('',*,*,#14646,.F.);
#19483=ORIENTED_EDGE('',*,*,#14647,.T.);
#19484=ORIENTED_EDGE('',*,*,#14643,.T.);
#19485=ORIENTED_EDGE('',*,*,#14648,.F.);
#19486=ORIENTED_EDGE('',*,*,#14649,.F.);
#19487=ORIENTED_EDGE('',*,*,#14650,.T.);
#19488=ORIENTED_EDGE('',*,*,#14646,.T.);
#19489=ORIENTED_EDGE('',*,*,#14651,.F.);
#19490=ORIENTED_EDGE('',*,*,#14652,.F.);
#19491=ORIENTED_EDGE('',*,*,#14653,.T.);
#19492=ORIENTED_EDGE('',*,*,#14649,.T.);
#19493=ORIENTED_EDGE('',*,*,#14654,.F.);
#19494=ORIENTED_EDGE('',*,*,#14655,.F.);
#19495=ORIENTED_EDGE('',*,*,#14656,.T.);
#19496=ORIENTED_EDGE('',*,*,#14652,.T.);
#19497=ORIENTED_EDGE('',*,*,#14657,.F.);
#19498=ORIENTED_EDGE('',*,*,#14658,.F.);
#19499=ORIENTED_EDGE('',*,*,#14659,.T.);
#19500=ORIENTED_EDGE('',*,*,#14655,.T.);
#19501=ORIENTED_EDGE('',*,*,#14660,.F.);
#19502=ORIENTED_EDGE('',*,*,#14661,.F.);
#19503=ORIENTED_EDGE('',*,*,#14662,.T.);
#19504=ORIENTED_EDGE('',*,*,#14658,.T.);
#19505=ORIENTED_EDGE('',*,*,#14663,.F.);
#19506=ORIENTED_EDGE('',*,*,#14664,.F.);
#19507=ORIENTED_EDGE('',*,*,#14665,.T.);
#19508=ORIENTED_EDGE('',*,*,#14661,.T.);
#19509=ORIENTED_EDGE('',*,*,#14666,.F.);
#19510=ORIENTED_EDGE('',*,*,#14667,.F.);
#19511=ORIENTED_EDGE('',*,*,#14668,.T.);
#19512=ORIENTED_EDGE('',*,*,#14664,.T.);
#19513=ORIENTED_EDGE('',*,*,#14669,.F.);
#19514=ORIENTED_EDGE('',*,*,#14587,.T.);
#19515=ORIENTED_EDGE('',*,*,#14584,.T.);
#19516=ORIENTED_EDGE('',*,*,#14670,.T.);
#19517=ORIENTED_EDGE('',*,*,#14671,.F.);
#19518=ORIENTED_EDGE('',*,*,#14672,.F.);
#19519=ORIENTED_EDGE('',*,*,#14673,.T.);
#19520=ORIENTED_EDGE('',*,*,#14673,.F.);
#19521=ORIENTED_EDGE('',*,*,#14674,.F.);
#19522=ORIENTED_EDGE('',*,*,#14581,.F.);
#19523=ORIENTED_EDGE('',*,*,#14578,.F.);
#19524=ORIENTED_EDGE('',*,*,#14575,.F.);
#19525=ORIENTED_EDGE('',*,*,#14572,.F.);
#19526=ORIENTED_EDGE('',*,*,#14569,.F.);
#19527=ORIENTED_EDGE('',*,*,#14566,.F.);
#19528=ORIENTED_EDGE('',*,*,#14563,.F.);
#19529=ORIENTED_EDGE('',*,*,#14560,.F.);
#19530=ORIENTED_EDGE('',*,*,#14557,.F.);
#19531=ORIENTED_EDGE('',*,*,#14554,.F.);
#19532=ORIENTED_EDGE('',*,*,#14551,.F.);
#19533=ORIENTED_EDGE('',*,*,#14548,.F.);
#19534=ORIENTED_EDGE('',*,*,#14545,.F.);
#19535=ORIENTED_EDGE('',*,*,#14542,.F.);
#19536=ORIENTED_EDGE('',*,*,#14539,.F.);
#19537=ORIENTED_EDGE('',*,*,#14536,.F.);
#19538=ORIENTED_EDGE('',*,*,#14533,.F.);
#19539=ORIENTED_EDGE('',*,*,#14530,.F.);
#19540=ORIENTED_EDGE('',*,*,#14527,.F.);
#19541=ORIENTED_EDGE('',*,*,#14524,.F.);
#19542=ORIENTED_EDGE('',*,*,#14521,.F.);
#19543=ORIENTED_EDGE('',*,*,#14518,.F.);
#19544=ORIENTED_EDGE('',*,*,#14515,.F.);
#19545=ORIENTED_EDGE('',*,*,#14512,.F.);
#19546=ORIENTED_EDGE('',*,*,#14509,.F.);
#19547=ORIENTED_EDGE('',*,*,#14506,.F.);
#19548=ORIENTED_EDGE('',*,*,#14503,.F.);
#19549=ORIENTED_EDGE('',*,*,#14500,.F.);
#19550=ORIENTED_EDGE('',*,*,#14497,.F.);
#19551=ORIENTED_EDGE('',*,*,#14675,.F.);
#19552=ORIENTED_EDGE('',*,*,#14676,.T.);
#19553=ORIENTED_EDGE('',*,*,#14669,.T.);
#19554=ORIENTED_EDGE('',*,*,#14666,.T.);
#19555=ORIENTED_EDGE('',*,*,#14663,.T.);
#19556=ORIENTED_EDGE('',*,*,#14660,.T.);
#19557=ORIENTED_EDGE('',*,*,#14657,.T.);
#19558=ORIENTED_EDGE('',*,*,#14654,.T.);
#19559=ORIENTED_EDGE('',*,*,#14651,.T.);
#19560=ORIENTED_EDGE('',*,*,#14648,.T.);
#19561=ORIENTED_EDGE('',*,*,#14645,.T.);
#19562=ORIENTED_EDGE('',*,*,#14642,.T.);
#19563=ORIENTED_EDGE('',*,*,#14639,.T.);
#19564=ORIENTED_EDGE('',*,*,#14636,.T.);
#19565=ORIENTED_EDGE('',*,*,#14633,.T.);
#19566=ORIENTED_EDGE('',*,*,#14630,.T.);
#19567=ORIENTED_EDGE('',*,*,#14627,.T.);
#19568=ORIENTED_EDGE('',*,*,#14624,.T.);
#19569=ORIENTED_EDGE('',*,*,#14621,.T.);
#19570=ORIENTED_EDGE('',*,*,#14618,.T.);
#19571=ORIENTED_EDGE('',*,*,#14615,.T.);
#19572=ORIENTED_EDGE('',*,*,#14612,.T.);
#19573=ORIENTED_EDGE('',*,*,#14609,.T.);
#19574=ORIENTED_EDGE('',*,*,#14606,.T.);
#19575=ORIENTED_EDGE('',*,*,#14603,.T.);
#19576=ORIENTED_EDGE('',*,*,#14600,.T.);
#19577=ORIENTED_EDGE('',*,*,#14597,.T.);
#19578=ORIENTED_EDGE('',*,*,#14594,.T.);
#19579=ORIENTED_EDGE('',*,*,#14591,.T.);
#19580=ORIENTED_EDGE('',*,*,#14588,.T.);
#19581=ORIENTED_EDGE('',*,*,#14677,.T.);
#19582=ORIENTED_EDGE('',*,*,#14678,.T.);
#19583=ORIENTED_EDGE('',*,*,#14679,.T.);
#19584=ORIENTED_EDGE('',*,*,#14680,.T.);
#19585=ORIENTED_EDGE('',*,*,#14675,.T.);
#19586=ORIENTED_EDGE('',*,*,#14667,.T.);
#19587=ORIENTED_EDGE('',*,*,#14676,.F.);
#19588=ORIENTED_EDGE('',*,*,#14680,.F.);
#19589=ORIENTED_EDGE('',*,*,#14681,.T.);
#19590=ORIENTED_EDGE('',*,*,#14670,.F.);
#19591=ORIENTED_EDGE('',*,*,#14583,.F.);
#19592=ORIENTED_EDGE('',*,*,#14586,.F.);
#19593=ORIENTED_EDGE('',*,*,#14590,.F.);
#19594=ORIENTED_EDGE('',*,*,#14593,.F.);
#19595=ORIENTED_EDGE('',*,*,#14596,.F.);
#19596=ORIENTED_EDGE('',*,*,#14599,.F.);
#19597=ORIENTED_EDGE('',*,*,#14602,.F.);
#19598=ORIENTED_EDGE('',*,*,#14605,.F.);
#19599=ORIENTED_EDGE('',*,*,#14608,.F.);
#19600=ORIENTED_EDGE('',*,*,#14611,.F.);
#19601=ORIENTED_EDGE('',*,*,#14614,.F.);
#19602=ORIENTED_EDGE('',*,*,#14617,.F.);
#19603=ORIENTED_EDGE('',*,*,#14620,.F.);
#19604=ORIENTED_EDGE('',*,*,#14623,.F.);
#19605=ORIENTED_EDGE('',*,*,#14626,.F.);
#19606=ORIENTED_EDGE('',*,*,#14629,.F.);
#19607=ORIENTED_EDGE('',*,*,#14632,.F.);
#19608=ORIENTED_EDGE('',*,*,#14635,.F.);
#19609=ORIENTED_EDGE('',*,*,#14638,.F.);
#19610=ORIENTED_EDGE('',*,*,#14641,.F.);
#19611=ORIENTED_EDGE('',*,*,#14644,.F.);
#19612=ORIENTED_EDGE('',*,*,#14647,.F.);
#19613=ORIENTED_EDGE('',*,*,#14650,.F.);
#19614=ORIENTED_EDGE('',*,*,#14653,.F.);
#19615=ORIENTED_EDGE('',*,*,#14656,.F.);
#19616=ORIENTED_EDGE('',*,*,#14659,.F.);
#19617=ORIENTED_EDGE('',*,*,#14662,.F.);
#19618=ORIENTED_EDGE('',*,*,#14665,.F.);
#19619=ORIENTED_EDGE('',*,*,#14668,.F.);
#19620=ORIENTED_EDGE('',*,*,#14681,.F.);
#19621=ORIENTED_EDGE('',*,*,#14679,.F.);
#19622=ORIENTED_EDGE('',*,*,#14495,.F.);
#19623=ORIENTED_EDGE('',*,*,#14499,.F.);
#19624=ORIENTED_EDGE('',*,*,#14502,.F.);
#19625=ORIENTED_EDGE('',*,*,#14505,.F.);
#19626=ORIENTED_EDGE('',*,*,#14508,.F.);
#19627=ORIENTED_EDGE('',*,*,#14511,.F.);
#19628=ORIENTED_EDGE('',*,*,#14514,.F.);
#19629=ORIENTED_EDGE('',*,*,#14517,.F.);
#19630=ORIENTED_EDGE('',*,*,#14520,.F.);
#19631=ORIENTED_EDGE('',*,*,#14523,.F.);
#19632=ORIENTED_EDGE('',*,*,#14526,.F.);
#19633=ORIENTED_EDGE('',*,*,#14529,.F.);
#19634=ORIENTED_EDGE('',*,*,#14532,.F.);
#19635=ORIENTED_EDGE('',*,*,#14535,.F.);
#19636=ORIENTED_EDGE('',*,*,#14538,.F.);
#19637=ORIENTED_EDGE('',*,*,#14541,.F.);
#19638=ORIENTED_EDGE('',*,*,#14544,.F.);
#19639=ORIENTED_EDGE('',*,*,#14547,.F.);
#19640=ORIENTED_EDGE('',*,*,#14550,.F.);
#19641=ORIENTED_EDGE('',*,*,#14553,.F.);
#19642=ORIENTED_EDGE('',*,*,#14556,.F.);
#19643=ORIENTED_EDGE('',*,*,#14559,.F.);
#19644=ORIENTED_EDGE('',*,*,#14562,.F.);
#19645=ORIENTED_EDGE('',*,*,#14565,.F.);
#19646=ORIENTED_EDGE('',*,*,#14568,.F.);
#19647=ORIENTED_EDGE('',*,*,#14571,.F.);
#19648=ORIENTED_EDGE('',*,*,#14574,.F.);
#19649=ORIENTED_EDGE('',*,*,#14577,.F.);
#19650=ORIENTED_EDGE('',*,*,#14580,.F.);
#19651=ORIENTED_EDGE('',*,*,#14682,.F.);
#19652=ORIENTED_EDGE('',*,*,#14683,.F.);
#19653=ORIENTED_EDGE('',*,*,#14684,.F.);
#19654=ORIENTED_EDGE('',*,*,#14685,.F.);
#19655=ORIENTED_EDGE('',*,*,#14686,.F.);
#19656=ORIENTED_EDGE('',*,*,#14687,.F.);
#19657=ORIENTED_EDGE('',*,*,#14688,.F.);
#19658=ORIENTED_EDGE('',*,*,#14689,.F.);
#19659=ORIENTED_EDGE('',*,*,#14690,.F.);
#19660=ORIENTED_EDGE('',*,*,#14691,.F.);
#19661=ORIENTED_EDGE('',*,*,#14692,.F.);
#19662=ORIENTED_EDGE('',*,*,#14693,.F.);
#19663=ORIENTED_EDGE('',*,*,#14694,.F.);
#19664=ORIENTED_EDGE('',*,*,#14695,.T.);
#19665=ORIENTED_EDGE('',*,*,#14696,.F.);
#19666=ORIENTED_EDGE('',*,*,#14697,.F.);
#19667=ORIENTED_EDGE('',*,*,#14686,.T.);
#19668=ORIENTED_EDGE('',*,*,#14698,.F.);
#19669=ORIENTED_EDGE('',*,*,#14699,.F.);
#19670=ORIENTED_EDGE('',*,*,#14700,.F.);
#19671=ORIENTED_EDGE('',*,*,#14684,.T.);
#19672=ORIENTED_EDGE('',*,*,#14701,.F.);
#19673=ORIENTED_EDGE('',*,*,#14702,.F.);
#19674=ORIENTED_EDGE('',*,*,#14703,.F.);
#19675=ORIENTED_EDGE('',*,*,#14694,.T.);
#19676=ORIENTED_EDGE('',*,*,#14704,.F.);
#19677=ORIENTED_EDGE('',*,*,#14705,.F.);
#19678=ORIENTED_EDGE('',*,*,#14706,.F.);
#19679=ORIENTED_EDGE('',*,*,#14692,.T.);
#19680=ORIENTED_EDGE('',*,*,#14707,.F.);
#19681=ORIENTED_EDGE('',*,*,#14708,.F.);
#19682=ORIENTED_EDGE('',*,*,#14709,.F.);
#19683=ORIENTED_EDGE('',*,*,#14690,.T.);
#19684=ORIENTED_EDGE('',*,*,#14710,.F.);
#19685=ORIENTED_EDGE('',*,*,#14711,.F.);
#19686=ORIENTED_EDGE('',*,*,#14712,.F.);
#19687=ORIENTED_EDGE('',*,*,#14688,.T.);
#19688=ORIENTED_EDGE('',*,*,#14713,.F.);
#19689=ORIENTED_EDGE('',*,*,#14714,.F.);
#19690=ORIENTED_EDGE('',*,*,#14695,.F.);
#19691=ORIENTED_EDGE('',*,*,#14687,.T.);
#19692=ORIENTED_EDGE('',*,*,#14715,.F.);
#19693=ORIENTED_EDGE('',*,*,#14716,.F.);
#19694=ORIENTED_EDGE('',*,*,#14717,.T.);
#19695=ORIENTED_EDGE('',*,*,#14713,.T.);
#19696=ORIENTED_EDGE('',*,*,#14718,.T.);
#19697=ORIENTED_EDGE('',*,*,#14719,.T.);
#19698=ORIENTED_EDGE('',*,*,#14689,.T.);
#19699=ORIENTED_EDGE('',*,*,#14720,.F.);
#19700=ORIENTED_EDGE('',*,*,#14721,.F.);
#19701=ORIENTED_EDGE('',*,*,#14715,.T.);
#19702=ORIENTED_EDGE('',*,*,#14709,.T.);
#19703=ORIENTED_EDGE('',*,*,#14722,.T.);
#19704=ORIENTED_EDGE('',*,*,#14723,.F.);
#19705=ORIENTED_EDGE('',*,*,#14710,.T.);
#19706=ORIENTED_EDGE('',*,*,#14724,.T.);
#19707=ORIENTED_EDGE('',*,*,#14725,.T.);
#19708=ORIENTED_EDGE('',*,*,#14685,.T.);
#19709=ORIENTED_EDGE('',*,*,#14717,.F.);
#19710=ORIENTED_EDGE('',*,*,#14726,.F.);
#19711=ORIENTED_EDGE('',*,*,#14727,.T.);
#19712=ORIENTED_EDGE('',*,*,#14698,.T.);
#19713=ORIENTED_EDGE('',*,*,#14728,.T.);
#19714=ORIENTED_EDGE('',*,*,#14729,.T.);
#19715=ORIENTED_EDGE('',*,*,#14691,.T.);
#19716=ORIENTED_EDGE('',*,*,#14730,.F.);
#19717=ORIENTED_EDGE('',*,*,#14731,.F.);
#19718=ORIENTED_EDGE('',*,*,#14720,.T.);
#19719=ORIENTED_EDGE('',*,*,#14706,.T.);
#19720=ORIENTED_EDGE('',*,*,#14732,.T.);
#19721=ORIENTED_EDGE('',*,*,#14733,.F.);
#19722=ORIENTED_EDGE('',*,*,#14707,.T.);
#19723=ORIENTED_EDGE('',*,*,#14723,.T.);
#19724=ORIENTED_EDGE('',*,*,#14734,.T.);
#19725=ORIENTED_EDGE('',*,*,#14711,.T.);
#19726=ORIENTED_EDGE('',*,*,#14725,.F.);
#19727=ORIENTED_EDGE('',*,*,#14735,.F.);
#19728=ORIENTED_EDGE('',*,*,#14708,.T.);
#19729=ORIENTED_EDGE('',*,*,#14734,.F.);
#19730=ORIENTED_EDGE('',*,*,#14722,.F.);
#19731=ORIENTED_EDGE('',*,*,#14705,.T.);
#19732=ORIENTED_EDGE('',*,*,#14736,.F.);
#19733=ORIENTED_EDGE('',*,*,#14732,.F.);
#19734=ORIENTED_EDGE('',*,*,#14702,.T.);
#19735=ORIENTED_EDGE('',*,*,#14737,.F.);
#19736=ORIENTED_EDGE('',*,*,#14738,.F.);
#19737=ORIENTED_EDGE('',*,*,#14699,.T.);
#19738=ORIENTED_EDGE('',*,*,#14729,.F.);
#19739=ORIENTED_EDGE('',*,*,#14739,.F.);
#19740=ORIENTED_EDGE('',*,*,#14696,.T.);
#19741=ORIENTED_EDGE('',*,*,#14714,.T.);
#19742=ORIENTED_EDGE('',*,*,#14719,.F.);
#19743=ORIENTED_EDGE('',*,*,#14740,.F.);
#19744=ORIENTED_EDGE('',*,*,#14693,.T.);
#19745=ORIENTED_EDGE('',*,*,#14741,.F.);
#19746=ORIENTED_EDGE('',*,*,#14742,.F.);
#19747=ORIENTED_EDGE('',*,*,#14730,.T.);
#19748=ORIENTED_EDGE('',*,*,#14703,.T.);
#19749=ORIENTED_EDGE('',*,*,#14738,.T.);
#19750=ORIENTED_EDGE('',*,*,#14743,.F.);
#19751=ORIENTED_EDGE('',*,*,#14704,.T.);
#19752=ORIENTED_EDGE('',*,*,#14733,.T.);
#19753=ORIENTED_EDGE('',*,*,#14736,.T.);
#19754=ORIENTED_EDGE('',*,*,#14701,.T.);
#19755=ORIENTED_EDGE('',*,*,#14743,.T.);
#19756=ORIENTED_EDGE('',*,*,#14737,.T.);
#19757=ORIENTED_EDGE('',*,*,#14683,.T.);
#19758=ORIENTED_EDGE('',*,*,#14727,.F.);
#19759=ORIENTED_EDGE('',*,*,#14744,.F.);
#19760=ORIENTED_EDGE('',*,*,#14741,.T.);
#19761=ORIENTED_EDGE('',*,*,#14712,.T.);
#19762=ORIENTED_EDGE('',*,*,#14735,.T.);
#19763=ORIENTED_EDGE('',*,*,#14724,.F.);
#19764=ORIENTED_EDGE('',*,*,#14697,.T.);
#19765=ORIENTED_EDGE('',*,*,#14740,.T.);
#19766=ORIENTED_EDGE('',*,*,#14718,.F.);
#19767=ORIENTED_EDGE('',*,*,#14700,.T.);
#19768=ORIENTED_EDGE('',*,*,#14739,.T.);
#19769=ORIENTED_EDGE('',*,*,#14728,.F.);
#19770=ORIENTED_EDGE('',*,*,#14745,.F.);
#19771=ORIENTED_EDGE('',*,*,#14677,.F.);
#19772=ORIENTED_EDGE('',*,*,#14496,.F.);
#19773=ORIENTED_EDGE('',*,*,#14678,.F.);
#19774=ORIENTED_EDGE('',*,*,#14746,.T.);
#19775=ORIENTED_EDGE('',*,*,#14745,.T.);
#19776=ORIENTED_EDGE('',*,*,#14746,.F.);
#19777=ORIENTED_EDGE('',*,*,#14579,.T.);
#19778=ORIENTED_EDGE('',*,*,#14674,.T.);
#19779=ORIENTED_EDGE('',*,*,#14747,.F.);
#19780=ORIENTED_EDGE('',*,*,#14682,.T.);
#19781=ORIENTED_EDGE('',*,*,#14748,.F.);
#19782=ORIENTED_EDGE('',*,*,#14749,.T.);
#19783=ORIENTED_EDGE('',*,*,#14671,.T.);
#19784=ORIENTED_EDGE('',*,*,#14747,.T.);
#19785=ORIENTED_EDGE('',*,*,#14672,.T.);
#19786=ORIENTED_EDGE('',*,*,#14749,.F.);
#19787=ORIENTED_EDGE('',*,*,#14748,.T.);
#19788=ORIENTED_EDGE('',*,*,#14731,.T.);
#19789=ORIENTED_EDGE('',*,*,#14742,.T.);
#19790=ORIENTED_EDGE('',*,*,#14744,.T.);
#19791=ORIENTED_EDGE('',*,*,#14726,.T.);
#19792=ORIENTED_EDGE('',*,*,#14716,.T.);
#19793=ORIENTED_EDGE('',*,*,#14721,.T.);
#25330=CONICAL_SURFACE('',#27629,0.23094010767585,1.02878638855047);
#25331=CONICAL_SURFACE('',#27663,0.7,0.785398163397448);
#25332=CONICAL_SURFACE('',#27666,0.76,0.785398163397449);
#25725=ADVANCED_FACE('',(#2912),#622,.T.);
#25726=ADVANCED_FACE('',(#2913),#623,.T.);
#25727=ADVANCED_FACE('',(#2914),#624,.T.);
#25728=ADVANCED_FACE('',(#2915),#625,.T.);
#25729=ADVANCED_FACE('',(#2916),#626,.T.);
#25730=ADVANCED_FACE('',(#2917),#627,.T.);
#25731=ADVANCED_FACE('',(#2918),#628,.T.);
#25732=ADVANCED_FACE('',(#2919),#629,.T.);
#25733=ADVANCED_FACE('',(#2920),#630,.T.);
#25734=ADVANCED_FACE('',(#2921),#631,.T.);
#25735=ADVANCED_FACE('',(#2922),#632,.T.);
#25736=ADVANCED_FACE('',(#2923),#633,.T.);
#25737=ADVANCED_FACE('',(#2924),#634,.T.);
#25738=ADVANCED_FACE('',(#2925),#635,.T.);
#25739=ADVANCED_FACE('',(#2926),#636,.T.);
#25740=ADVANCED_FACE('',(#2927),#637,.T.);
#25741=ADVANCED_FACE('',(#2928),#638,.T.);
#25742=ADVANCED_FACE('',(#2929),#639,.T.);
#25743=ADVANCED_FACE('',(#2930),#640,.T.);
#25744=ADVANCED_FACE('',(#2931),#641,.T.);
#25745=ADVANCED_FACE('',(#2932),#642,.T.);
#25746=ADVANCED_FACE('',(#2933),#643,.T.);
#25747=ADVANCED_FACE('',(#2934),#644,.T.);
#25748=ADVANCED_FACE('',(#2935),#645,.T.);
#25749=ADVANCED_FACE('',(#2936),#646,.T.);
#25750=ADVANCED_FACE('',(#2937),#647,.T.);
#25751=ADVANCED_FACE('',(#2938),#648,.T.);
#25752=ADVANCED_FACE('',(#2939),#649,.T.);
#25753=ADVANCED_FACE('',(#2940),#650,.T.);
#25754=ADVANCED_FACE('',(#2941),#651,.T.);
#25755=ADVANCED_FACE('',(#2942),#652,.T.);
#25756=ADVANCED_FACE('',(#2943),#653,.T.);
#25757=ADVANCED_FACE('',(#2944),#654,.T.);
#25758=ADVANCED_FACE('',(#2945),#655,.T.);
#25759=ADVANCED_FACE('',(#2946),#656,.T.);
#25760=ADVANCED_FACE('',(#2947),#657,.T.);
#25761=ADVANCED_FACE('',(#2948),#658,.T.);
#25762=ADVANCED_FACE('',(#2949),#659,.T.);
#25763=ADVANCED_FACE('',(#2950),#660,.T.);
#25764=ADVANCED_FACE('',(#2951),#661,.T.);
#25765=ADVANCED_FACE('',(#2952),#662,.T.);
#25766=ADVANCED_FACE('',(#2953),#663,.T.);
#25767=ADVANCED_FACE('',(#2954),#664,.T.);
#25768=ADVANCED_FACE('',(#2955),#665,.T.);
#25769=ADVANCED_FACE('',(#2956),#666,.T.);
#25770=ADVANCED_FACE('',(#2957),#667,.T.);
#25771=ADVANCED_FACE('',(#2958),#668,.T.);
#25772=ADVANCED_FACE('',(#2959),#669,.T.);
#25773=ADVANCED_FACE('',(#2960),#670,.T.);
#25774=ADVANCED_FACE('',(#2961),#671,.T.);
#25775=ADVANCED_FACE('',(#2962),#672,.T.);
#25776=ADVANCED_FACE('',(#2963),#673,.T.);
#25777=ADVANCED_FACE('',(#2964),#674,.T.);
#25778=ADVANCED_FACE('',(#2965),#675,.T.);
#25779=ADVANCED_FACE('',(#2966),#676,.T.);
#25780=ADVANCED_FACE('',(#2967),#677,.T.);
#25781=ADVANCED_FACE('',(#2968),#678,.T.);
#25782=ADVANCED_FACE('',(#2969),#679,.T.);
#25783=ADVANCED_FACE('',(#2970),#1835,.F.);
#25784=ADVANCED_FACE('',(#2971),#276,.F.);
#25785=ADVANCED_FACE('',(#2972),#1836,.T.);
#25786=ADVANCED_FACE('',(#2973),#680,.T.);
#25787=ADVANCED_FACE('',(#2974),#277,.F.);
#25788=ADVANCED_FACE('',(#2975),#1837,.F.);
#25789=ADVANCED_FACE('',(#2976),#1838,.F.);
#25790=ADVANCED_FACE('',(#2977),#1839,.F.);
#25791=ADVANCED_FACE('',(#2978),#1840,.F.);
#25792=ADVANCED_FACE('',(#2979),#1841,.F.);
#25793=ADVANCED_FACE('',(#2980),#1842,.F.);
#25794=ADVANCED_FACE('',(#2981),#25330,.F.);
#25795=ADVANCED_FACE('',(#2982),#1843,.F.);
#25796=ADVANCED_FACE('',(#2983),#1844,.F.);
#25797=ADVANCED_FACE('',(#2984),#1845,.F.);
#25798=ADVANCED_FACE('',(#2985),#1846,.F.);
#25799=ADVANCED_FACE('',(#2986),#1847,.F.);
#25800=ADVANCED_FACE('',(#2987),#1848,.F.);
#25801=ADVANCED_FACE('',(#2988),#1849,.F.);
#25802=ADVANCED_FACE('',(#2989),#1850,.F.);
#25803=ADVANCED_FACE('',(#2990),#1851,.F.);
#25804=ADVANCED_FACE('',(#2991),#1852,.F.);
#25805=ADVANCED_FACE('',(#2992),#1853,.F.);
#25806=ADVANCED_FACE('',(#2993),#1854,.F.);
#25807=ADVANCED_FACE('',(#2994),#1855,.F.);
#25808=ADVANCED_FACE('',(#2995),#1856,.F.);
#25809=ADVANCED_FACE('',(#2996),#1857,.F.);
#25810=ADVANCED_FACE('',(#2997),#1858,.F.);
#25811=ADVANCED_FACE('',(#2998),#1859,.F.);
#25812=ADVANCED_FACE('',(#2999),#1860,.F.);
#25813=ADVANCED_FACE('',(#3000),#1861,.F.);
#25814=ADVANCED_FACE('',(#3001),#1862,.F.);
#25815=ADVANCED_FACE('',(#3002),#1863,.F.);
#25816=ADVANCED_FACE('',(#3003),#1864,.F.);
#25817=ADVANCED_FACE('',(#3004),#1865,.F.);
#25818=ADVANCED_FACE('',(#3005),#1866,.F.);
#25819=ADVANCED_FACE('',(#3006),#1867,.T.);
#25820=ADVANCED_FACE('',(#3007),#25331,.T.);
#25821=ADVANCED_FACE('',(#3008),#681,.T.);
#25822=ADVANCED_FACE('',(#3009),#25332,.T.);
#25823=ADVANCED_FACE('',(#3010,#864),#1868,.T.);
#26879=CLOSED_SHELL('',(#25725,#25726,#25727,#25728,#25729,#25730,#25731,
#25732,#25733,#25734,#25735,#25736,#25737,#25738,#25739,#25740,#25741,#25742,
#25743,#25744,#25745,#25746,#25747,#25748,#25749,#25750,#25751,#25752,#25753,
#25754,#25755,#25756,#25757,#25758,#25759,#25760,#25761,#25762,#25763,#25764,
#25765,#25766,#25767,#25768,#25769,#25770,#25771,#25772,#25773,#25774,#25775,
#25776,#25777,#25778,#25779,#25780,#25781,#25782,#25783,#25784,#25785,#25786,
#25787,#25788,#25789,#25790,#25791,#25792,#25793,#25794,#25795,#25796,#25797,
#25798,#25799,#25800,#25801,#25802,#25803,#25804,#25805,#25806,#25807,#25808,
#25809,#25810,#25811,#25812,#25813,#25814,#25815,#25816,#25817,#25818,#25819,
#25820,#25821,#25822,#25823));
#27547=AXIS2_PLACEMENT_3D('',#47588,#30392,#30393);
#27548=AXIS2_PLACEMENT_3D('',#47589,#30394,#30395);
#27549=AXIS2_PLACEMENT_3D('',#47611,#30397,#30398);
#27550=AXIS2_PLACEMENT_3D('',#47622,#30399,#30400);
#27551=AXIS2_PLACEMENT_3D('',#47706,#30402,#30403);
#27552=AXIS2_PLACEMENT_3D('',#47796,#30405,#30406);
#27553=AXIS2_PLACEMENT_3D('',#47886,#30408,#30409);
#27554=AXIS2_PLACEMENT_3D('',#47970,#30411,#30412);
#27555=AXIS2_PLACEMENT_3D('',#48060,#30414,#30415);
#27556=AXIS2_PLACEMENT_3D('',#48144,#30417,#30418);
#27557=AXIS2_PLACEMENT_3D('',#48234,#30420,#30421);
#27558=AXIS2_PLACEMENT_3D('',#48324,#30423,#30424);
#27559=AXIS2_PLACEMENT_3D('',#48408,#30426,#30427);
#27560=AXIS2_PLACEMENT_3D('',#48498,#30429,#30430);
#27561=AXIS2_PLACEMENT_3D('',#48582,#30432,#30433);
#27562=AXIS2_PLACEMENT_3D('',#48672,#30435,#30436);
#27563=AXIS2_PLACEMENT_3D('',#48762,#30438,#30439);
#27564=AXIS2_PLACEMENT_3D('',#48846,#30441,#30442);
#27565=AXIS2_PLACEMENT_3D('',#48936,#30444,#30445);
#27566=AXIS2_PLACEMENT_3D('',#49026,#30447,#30448);
#27567=AXIS2_PLACEMENT_3D('',#49110,#30450,#30451);
#27568=AXIS2_PLACEMENT_3D('',#49200,#30453,#30454);
#27569=AXIS2_PLACEMENT_3D('',#49284,#30456,#30457);
#27570=AXIS2_PLACEMENT_3D('',#49374,#30459,#30460);
#27571=AXIS2_PLACEMENT_3D('',#49464,#30462,#30463);
#27572=AXIS2_PLACEMENT_3D('',#49548,#30465,#30466);
#27573=AXIS2_PLACEMENT_3D('',#49638,#30468,#30469);
#27574=AXIS2_PLACEMENT_3D('',#49722,#30471,#30472);
#27575=AXIS2_PLACEMENT_3D('',#49812,#30474,#30475);
#27576=AXIS2_PLACEMENT_3D('',#49902,#30477,#30478);
#27577=AXIS2_PLACEMENT_3D('',#49986,#30480,#30481);
#27578=AXIS2_PLACEMENT_3D('',#50076,#30483,#30484);
#27579=AXIS2_PLACEMENT_3D('',#50085,#30486,#30487);
#27580=AXIS2_PLACEMENT_3D('',#50086,#30488,#30489);
#27581=AXIS2_PLACEMENT_3D('',#50108,#30491,#30492);
#27582=AXIS2_PLACEMENT_3D('',#50123,#30493,#30494);
#27583=AXIS2_PLACEMENT_3D('',#50160,#30496,#30497);
#27584=AXIS2_PLACEMENT_3D('',#50197,#30499,#30500);
#27585=AXIS2_PLACEMENT_3D('',#50235,#30502,#30503);
#27586=AXIS2_PLACEMENT_3D('',#50272,#30505,#30506);
#27587=AXIS2_PLACEMENT_3D('',#50309,#30508,#30509);
#27588=AXIS2_PLACEMENT_3D('',#50346,#30511,#30512);
#27589=AXIS2_PLACEMENT_3D('',#50383,#30514,#30515);
#27590=AXIS2_PLACEMENT_3D('',#50421,#30517,#30518);
#27591=AXIS2_PLACEMENT_3D('',#50458,#30520,#30521);
#27592=AXIS2_PLACEMENT_3D('',#50495,#30523,#30524);
#27593=AXIS2_PLACEMENT_3D('',#50532,#30526,#30527);
#27594=AXIS2_PLACEMENT_3D('',#50569,#30529,#30530);
#27595=AXIS2_PLACEMENT_3D('',#50607,#30532,#30533);
#27596=AXIS2_PLACEMENT_3D('',#50644,#30535,#30536);
#27597=AXIS2_PLACEMENT_3D('',#50681,#30538,#30539);
#27598=AXIS2_PLACEMENT_3D('',#50719,#30541,#30542);
#27599=AXIS2_PLACEMENT_3D('',#50756,#30544,#30545);
#27600=AXIS2_PLACEMENT_3D('',#50793,#30547,#30548);
#27601=AXIS2_PLACEMENT_3D('',#50830,#30550,#30551);
#27602=AXIS2_PLACEMENT_3D('',#50867,#30553,#30554);
#27603=AXIS2_PLACEMENT_3D('',#50905,#30556,#30557);
#27604=AXIS2_PLACEMENT_3D('',#50942,#30559,#30560);
#27605=AXIS2_PLACEMENT_3D('',#50979,#30562,#30563);
#27606=AXIS2_PLACEMENT_3D('',#51016,#30565,#30566);
#27607=AXIS2_PLACEMENT_3D('',#51053,#30568,#30569);
#27608=AXIS2_PLACEMENT_3D('',#51091,#30571,#30572);
#27609=AXIS2_PLACEMENT_3D('',#51128,#30574,#30575);
#27610=AXIS2_PLACEMENT_3D('',#51204,#30576,#30577);
#27611=AXIS2_PLACEMENT_3D('',#51206,#30578,#30579);
#27612=AXIS2_PLACEMENT_3D('',#52869,#30580,#30581);
#27613=AXIS2_PLACEMENT_3D('',#52871,#30582,#30583);
#27614=AXIS2_PLACEMENT_3D('',#52872,#30584,#30585);
#27615=AXIS2_PLACEMENT_3D('',#52950,#30586,#30587);
#27616=AXIS2_PLACEMENT_3D('',#52951,#30588,#30589);
#27617=AXIS2_PLACEMENT_3D('',#54456,#30590,#30591);
#27618=AXIS2_PLACEMENT_3D('',#54460,#30593,#30594);
#27619=AXIS2_PLACEMENT_3D('',#54461,#30595,#30596);
#27620=AXIS2_PLACEMENT_3D('',#54464,#30598,#30599);
#27621=AXIS2_PLACEMENT_3D('',#54465,#30600,#30601);
#27622=AXIS2_PLACEMENT_3D('',#54468,#30603,#30604);
#27623=AXIS2_PLACEMENT_3D('',#54469,#30605,#30606);
#27624=AXIS2_PLACEMENT_3D('',#54472,#30608,#30609);
#27625=AXIS2_PLACEMENT_3D('',#54473,#30610,#30611);
#27626=AXIS2_PLACEMENT_3D('',#54476,#30613,#30614);
#27627=AXIS2_PLACEMENT_3D('',#54477,#30615,#30616);
#27628=AXIS2_PLACEMENT_3D('',#54479,#30618,#30619);
#27629=AXIS2_PLACEMENT_3D('',#54480,#30620,#30621);
#27630=AXIS2_PLACEMENT_3D('',#54485,#30623,#30624);
#27631=AXIS2_PLACEMENT_3D('',#54494,#30625,#30626);
#27632=AXIS2_PLACEMENT_3D('',#54503,#30627,#30628);
#27633=AXIS2_PLACEMENT_3D('',#54512,#30629,#30630);
#27634=AXIS2_PLACEMENT_3D('',#54521,#30631,#30632);
#27635=AXIS2_PLACEMENT_3D('',#54530,#30633,#30634);
#27636=AXIS2_PLACEMENT_3D('',#54538,#30635,#30636);
#27637=AXIS2_PLACEMENT_3D('',#54539,#30637,#30638);
#27638=AXIS2_PLACEMENT_3D('',#54545,#30642,#30643);
#27639=AXIS2_PLACEMENT_3D('',#54549,#30646,#30647);
#27640=AXIS2_PLACEMENT_3D('',#54553,#30650,#30651);
#27641=AXIS2_PLACEMENT_3D('',#54557,#30654,#30655);
#27642=AXIS2_PLACEMENT_3D('',#54561,#30658,#30659);
#27643=AXIS2_PLACEMENT_3D('',#54565,#30662,#30663);
#27644=AXIS2_PLACEMENT_3D('',#54569,#30666,#30667);
#27645=AXIS2_PLACEMENT_3D('',#54573,#30670,#30671);
#27646=AXIS2_PLACEMENT_3D('',#54577,#30674,#30675);
#27647=AXIS2_PLACEMENT_3D('',#54579,#30677,#30678);
#27648=AXIS2_PLACEMENT_3D('',#54581,#30680,#30681);
#27649=AXIS2_PLACEMENT_3D('',#54582,#30682,#30683);
#27650=AXIS2_PLACEMENT_3D('',#54584,#30685,#30686);
#27651=AXIS2_PLACEMENT_3D('',#54588,#30689,#30690);
#27652=AXIS2_PLACEMENT_3D('',#54590,#30692,#30693);
#27653=AXIS2_PLACEMENT_3D('',#54592,#30695,#30696);
#27654=AXIS2_PLACEMENT_3D('',#54596,#30699,#30700);
#27655=AXIS2_PLACEMENT_3D('',#54598,#30702,#30703);
#27656=AXIS2_PLACEMENT_3D('',#54599,#30704,#30705);
#27657=AXIS2_PLACEMENT_3D('',#54600,#30706,#30707);
#27658=AXIS2_PLACEMENT_3D('',#54602,#30709,#30710);
#27659=AXIS2_PLACEMENT_3D('',#54603,#30711,#30712);
#27660=AXIS2_PLACEMENT_3D('',#54604,#30713,#30714);
#27661=AXIS2_PLACEMENT_3D('',#54605,#30715,#30716);
#27662=AXIS2_PLACEMENT_3D('',#54607,#30717,#30718);
#27663=AXIS2_PLACEMENT_3D('',#54608,#30719,#30720);
#27664=AXIS2_PLACEMENT_3D('',#54610,#30722,#30723);
#27665=AXIS2_PLACEMENT_3D('',#54611,#30724,#30725);
#27666=AXIS2_PLACEMENT_3D('',#54612,#30726,#30727);
#27667=AXIS2_PLACEMENT_3D('',#54614,#30728,#30729);
#27668=AXIS2_PLACEMENT_3D('',#54616,#30731,#30732);
#30392=DIRECTION('axis',(0.,0.,1.));
#30393=DIRECTION('refdir',(1.,0.,0.));
#30394=DIRECTION('center_axis',(0.,0.,1.));
#30395=DIRECTION('ref_axis',(1.,0.,0.));
#30396=DIRECTION('',(0.,0.,-1.));
#30397=DIRECTION('center_axis',(0.,0.,1.));
#30398=DIRECTION('ref_axis',(1.,0.,0.));
#30399=DIRECTION('center_axis',(0.,0.,1.));
#30400=DIRECTION('ref_axis',(1.,0.,0.));
#30401=DIRECTION('',(0.,0.,-1.));
#30402=DIRECTION('center_axis',(0.,0.,1.));
#30403=DIRECTION('ref_axis',(1.,0.,0.));
#30404=DIRECTION('',(0.,0.,-1.));
#30405=DIRECTION('center_axis',(0.,0.,1.));
#30406=DIRECTION('ref_axis',(1.,0.,0.));
#30407=DIRECTION('',(0.,0.,-1.));
#30408=DIRECTION('center_axis',(0.,0.,1.));
#30409=DIRECTION('ref_axis',(1.,0.,0.));
#30410=DIRECTION('',(0.,0.,-1.));
#30411=DIRECTION('center_axis',(0.,0.,1.));
#30412=DIRECTION('ref_axis',(1.,0.,0.));
#30413=DIRECTION('',(0.,0.,-1.));
#30414=DIRECTION('center_axis',(0.,0.,1.));
#30415=DIRECTION('ref_axis',(1.,0.,0.));
#30416=DIRECTION('',(0.,0.,-1.));
#30417=DIRECTION('center_axis',(0.,0.,1.));
#30418=DIRECTION('ref_axis',(1.,0.,0.));
#30419=DIRECTION('',(0.,0.,-1.));
#30420=DIRECTION('center_axis',(0.,0.,1.));
#30421=DIRECTION('ref_axis',(1.,0.,0.));
#30422=DIRECTION('',(0.,0.,-1.));
#30423=DIRECTION('center_axis',(0.,0.,1.));
#30424=DIRECTION('ref_axis',(1.,0.,0.));
#30425=DIRECTION('',(0.,0.,-1.));
#30426=DIRECTION('center_axis',(0.,0.,1.));
#30427=DIRECTION('ref_axis',(1.,0.,0.));
#30428=DIRECTION('',(0.,0.,-1.));
#30429=DIRECTION('center_axis',(0.,0.,1.));
#30430=DIRECTION('ref_axis',(1.,0.,0.));
#30431=DIRECTION('',(0.,0.,-1.));
#30432=DIRECTION('center_axis',(0.,0.,1.));
#30433=DIRECTION('ref_axis',(1.,0.,0.));
#30434=DIRECTION('',(0.,0.,-1.));
#30435=DIRECTION('center_axis',(0.,0.,1.));
#30436=DIRECTION('ref_axis',(1.,0.,0.));
#30437=DIRECTION('',(0.,0.,-1.));
#30438=DIRECTION('center_axis',(0.,0.,1.));
#30439=DIRECTION('ref_axis',(1.,0.,0.));
#30440=DIRECTION('',(0.,0.,-1.));
#30441=DIRECTION('center_axis',(0.,0.,1.));
#30442=DIRECTION('ref_axis',(1.,0.,0.));
#30443=DIRECTION('',(0.,0.,-1.));
#30444=DIRECTION('center_axis',(0.,0.,1.));
#30445=DIRECTION('ref_axis',(1.,0.,0.));
#30446=DIRECTION('',(0.,0.,-1.));
#30447=DIRECTION('center_axis',(0.,0.,1.));
#30448=DIRECTION('ref_axis',(1.,0.,0.));
#30449=DIRECTION('',(0.,0.,-1.));
#30450=DIRECTION('center_axis',(0.,0.,1.));
#30451=DIRECTION('ref_axis',(1.,0.,0.));
#30452=DIRECTION('',(0.,0.,-1.));
#30453=DIRECTION('center_axis',(0.,0.,1.));
#30454=DIRECTION('ref_axis',(1.,0.,0.));
#30455=DIRECTION('',(0.,0.,-1.));
#30456=DIRECTION('center_axis',(0.,0.,1.));
#30457=DIRECTION('ref_axis',(1.,0.,0.));
#30458=DIRECTION('',(0.,0.,-1.));
#30459=DIRECTION('center_axis',(0.,0.,1.));
#30460=DIRECTION('ref_axis',(1.,0.,0.));
#30461=DIRECTION('',(0.,0.,-1.));
#30462=DIRECTION('center_axis',(0.,0.,1.));
#30463=DIRECTION('ref_axis',(1.,0.,0.));
#30464=DIRECTION('',(0.,0.,-1.));
#30465=DIRECTION('center_axis',(0.,0.,1.));
#30466=DIRECTION('ref_axis',(1.,0.,0.));
#30467=DIRECTION('',(0.,0.,-1.));
#30468=DIRECTION('center_axis',(0.,0.,1.));
#30469=DIRECTION('ref_axis',(1.,0.,0.));
#30470=DIRECTION('',(0.,0.,-1.));
#30471=DIRECTION('center_axis',(0.,0.,1.));
#30472=DIRECTION('ref_axis',(1.,0.,0.));
#30473=DIRECTION('',(0.,0.,-1.));
#30474=DIRECTION('center_axis',(0.,0.,1.));
#30475=DIRECTION('ref_axis',(1.,0.,0.));
#30476=DIRECTION('',(0.,0.,-1.));
#30477=DIRECTION('center_axis',(0.,0.,1.));
#30478=DIRECTION('ref_axis',(1.,0.,0.));
#30479=DIRECTION('',(0.,0.,-1.));
#30480=DIRECTION('center_axis',(0.,0.,1.));
#30481=DIRECTION('ref_axis',(1.,0.,0.));
#30482=DIRECTION('',(0.,0.,-1.));
#30483=DIRECTION('center_axis',(0.,0.,1.));
#30484=DIRECTION('ref_axis',(-0.993035081806481,-0.11781904048835,0.));
#30485=DIRECTION('',(0.,0.,1.));
#30486=DIRECTION('center_axis',(0.,0.,1.));
#30487=DIRECTION('ref_axis',(1.,-1.07699989592456E-13,0.));
#30488=DIRECTION('center_axis',(0.,0.,1.));
#30489=DIRECTION('ref_axis',(1.,-1.07699989592456E-13,0.));
#30490=DIRECTION('',(0.,0.,1.));
#30491=DIRECTION('center_axis',(0.,0.,1.));
#30492=DIRECTION('ref_axis',(1.,-1.07699989592456E-13,0.));
#30493=DIRECTION('center_axis',(0.,0.,1.));
#30494=DIRECTION('ref_axis',(1.,-1.07699989592456E-13,0.));
#30495=DIRECTION('',(0.,0.,1.));
#30496=DIRECTION('center_axis',(0.,0.,1.));
#30497=DIRECTION('ref_axis',(1.,-1.07699989592456E-13,0.));
#30498=DIRECTION('',(0.,0.,1.));
#30499=DIRECTION('center_axis',(0.,0.,1.));
#30500=DIRECTION('ref_axis',(1.,-1.07699989592456E-13,0.));
#30501=DIRECTION('',(0.,0.,1.));
#30502=DIRECTION('center_axis',(0.,0.,1.));
#30503=DIRECTION('ref_axis',(1.,-1.07699989592456E-13,0.));
#30504=DIRECTION('',(0.,0.,1.));
#30505=DIRECTION('center_axis',(0.,0.,1.));
#30506=DIRECTION('ref_axis',(1.,-1.07699989592456E-13,0.));
#30507=DIRECTION('',(0.,0.,1.));
#30508=DIRECTION('center_axis',(0.,0.,1.));
#30509=DIRECTION('ref_axis',(1.,-1.07699989592456E-13,0.));
#30510=DIRECTION('',(0.,0.,1.));
#30511=DIRECTION('center_axis',(0.,0.,1.));
#30512=DIRECTION('ref_axis',(1.,-1.07699989592456E-13,0.));
#30513=DIRECTION('',(0.,0.,1.));
#30514=DIRECTION('center_axis',(0.,0.,1.));
#30515=DIRECTION('ref_axis',(1.,-1.07699989592456E-13,0.));
#30516=DIRECTION('',(0.,0.,1.));
#30517=DIRECTION('center_axis',(0.,0.,1.));
#30518=DIRECTION('ref_axis',(1.,-1.07699989592456E-13,0.));
#30519=DIRECTION('',(0.,0.,1.));
#30520=DIRECTION('center_axis',(0.,0.,1.));
#30521=DIRECTION('ref_axis',(1.,-1.07699989592456E-13,0.));
#30522=DIRECTION('',(0.,0.,1.));
#30523=DIRECTION('center_axis',(0.,0.,1.));
#30524=DIRECTION('ref_axis',(1.,-1.07699989592456E-13,0.));
#30525=DIRECTION('',(0.,0.,1.));
#30526=DIRECTION('center_axis',(0.,0.,1.));
#30527=DIRECTION('ref_axis',(1.,-1.07699989592456E-13,0.));
#30528=DIRECTION('',(0.,0.,1.));
#30529=DIRECTION('center_axis',(0.,0.,1.));
#30530=DIRECTION('ref_axis',(1.,-1.07699989592456E-13,0.));
#30531=DIRECTION('',(0.,0.,1.));
#30532=DIRECTION('center_axis',(0.,0.,1.));
#30533=DIRECTION('ref_axis',(1.,-1.07699989592456E-13,0.));
#30534=DIRECTION('',(0.,0.,1.));
#30535=DIRECTION('center_axis',(0.,0.,1.));
#30536=DIRECTION('ref_axis',(1.,-1.07699989592456E-13,0.));
#30537=DIRECTION('',(0.,0.,1.));
#30538=DIRECTION('center_axis',(0.,0.,1.));
#30539=DIRECTION('ref_axis',(1.,-1.07699989592456E-13,0.));
#30540=DIRECTION('',(0.,0.,1.));
#30541=DIRECTION('center_axis',(0.,0.,1.));
#30542=DIRECTION('ref_axis',(1.,-1.07699989592456E-13,0.));
#30543=DIRECTION('',(0.,0.,1.));
#30544=DIRECTION('center_axis',(0.,0.,1.));
#30545=DIRECTION('ref_axis',(1.,-1.07699989592456E-13,0.));
#30546=DIRECTION('',(0.,0.,1.));
#30547=DIRECTION('center_axis',(0.,0.,1.));
#30548=DIRECTION('ref_axis',(1.,-1.07699989592456E-13,0.));
#30549=DIRECTION('',(0.,0.,1.));
#30550=DIRECTION('center_axis',(0.,0.,1.));
#30551=DIRECTION('ref_axis',(1.,-1.07699989592456E-13,0.));
#30552=DIRECTION('',(0.,0.,1.));
#30553=DIRECTION('center_axis',(0.,0.,1.));
#30554=DIRECTION('ref_axis',(1.,-1.07699989592456E-13,0.));
#30555=DIRECTION('',(0.,0.,1.));
#30556=DIRECTION('center_axis',(0.,0.,1.));
#30557=DIRECTION('ref_axis',(1.,-1.07699989592456E-13,0.));
#30558=DIRECTION('',(0.,0.,1.));
#30559=DIRECTION('center_axis',(0.,0.,1.));
#30560=DIRECTION('ref_axis',(1.,-1.07699989592456E-13,0.));
#30561=DIRECTION('',(0.,0.,1.));
#30562=DIRECTION('center_axis',(0.,0.,1.));
#30563=DIRECTION('ref_axis',(1.,-1.07699989592456E-13,0.));
#30564=DIRECTION('',(0.,0.,1.));
#30565=DIRECTION('center_axis',(0.,0.,1.));
#30566=DIRECTION('ref_axis',(1.,-1.07699989592456E-13,0.));
#30567=DIRECTION('',(0.,0.,1.));
#30568=DIRECTION('center_axis',(0.,0.,1.));
#30569=DIRECTION('ref_axis',(1.,-1.07699989592456E-13,0.));
#30570=DIRECTION('',(0.,0.,1.));
#30571=DIRECTION('center_axis',(0.,0.,1.));
#30572=DIRECTION('ref_axis',(1.,-1.07699989592456E-13,0.));
#30573=DIRECTION('',(0.,0.,1.));
#30574=DIRECTION('center_axis',(0.,0.,1.));
#30575=DIRECTION('ref_axis',(1.,0.,0.));
#30576=DIRECTION('center_axis',(0.,0.,-1.));
#30577=DIRECTION('ref_axis',(1.,0.,0.));
#30578=DIRECTION('center_axis',(0.,0.,-1.));
#30579=DIRECTION('ref_axis',(1.,0.,0.));
#30580=DIRECTION('center_axis',(0.,0.,1.));
#30581=DIRECTION('ref_axis',(1.,0.,0.));
#30582=DIRECTION('center_axis',(0.,0.,1.));
#30583=DIRECTION('ref_axis',(1.,0.,0.));
#30584=DIRECTION('center_axis',(0.,0.,1.));
#30585=DIRECTION('ref_axis',(1.,0.,0.));
#30586=DIRECTION('center_axis',(0.,0.,-1.));
#30587=DIRECTION('ref_axis',(1.,-1.07699989592456E-13,0.));
#30588=DIRECTION('center_axis',(0.,0.,1.));
#30589=DIRECTION('ref_axis',(0.888987032667973,0.457932370277743,0.));
#30590=DIRECTION('center_axis',(0.,0.,1.));
#30591=DIRECTION('ref_axis',(1.,0.,0.));
#30592=DIRECTION('',(-1.,2.40370335797945E-16,0.));
#30593=DIRECTION('center_axis',(0.,0.,1.));
#30594=DIRECTION('ref_axis',(1.,0.,0.));
#30595=DIRECTION('center_axis',(0.,0.,1.));
#30596=DIRECTION('ref_axis',(1.,0.,0.));
#30597=DIRECTION('',(-0.5,0.866025403784439,0.));
#30598=DIRECTION('center_axis',(0.,0.,1.));
#30599=DIRECTION('ref_axis',(1.,0.,0.));
#30600=DIRECTION('center_axis',(0.,0.,1.));
#30601=DIRECTION('ref_axis',(1.,0.,0.));
#30602=DIRECTION('',(0.5,0.866025403784439,0.));
#30603=DIRECTION('center_axis',(0.,0.,1.));
#30604=DIRECTION('ref_axis',(1.,0.,0.));
#30605=DIRECTION('center_axis',(0.,0.,1.));
#30606=DIRECTION('ref_axis',(1.,0.,0.));
#30607=DIRECTION('',(1.,-1.20185167898973E-16,0.));
#30608=DIRECTION('center_axis',(0.,0.,1.));
#30609=DIRECTION('ref_axis',(1.,0.,0.));
#30610=DIRECTION('center_axis',(0.,0.,1.));
#30611=DIRECTION('ref_axis',(1.,0.,0.));
#30612=DIRECTION('',(0.5,-0.866025403784439,0.));
#30613=DIRECTION('center_axis',(0.,0.,1.));
#30614=DIRECTION('ref_axis',(1.,0.,0.));
#30615=DIRECTION('center_axis',(0.,0.,1.));
#30616=DIRECTION('ref_axis',(1.,0.,0.));
#30617=DIRECTION('',(-0.5,-0.866025403784439,0.));
#30618=DIRECTION('center_axis',(0.,0.,1.));
#30619=DIRECTION('ref_axis',(1.,0.,0.));
#30620=DIRECTION('center_axis',(0.,0.,1.));
#30621=DIRECTION('ref_axis',(1.,0.,0.));
#30622=DIRECTION('',(-0.856673567959776,-1.04912254291608E-16,0.515858893457375));
#30623=DIRECTION('center_axis',(0.,0.,-1.));
#30624=DIRECTION('ref_axis',(1.,0.,0.));
#30625=DIRECTION('center_axis',(0.,0.,-1.));
#30626=DIRECTION('ref_axis',(1.,0.,0.));
#30627=DIRECTION('center_axis',(0.,0.,-1.));
#30628=DIRECTION('ref_axis',(1.,0.,0.));
#30629=DIRECTION('center_axis',(0.,0.,-1.));
#30630=DIRECTION('ref_axis',(1.,0.,0.));
#30631=DIRECTION('center_axis',(0.,0.,-1.));
#30632=DIRECTION('ref_axis',(1.,0.,0.));
#30633=DIRECTION('center_axis',(0.,0.,-1.));
#30634=DIRECTION('ref_axis',(1.,0.,0.));
#30635=DIRECTION('center_axis',(0.,0.,-1.));
#30636=DIRECTION('ref_axis',(1.,0.,0.));
#30637=DIRECTION('center_axis',(-0.866025403784439,0.5,0.));
#30638=DIRECTION('ref_axis',(0.5,0.866025403784439,0.));
#30639=DIRECTION('',(0.,0.,-1.));
#30640=DIRECTION('',(0.5,0.866025403784439,0.));
#30641=DIRECTION('',(0.,0.,-1.));
#30642=DIRECTION('center_axis',(-0.866025403784439,0.5,0.));
#30643=DIRECTION('ref_axis',(0.5,0.866025403784439,0.));
#30644=DIRECTION('',(0.,0.,-1.));
#30645=DIRECTION('',(0.5,0.866025403784439,0.));
#30646=DIRECTION('center_axis',(1.20185167898973E-16,1.,0.));
#30647=DIRECTION('ref_axis',(1.,-1.20185167898973E-16,0.));
#30648=DIRECTION('',(0.,0.,-1.));
#30649=DIRECTION('',(1.,-1.20185167898973E-16,0.));
#30650=DIRECTION('center_axis',(1.20185167898973E-16,1.,0.));
#30651=DIRECTION('ref_axis',(1.,-1.20185167898973E-16,0.));
#30652=DIRECTION('',(1.,-1.20185167898973E-16,0.));
#30653=DIRECTION('',(0.,0.,-1.));
#30654=DIRECTION('center_axis',(1.20185167898973E-16,1.,0.));
#30655=DIRECTION('ref_axis',(1.,-1.20185167898973E-16,0.));
#30656=DIRECTION('',(0.,0.,-1.));
#30657=DIRECTION('',(1.,-1.20185167898973E-16,0.));
#30658=DIRECTION('center_axis',(-0.866025403784439,-0.5,0.));
#30659=DIRECTION('ref_axis',(-0.5,0.866025403784439,0.));
#30660=DIRECTION('',(-0.5,0.866025403784439,0.));
#30661=DIRECTION('',(0.,0.,-1.));
#30662=DIRECTION('center_axis',(-0.866025403784439,-0.5,0.));
#30663=DIRECTION('ref_axis',(-0.5,0.866025403784439,0.));
#30664=DIRECTION('',(0.,0.,-1.));
#30665=DIRECTION('',(-0.5,0.866025403784439,0.));
#30666=DIRECTION('center_axis',(0.866025403784439,0.5,0.));
#30667=DIRECTION('ref_axis',(0.5,-0.866025403784439,0.));
#30668=DIRECTION('',(0.,0.,-1.));
#30669=DIRECTION('',(0.5,-0.866025403784439,0.));
#30670=DIRECTION('center_axis',(0.866025403784439,0.5,0.));
#30671=DIRECTION('ref_axis',(0.5,-0.866025403784439,0.));
#30672=DIRECTION('',(0.5,-0.866025403784439,0.));
#30673=DIRECTION('',(0.,0.,-1.));
#30674=DIRECTION('center_axis',(0.866025403784439,0.5,0.));
#30675=DIRECTION('ref_axis',(0.5,-0.866025403784439,0.));
#30676=DIRECTION('',(0.5,-0.866025403784439,0.));
#30677=DIRECTION('center_axis',(0.,0.,-1.));
#30678=DIRECTION('ref_axis',(-1.,0.,0.));
#30679=DIRECTION('',(0.5,0.866025403784439,0.));
#30680=DIRECTION('center_axis',(0.,0.,-1.));
#30681=DIRECTION('ref_axis',(-1.,0.,0.));
#30682=DIRECTION('center_axis',(0.,0.,-1.));
#30683=DIRECTION('ref_axis',(-1.,0.,0.));
#30684=DIRECTION('',(-0.5,-0.866025403784439,0.));
#30685=DIRECTION('center_axis',(0.,0.,-1.));
#30686=DIRECTION('ref_axis',(-1.,0.,0.));
#30687=DIRECTION('',(-1.,2.40370335797945E-16,0.));
#30688=DIRECTION('',(-0.5,-0.866025403784439,0.));
#30689=DIRECTION('center_axis',(0.,0.,-1.));
#30690=DIRECTION('ref_axis',(-1.,0.,0.));
#30691=DIRECTION('',(-1.,2.40370335797945E-16,0.));
#30692=DIRECTION('center_axis',(0.,0.,-1.));
#30693=DIRECTION('ref_axis',(-1.,0.,0.));
#30694=DIRECTION('',(-0.5,0.866025403784439,0.));
#30695=DIRECTION('center_axis',(0.866025403784439,-0.5,0.));
#30696=DIRECTION('ref_axis',(-0.5,-0.866025403784439,0.));
#30697=DIRECTION('',(0.,0.,-1.));
#30698=DIRECTION('',(-0.5,-0.866025403784439,0.));
#30699=DIRECTION('center_axis',(0.866025403784439,-0.5,0.));
#30700=DIRECTION('ref_axis',(-0.5,-0.866025403784439,0.));
#30701=DIRECTION('',(0.,0.,-1.));
#30702=DIRECTION('center_axis',(0.866025403784439,-0.5,0.));
#30703=DIRECTION('ref_axis',(-0.5,-0.866025403784439,0.));
#30704=DIRECTION('center_axis',(-2.40370335797945E-16,-1.,0.));
#30705=DIRECTION('ref_axis',(-1.,2.40370335797945E-16,0.));
#30706=DIRECTION('center_axis',(-2.40370335797945E-16,-1.,0.));
#30707=DIRECTION('ref_axis',(-1.,2.40370335797945E-16,0.));
#30708=DIRECTION('',(-1.,2.40370335797945E-16,0.));
#30709=DIRECTION('center_axis',(-0.866025403784439,0.5,0.));
#30710=DIRECTION('ref_axis',(0.5,0.866025403784439,0.));
#30711=DIRECTION('center_axis',(-0.866025403784439,-0.5,0.));
#30712=DIRECTION('ref_axis',(-0.5,0.866025403784439,0.));
#30713=DIRECTION('center_axis',(-2.40370335797945E-16,-1.,0.));
#30714=DIRECTION('ref_axis',(-1.,2.40370335797945E-16,0.));
#30715=DIRECTION('center_axis',(0.,0.,-1.));
#30716=DIRECTION('ref_axis',(-1.,0.,0.));
#30717=DIRECTION('center_axis',(0.,0.,1.));
#30718=DIRECTION('ref_axis',(1.,0.,0.));
#30719=DIRECTION('center_axis',(0.,0.,1.));
#30720=DIRECTION('ref_axis',(1.,0.,0.));
#30721=DIRECTION('',(0.707106781186547,8.65956056235493E-17,-0.707106781186548));
#30722=DIRECTION('center_axis',(0.,0.,1.));
#30723=DIRECTION('ref_axis',(0.0319324370611075,-0.999490029696814,0.));
#30724=DIRECTION('center_axis',(0.,0.,-1.));
#30725=DIRECTION('ref_axis',(1.,0.,0.));
#30726=DIRECTION('center_axis',(0.,0.,-1.));
#30727=DIRECTION('ref_axis',(1.,0.,0.));
#30728=DIRECTION('center_axis',(0.,0.,1.));
#30729=DIRECTION('ref_axis',(1.,0.,0.));
#30730=DIRECTION('',(-0.707106781186548,-8.65956056235494E-17,-0.707106781186547));
#30731=DIRECTION('center_axis',(0.,0.,1.));
#30732=DIRECTION('ref_axis',(1.,0.,0.));
#47588=CARTESIAN_POINT('',(0.,0.,0.));
#47589=CARTESIAN_POINT('Origin',(0.,0.,-2.94));
#47590=CARTESIAN_POINT('',(-0.791106180021776,2.03161438686317E-5,-5.74466684917629));
#47591=CARTESIAN_POINT('',(-0.791090782287945,1.29766800149628E-5,-5.7731331508237));
#47592=CARTESIAN_POINT('',(-0.7911,-9.68818082805471E-17,-2.94));
#47593=CARTESIAN_POINT('',(0.342081922270278,0.713331522816647,-5.8089));
#47594=CARTESIAN_POINT('Ctrl Pts',(-0.791106180021776,2.03161438686317E-5,
-5.74466684917629));
#47595=CARTESIAN_POINT('Ctrl Pts',(-0.791135343475079,0.0283677424344691,
-5.74580749484678));
#47596=CARTESIAN_POINT('Ctrl Pts',(-0.789641156878406,0.0567121003347207,
-5.74694814051726));
#47597=CARTESIAN_POINT('Ctrl Pts',(-0.786600263288403,0.0848895237920406,
-5.74808878618774));
#47598=CARTESIAN_POINT('Ctrl Pts',(-0.772508536262909,0.215465799445913,
-5.75337462304639));
#47599=CARTESIAN_POINT('Ctrl Pts',(-0.725201825327082,0.342457217166145,
-5.75866045990504));
#47600=CARTESIAN_POINT('Ctrl Pts',(-0.650430093527711,0.450429424087558,
-5.76394629676369));
#47601=CARTESIAN_POINT('Ctrl Pts',(-0.57565836172834,0.558401631008971,
-5.76923213362234));
#47602=CARTESIAN_POINT('Ctrl Pts',(-0.473421609065425,0.647354627131565,
-5.77451797048098));
#47603=CARTESIAN_POINT('Ctrl Pts',(-0.356146177440628,0.70647482914802,
-5.77980380733963));
#47604=CARTESIAN_POINT('Ctrl Pts',(-0.238870745815832,0.765595031164475,
-5.78508964419828));
#47605=CARTESIAN_POINT('Ctrl Pts',(-0.106556635229153,0.794882439074792,
-5.79037548105694));
#47606=CARTESIAN_POINT('Ctrl Pts',(0.0247138000160614,0.790780700517692,
-5.79566131791558));
#47607=CARTESIAN_POINT('Ctrl Pts',(0.134305248873851,0.787356353897155,
-5.80007421194372));
#47608=CARTESIAN_POINT('Ctrl Pts',(0.243169278281288,0.760660484412965,
-5.80448710597186));
#47609=CARTESIAN_POINT('Ctrl Pts',(0.342095882030774,0.713340734875802,
-5.8089));
#47610=CARTESIAN_POINT('',(-0.342067962509742,0.71332231075751,-5.8089));
#47611=CARTESIAN_POINT('Origin',(0.,0.,-5.8089));
#47612=CARTESIAN_POINT('Ctrl Pts',(-0.342067962509741,0.71332231075751,
-5.8089));
#47613=CARTESIAN_POINT('Ctrl Pts',(-0.460521881974901,0.656518688787926,
-5.80361416314135));
#47614=CARTESIAN_POINT('Ctrl Pts',(-0.564494897987404,0.569670406071105,
-5.79832832628271));
#47615=CARTESIAN_POINT('Ctrl Pts',(-0.641387916838763,0.463218315988371,
-5.79304248942406));
#47616=CARTESIAN_POINT('Ctrl Pts',(-0.718280935690122,0.356766225905636,
-5.78775665256541));
#47617=CARTESIAN_POINT('Ctrl Pts',(-0.768093957380336,0.230710328456987,
-5.78247081570676));
#47618=CARTESIAN_POINT('Ctrl Pts',(-0.784767319259172,0.100431910373907,
-5.77718497884811));
#47619=CARTESIAN_POINT('Ctrl Pts',(-0.789027609334232,0.0671438515176777,
-5.77583436950664));
#47620=CARTESIAN_POINT('Ctrl Pts',(-0.791124284156975,0.0335801136080157,
-5.77448376016517));
#47621=CARTESIAN_POINT('Ctrl Pts',(-0.791090782287945,1.29766800149628E-5,
-5.7731331508237));
#47622=CARTESIAN_POINT('Origin',(0.,0.,-2.94));
#47623=CARTESIAN_POINT('',(-0.791124235703911,-1.85398115769009E-5,-5.5446668491763));
#47624=CARTESIAN_POINT('',(-0.791139506632643,-1.5767809539321E-5,-5.5731331508237));
#47625=CARTESIAN_POINT('',(-0.7911,-9.68818082805471E-17,-2.94));
#47626=CARTESIAN_POINT('Ctrl Pts',(-0.791124235703911,-1.85398115769009E-5,
-5.5446668491763));
#47627=CARTESIAN_POINT('Ctrl Pts',(-0.791015771065361,0.108758589208093,
-5.54904411920968));
#47628=CARTESIAN_POINT('Ctrl Pts',(-0.768397083456412,0.21757942619962,
-5.55342138924305));
#47629=CARTESIAN_POINT('Ctrl Pts',(-0.724790381405401,0.31721456737946,
-5.55779865927643));
#47630=CARTESIAN_POINT('Ctrl Pts',(-0.672132466488617,0.437530448659187,
-5.56308449613507));
#47631=CARTESIAN_POINT('Ctrl Pts',(-0.588869565491455,0.54445163301647,
-5.56837033299372));
#47632=CARTESIAN_POINT('Ctrl Pts',(-0.485121914936739,0.62498232476536,
-5.57365616985236));
#47633=CARTESIAN_POINT('Ctrl Pts',(-0.381374264382023,0.705513016514249,
-5.57894200671101));
#47634=CARTESIAN_POINT('Ctrl Pts',(-0.257141864269753,0.759653215654744,
-5.58422784356967));
#47635=CARTESIAN_POINT('Ctrl Pts',(-0.127524612081043,0.780822420424087,
-5.58951368042832));
#47636=CARTESIAN_POINT('Ctrl Pts',(0.00209264010766494,0.801991625193429,
-5.59479951728696));
#47637=CARTESIAN_POINT('Ctrl Pts',(0.137094744372813,0.79018983559162,-5.60008535414561));
#47638=CARTESIAN_POINT('Ctrl Pts',(0.261072793357542,0.746851507925876,
-5.60537119100425));
#47639=CARTESIAN_POINT('Ctrl Pts',(0.385050842342272,0.703513180260131,
-5.6106570278629));
#47640=CARTESIAN_POINT('Ctrl Pts',(0.498004836046584,0.628638314530449,
-5.61594286472155));
#47641=CARTESIAN_POINT('Ctrl Pts',(0.586205717365502,0.531327616596799,
-5.6212287015802));
#47642=CARTESIAN_POINT('Ctrl Pts',(0.674406598684419,0.434016918663149,
-5.62651453843885));
#47643=CARTESIAN_POINT('Ctrl Pts',(0.737854367617943,0.314270388525531,
-5.63180037529749));
#47644=CARTESIAN_POINT('Ctrl Pts',(0.768837228920146,0.186642690276987,
-5.63708621215614));
#47645=CARTESIAN_POINT('Ctrl Pts',(0.799820090222349,0.0590149920284431,
-5.64237204901479));
#47646=CARTESIAN_POINT('Ctrl Pts',(0.798338043893232,-0.0764938743310262,
-5.64765788587344));
#47647=CARTESIAN_POINT('Ctrl Pts',(0.764571226480889,-0.203413415006452,
-5.65294372273209));
#47648=CARTESIAN_POINT('Ctrl Pts',(0.730804409068546,-0.330332955681878,
-5.65822955959074));
#47649=CARTESIAN_POINT('Ctrl Pts',(0.664752820572977,-0.44866317067326,
-5.66351539644938));
#47650=CARTESIAN_POINT('Ctrl Pts',(0.574444738011475,-0.544021530895698,
-5.66880123330803));
#47651=CARTESIAN_POINT('Ctrl Pts',(0.484136655449973,-0.639379891118138,
-5.67408707016667));
#47652=CARTESIAN_POINT('Ctrl Pts',(0.369572078822538,-0.711766396571634,
-5.67937290702533));
#47653=CARTESIAN_POINT('Ctrl Pts',(0.244675826026431,-0.752382819699385,
-5.68465874388398));
#47654=CARTESIAN_POINT('Ctrl Pts',(0.119779573230324,-0.792999242827135,
-5.68994458074262));
#47655=CARTESIAN_POINT('Ctrl Pts',(-0.0154483557344541,-0.80184558362914,
-5.69523041760127));
#47656=CARTESIAN_POINT('Ctrl Pts',(-0.144571608456504,-0.777846547461446,
-5.70051625445991));
#47657=CARTESIAN_POINT('Ctrl Pts',(-0.273694861178554,-0.753847511293753,
-5.70580209131856));
#47658=CARTESIAN_POINT('Ctrl Pts',(-0.396713437657876,-0.69700309815636,
-5.71108792817721));
#47659=CARTESIAN_POINT('Ctrl Pts',(-0.49867496963204,-0.614222613923978,
-5.71637376503586));
#47660=CARTESIAN_POINT('Ctrl Pts',(-0.600636501606204,-0.531442129691597,
-5.72165960189451));
#47661=CARTESIAN_POINT('Ctrl Pts',(-0.681540989075211,-0.422725574364226,
-5.72694543875316));
#47662=CARTESIAN_POINT('Ctrl Pts',(-0.731554861252135,-0.301286729906785,
-5.7322312756118));
#47663=CARTESIAN_POINT('Ctrl Pts',(-0.770776098641365,-0.206053516811625,
-5.73637646679997));
#47664=CARTESIAN_POINT('Ctrl Pts',(-0.791000197863794,-0.102996338990715,
-5.74052165798813));
#47665=CARTESIAN_POINT('Ctrl Pts',(-0.791106180021776,2.03161438686317E-5,
-5.74466684917629));
#47666=CARTESIAN_POINT('Ctrl Pts',(-0.791090782287945,1.29766800149628E-5,
-5.7731331508237));
#47667=CARTESIAN_POINT('Ctrl Pts',(-0.790993168956811,-0.0977905234557233,
-5.76919792330652));
#47668=CARTESIAN_POINT('Ctrl Pts',(-0.772811500478589,-0.195622879430191,
-5.76526269578935));
#47669=CARTESIAN_POINT('Ctrl Pts',(-0.737372895602027,-0.286749114669279,
-5.76132746827217));
#47670=CARTESIAN_POINT('Ctrl Pts',(-0.68977140799859,-0.409150782911872,
-5.75604163141353));
#47671=CARTESIAN_POINT('Ctrl Pts',(-0.61103473072426,-0.519453180679546,
-5.75075579455488));
#47672=CARTESIAN_POINT('Ctrl Pts',(-0.510731350947639,-0.604236529687556,
-5.74546995769623));
#47673=CARTESIAN_POINT('Ctrl Pts',(-0.410427971171018,-0.689019878695568,
-5.74018412083758));
#47674=CARTESIAN_POINT('Ctrl Pts',(-0.288557888892106,-0.748284178943916,
-5.73489828397893));
#47675=CARTESIAN_POINT('Ctrl Pts',(-0.159934698591644,-0.774832740239663,
-5.72961244712028));
#47676=CARTESIAN_POINT('Ctrl Pts',(-0.0313115082911817,-0.801381301535411,
-5.72432661026163));
#47677=CARTESIAN_POINT('Ctrl Pts',(0.10406479003083,-0.795214123878558,
-5.71904077340299));
#47678=CARTESIAN_POINT('Ctrl Pts',(0.229740230761185,-0.757077413481008,
-5.71375493654434));
#47679=CARTESIAN_POINT('Ctrl Pts',(0.355415671491541,-0.718940703083458,
-5.70846909968569));
#47680=CARTESIAN_POINT('Ctrl Pts',(0.471390254630239,-0.648834459945212,
-5.70318326282704));
#47681=CARTESIAN_POINT('Ctrl Pts',(0.563567566968777,-0.555281520687494,
-5.6978974259684));
#47682=CARTESIAN_POINT('Ctrl Pts',(0.655744879307314,-0.461728581429777,
-5.69261158910975));
#47683=CARTESIAN_POINT('Ctrl Pts',(0.72412492084569,-0.344728946052588,
-5.6873257522511));
#47684=CARTESIAN_POINT('Ctrl Pts',(0.760396511630209,-0.218502514129848,
-5.68203991539245));
#47685=CARTESIAN_POINT('Ctrl Pts',(0.796668102414727,-0.0922760822071087,
-5.6767540785338));
#47686=CARTESIAN_POINT('Ctrl Pts',(0.800831242445389,0.0431771462611828,
-5.67146824167516));
#47687=CARTESIAN_POINT('Ctrl Pts',(0.772379863699283,0.171392977507774,
-5.66618240481651));
#47688=CARTESIAN_POINT('Ctrl Pts',(0.743928484953178,0.299608808754365,
-5.66089656795786));
#47689=CARTESIAN_POINT('Ctrl Pts',(0.682862587430305,0.420587242779256,
-5.65561073109921));
#47690=CARTESIAN_POINT('Ctrl Pts',(0.59660448934969,0.519624119809878,-5.65032489424056));
#47691=CARTESIAN_POINT('Ctrl Pts',(0.510346391269075,0.618660996840501,
-5.64503905738192));
#47692=CARTESIAN_POINT('Ctrl Pts',(0.398896092630719,0.695756316876854,
-5.63975322052327));
#47693=CARTESIAN_POINT('Ctrl Pts',(0.275799868283255,0.741539366466232,
-5.63446738366463));
#47694=CARTESIAN_POINT('Ctrl Pts',(0.152703643935791,0.787322416055611,
-5.62918154680598));
#47695=CARTESIAN_POINT('Ctrl Pts',(0.0179614938792174,0.801793195198013,
-5.62389570994733));
#47696=CARTESIAN_POINT('Ctrl Pts',(-0.112049263241192,0.78319290579391,
-5.61860987308868));
#47697=CARTESIAN_POINT('Ctrl Pts',(-0.242060020361602,0.764592616389807,
-5.61332403623003));
#47698=CARTESIAN_POINT('Ctrl Pts',(-0.36733938454585,0.712921258439198,
-5.60803819937139));
#47699=CARTESIAN_POINT('Ctrl Pts',(-0.472660208346534,0.634459225234524,
-5.60275236251274));
#47700=CARTESIAN_POINT('Ctrl Pts',(-0.577981032147217,0.555997192029851,
-5.59746652565409));
#47701=CARTESIAN_POINT('Ctrl Pts',(-0.663343315564336,0.450744483571114,
-5.59218068879544));
#47702=CARTESIAN_POINT('Ctrl Pts',(-0.718371649464549,0.331494115958518,
-5.58689485193679));
#47703=CARTESIAN_POINT('Ctrl Pts',(-0.766127158140359,0.228004485045039,
-5.58230761823243));
#47704=CARTESIAN_POINT('Ctrl Pts',(-0.791037034503848,0.11397269330664,
-5.57772038452807));
#47705=CARTESIAN_POINT('Ctrl Pts',(-0.791139506632643,-1.5767809539321E-5,
-5.5731331508237));
#47706=CARTESIAN_POINT('Origin',(0.,0.,-2.94));
#47707=CARTESIAN_POINT('',(-0.791036503466522,7.11594896907197E-6,-5.3446668491763));
#47708=CARTESIAN_POINT('',(-0.791033090718594,2.41426438800759E-6,-5.3731331508237));
#47709=CARTESIAN_POINT('',(-0.7911,-9.68818082805471E-17,-2.94));
#47710=CARTESIAN_POINT('Ctrl Pts',(-0.791036503466522,7.11594896907197E-6,
-5.3446668491763));
#47711=CARTESIAN_POINT('Ctrl Pts',(-0.791054774529985,0.0578788267958651,
-5.34699490671392));
#47712=CARTESIAN_POINT('Ctrl Pts',(-0.784789673957966,0.115746641424242,
-5.34932296425154));
#47713=CARTESIAN_POINT('Ctrl Pts',(-0.772199447682732,0.172203924778507,
-5.35165102178916));
#47714=CARTESIAN_POINT('Ctrl Pts',(-0.743613435082568,0.300389755442302,
-5.35693685864781));
#47715=CARTESIAN_POINT('Ctrl Pts',(-0.682420541996382,0.421304106164855,
-5.36222269550646));
#47716=CARTESIAN_POINT('Ctrl Pts',(-0.596058493308848,0.520250373632772,
-5.3675085323651));
#47717=CARTESIAN_POINT('Ctrl Pts',(-0.509696444621315,0.619196641100689,
-5.37279436922375));
#47718=CARTESIAN_POINT('Ctrl Pts',(-0.398165240332434,0.69617482531397,
-5.3780802060824));
#47719=CARTESIAN_POINT('Ctrl Pts',(-0.275021003902314,0.741828569228208,
-5.38336604294105));
#47720=CARTESIAN_POINT('Ctrl Pts',(-0.151876767472194,0.787482313142446,
-5.3886518797997));
#47721=CARTESIAN_POINT('Ctrl Pts',(-0.0171194989008363,0.801811616757642,
-5.39393771665834));
#47722=CARTESIAN_POINT('Ctrl Pts',(0.112871653199976,0.783074816741423,
-5.39922355351699));
#47723=CARTESIAN_POINT('Ctrl Pts',(0.24286280530079,0.764338016725204,-5.40450939037564));
#47724=CARTESIAN_POINT('Ctrl Pts',(0.368087840931059,0.712535113077569,
-5.40979522723429));
#47725=CARTESIAN_POINT('Ctrl Pts',(0.473326212136283,0.633962519093404,
-5.41508106409294));
#47726=CARTESIAN_POINT('Ctrl Pts',(0.578564583341508,0.555389925109238,
-5.42036690095158));
#47727=CARTESIAN_POINT('Ctrl Pts',(0.663816290121689,0.450047640788541,
-5.42565273781023));
#47728=CARTESIAN_POINT('Ctrl Pts',(0.718719365441129,0.33073955380426,-5.43093857466888));
#47729=CARTESIAN_POINT('Ctrl Pts',(0.773622440760568,0.211431466819979,
-5.43622441152752));
#47730=CARTESIAN_POINT('Ctrl Pts',(0.798176884619266,0.078157577172114,
-5.44151024838617));
#47731=CARTESIAN_POINT('Ctrl Pts',(0.789398213216727,-0.052883264658473,
-5.44679608524482));
#47732=CARTESIAN_POINT('Ctrl Pts',(0.780619541814188,-0.18392410648906,
-5.45208192210347));
#47733=CARTESIAN_POINT('Ctrl Pts',(0.738507755150412,-0.312731900502369,
-5.45736775896212));
#47734=CARTESIAN_POINT('Ctrl Pts',(0.66818135421168,-0.423650630347585,
-5.46265359582076));
#47735=CARTESIAN_POINT('Ctrl Pts',(0.597854953272949,-0.5345693601928,-5.46793943267941));
#47736=CARTESIAN_POINT('Ctrl Pts',(0.499313938059263,-0.627599025869922,
-5.47322526953806));
#47737=CARTESIAN_POINT('Ctrl Pts',(0.384535532134293,-0.691432283914052,
-5.47851110639671));
#47738=CARTESIAN_POINT('Ctrl Pts',(0.269757126209322,-0.755265541958182,
-5.48379694325536));
#47739=CARTESIAN_POINT('Ctrl Pts',(0.138741329573066,-0.789902392369319,
-5.489082780114));
#47740=CARTESIAN_POINT('Ctrl Pts',(0.00741253151014375,-0.791132879536305,
-5.49436861697265));
#47741=CARTESIAN_POINT('Ctrl Pts',(-0.123916266552779,-0.792363366703291,
-5.4996544538313));
#47742=CARTESIAN_POINT('Ctrl Pts',(-0.255558066042368,-0.760187490626126,
-5.50494029068995));
#47743=CARTESIAN_POINT('Ctrl Pts',(-0.371512389803684,-0.698516086385605,
-5.5102261275486));
#47744=CARTESIAN_POINT('Ctrl Pts',(-0.487466713564998,-0.636844682145085,
-5.51551196440724));
#47745=CARTESIAN_POINT('Ctrl Pts',(-0.587733561598039,-0.545677749741209,
-5.52079780126589));
#47746=CARTESIAN_POINT('Ctrl Pts',(-0.660125943008546,-0.436096225700483,
-5.52608363812454));
#47747=CARTESIAN_POINT('Ctrl Pts',(-0.732518324419053,-0.326514701659758,
-5.53136947498318));
#47748=CARTESIAN_POINT('Ctrl Pts',(-0.777036239207025,-0.198518585982181,
-5.53665531184184));
#47749=CARTESIAN_POINT('Ctrl Pts',(-0.788268732182809,-0.0676652390423088,
-5.54194114870048));
#47750=CARTESIAN_POINT('Ctrl Pts',(-0.790199452096383,-0.0451732452133963,
-5.54284971552576));
#47751=CARTESIAN_POINT('Ctrl Pts',(-0.791146749136153,-0.0225968340502242,
-5.54375828235103));
#47752=CARTESIAN_POINT('Ctrl Pts',(-0.791124235703911,-1.85398115769009E-5,
-5.5446668491763));
#47753=CARTESIAN_POINT('Ctrl Pts',(-0.791139506632643,-1.5767809539321E-5,
-5.5731331508237));
#47754=CARTESIAN_POINT('Ctrl Pts',(-0.791155112410987,-0.017375401876565,
-5.57243454766942));
#47755=CARTESIAN_POINT('Ctrl Pts',(-0.790595356852504,-0.0347340309708619,
-5.57173594451514));
#47756=CARTESIAN_POINT('Ctrl Pts',(-0.789453310686279,-0.0520542655584215,
-5.57103734136085));
#47757=CARTESIAN_POINT('Ctrl Pts',(-0.780812253624487,-0.183104252696313,
-5.5657515045022));
#47758=CARTESIAN_POINT('Ctrl Pts',(-0.738835755117596,-0.311956200205645,
-5.56046566764355));
#47759=CARTESIAN_POINT('Ctrl Pts',(-0.668625871952495,-0.422948720884337,
-5.5551798307849));
#47760=CARTESIAN_POINT('Ctrl Pts',(-0.598415988787394,-0.533941241563029,
-5.54989399392626));
#47761=CARTESIAN_POINT('Ctrl Pts',(-0.499972720964085,-0.627074335411082,
-5.54460815706761));
#47762=CARTESIAN_POINT('Ctrl Pts',(-0.385261411552517,-0.691028089876542,
-5.53932232020896));
#47763=CARTESIAN_POINT('Ctrl Pts',(-0.270550102140948,-0.754981844342002,
-5.53403648335032));
#47764=CARTESIAN_POINT('Ctrl Pts',(-0.139570751141121,-0.789756259424867,
-5.52875064649167));
#47765=CARTESIAN_POINT('Ctrl Pts',(-0.00824331789442176,-0.791124658030534,
-5.52346480963302));
#47766=CARTESIAN_POINT('Ctrl Pts',(0.123084115352277,-0.7924930566362,-5.51817897277437));
#47767=CARTESIAN_POINT('Ctrl Pts',(0.254759630845846,-0.760455438764667,
-5.51289313591572));
#47768=CARTESIAN_POINT('Ctrl Pts',(0.370778653329351,-0.698905835406252,
-5.50760729905707));
#47769=CARTESIAN_POINT('Ctrl Pts',(0.486797675812856,-0.637356232047837,
-5.50232146219843));
#47770=CARTESIAN_POINT('Ctrl Pts',(0.587160205286296,-0.546294643202539,
-5.49703562533978));
#47771=CARTESIAN_POINT('Ctrl Pts',(0.659667621238271,-0.436789201028132,
-5.49174978848114));
#47772=CARTESIAN_POINT('Ctrl Pts',(0.732175037190245,-0.327283758853726,
-5.48646395162249));
#47773=CARTESIAN_POINT('Ctrl Pts',(0.776827339620753,-0.199334463350209,
-5.48117811476383));
#47774=CARTESIAN_POINT('Ctrl Pts',(0.788197239095969,-0.0684929843301605,
-5.47589227790519));
#47775=CARTESIAN_POINT('Ctrl Pts',(0.799567138571185,0.0623484946898892,
-5.47060644104654));
#47776=CARTESIAN_POINT('Ctrl Pts',(0.777654635091107,0.196082157226472,
-5.46532060418789));
#47777=CARTESIAN_POINT('Ctrl Pts',(0.725123096324371,0.316453269519017,
-5.46003476732925));
#47778=CARTESIAN_POINT('Ctrl Pts',(0.672591557557635,0.436824381811562,
-5.4547489304706));
#47779=CARTESIAN_POINT('Ctrl Pts',(0.589440983504239,0.543832943860071,
-5.44946309361195));
#47780=CARTESIAN_POINT('Ctrl Pts',(0.485777957826538,0.624472539281158,
-5.4441772567533));
#47781=CARTESIAN_POINT('Ctrl Pts',(0.382114932148837,0.705112134702245,
-5.43889141989465));
#47782=CARTESIAN_POINT('Ctrl Pts',(0.257939454846829,0.759382763495911,
-5.43360558303601));
#47783=CARTESIAN_POINT('Ctrl Pts',(0.128344504715389,0.780688071335382,
-5.42831974617736));
#47784=CARTESIAN_POINT('Ctrl Pts',(-0.00125044541605168,0.801993379174853,
-5.42303390931871));
#47785=CARTESIAN_POINT('Ctrl Pts',(-0.136264868376925,0.79033336606013,
-5.41774807246006));
#47786=CARTESIAN_POINT('Ctrl Pts',(-0.26028835958063,0.747125254886002,
-5.41246223560142));
#47787=CARTESIAN_POINT('Ctrl Pts',(-0.384311850784336,0.703917143711875,
-5.40717639874277));
#47788=CARTESIAN_POINT('Ctrl Pts',(-0.497344410230873,0.629160934478343,
-5.40189056188412));
#47789=CARTESIAN_POINT('Ctrl Pts',(-0.58564743139563,0.531942913026377,
-5.39660472502547));
#47790=CARTESIAN_POINT('Ctrl Pts',(-0.673950452560386,0.434724891574412,
-5.39131888816682));
#47791=CARTESIAN_POINT('Ctrl Pts',(-0.737523935443362,0.315045057904013,
-5.38603305130817));
#47792=CARTESIAN_POINT('Ctrl Pts',(-0.76864080502364,0.187449965250839,
-5.38074721444953));
#47793=CARTESIAN_POINT('Ctrl Pts',(-0.783581726783468,0.126184538426627,
-5.37820919324092));
#47794=CARTESIAN_POINT('Ctrl Pts',(-0.79103981326595,0.0630942576475916,
-5.37567117203231));
#47795=CARTESIAN_POINT('Ctrl Pts',(-0.791033090718594,2.41426438800759E-6,
-5.3731331508237));
#47796=CARTESIAN_POINT('Origin',(0.,0.,-2.94));
#47797=CARTESIAN_POINT('',(-0.791162299475494,7.14138476723761E-6,-5.1446668491763));
#47798=CARTESIAN_POINT('',(-0.791152598342819,1.19001633874275E-5,-5.1731331508237));
#47799=CARTESIAN_POINT('',(-0.7911,-9.68818082805471E-17,-2.94));
#47800=CARTESIAN_POINT('Ctrl Pts',(-0.791162299475494,7.14138476723761E-6,
-5.1446668491763));
#47801=CARTESIAN_POINT('Ctrl Pts',(-0.791165583502069,0.00693560089265366,
-5.14494569421816));
#47802=CARTESIAN_POINT('Ctrl Pts',(-0.791076463159219,0.0138639757192367,
-5.14522453926003));
#47803=CARTESIAN_POINT('Ctrl Pts',(-0.79089440411256,0.0207899075053255,
-5.1455033843019));
#47804=CARTESIAN_POINT('Ctrl Pts',(-0.787443260018906,0.152079118424528,
-5.15078922116055));
#47805=CARTESIAN_POINT('Ctrl Pts',(-0.750595822533239,0.282490455069959,
-5.15607505801919));
#47806=CARTESIAN_POINT('Ctrl Pts',(-0.684830734336137,0.396172997589774,
-5.16136089487784));
#47807=CARTESIAN_POINT('Ctrl Pts',(-0.619065646139034,0.509855540109591,
-5.16664673173649));
#47808=CARTESIAN_POINT('Ctrl Pts',(-0.524382907230495,0.606809288503791,
-5.17193256859513));
#47809=CARTESIAN_POINT('Ctrl Pts',(-0.412290784793401,0.675249944453965,
-5.17721840545378));
#47810=CARTESIAN_POINT('Ctrl Pts',(-0.300198662356306,0.743690600404138,
-5.18250424231243));
#47811=CARTESIAN_POINT('Ctrl Pts',(-0.170697156390656,0.783618163910285,
-5.18779007917108));
#47812=CARTESIAN_POINT('Ctrl Pts',(-0.0395266008624761,0.790179616628333,
-5.19307591602973));
#47813=CARTESIAN_POINT('Ctrl Pts',(0.0916439546657044,0.79674106934638,
-5.19836175288837));
#47814=CARTESIAN_POINT('Ctrl Pts',(0.224483559756416,0.769936411276328,
-5.20364758974702));
#47815=CARTESIAN_POINT('Ctrl Pts',(0.342846149292877,0.71302362978073,-5.20893342660567));
#47816=CARTESIAN_POINT('Ctrl Pts',(0.461208738829339,0.656110848285131,
-5.21421926346432));
#47817=CARTESIAN_POINT('Ctrl Pts',(0.56509431281155,0.569089943363986,-5.21950510032297));
#47818=CARTESIAN_POINT('Ctrl Pts',(0.641876040249872,0.462537920244151,
-5.22479093718161));
#47819=CARTESIAN_POINT('Ctrl Pts',(0.718657767688194,0.355985897124317,
-5.23007677404026));
#47820=CARTESIAN_POINT('Ctrl Pts',(0.768335648582626,0.229902755805793,
-5.23536261089891));
#47821=CARTESIAN_POINT('Ctrl Pts',(0.784871556734003,0.0996133431854589,
-5.24064844775755));
#47822=CARTESIAN_POINT('Ctrl Pts',(0.801407464885379,-0.0306760694348751,
-5.2459342846162));
#47823=CARTESIAN_POINT('Ctrl Pts',(0.784801400293699,-0.165171753357019,
-5.25122012147486));
#47824=CARTESIAN_POINT('Ctrl Pts',(0.737071756494895,-0.28752635442368,
-5.2565059583335));
#47825=CARTESIAN_POINT('Ctrl Pts',(0.68934211269609,-0.409880955490341,
-5.26179179519215));
#47826=CARTESIAN_POINT('Ctrl Pts',(0.610488889690159,-0.520094473701518,
-5.26707763205079));
#47827=CARTESIAN_POINT('Ctrl Pts',(0.510096347174747,-0.60477094449851,
-5.27236346890944));
#47828=CARTESIAN_POINT('Ctrl Pts',(0.409703804659335,-0.689447415295502,
-5.27764930576809));
#47829=CARTESIAN_POINT('Ctrl Pts',(0.287771942634442,-0.748586838678309,
-5.28293514262674));
#47830=CARTESIAN_POINT('Ctrl Pts',(0.159121038401552,-0.775001079901604,
-5.28822097948539));
#47831=CARTESIAN_POINT('Ctrl Pts',(0.0304701341686633,-0.8014153211249,
-5.29350681634404));
#47832=CARTESIAN_POINT('Ctrl Pts',(-0.104899812272221,-0.795104380188685,
-5.29879265320268));
#47833=CARTESIAN_POINT('Ctrl Pts',(-0.230535184030287,-0.756835323987168,
-5.30407849006133));
#47834=CARTESIAN_POINT('Ctrl Pts',(-0.356170555788353,-0.71856626778565,
-5.30936432691998));
#47835=CARTESIAN_POINT('Ctrl Pts',(-0.4720713528636,-0.64833909631883,-5.31465016377863));
#47836=CARTESIAN_POINT('Ctrl Pts',(-0.564150347163279,-0.554689610959313,
-5.31993600063728));
#47837=CARTESIAN_POINT('Ctrl Pts',(-0.656229341462958,-0.461040125599795,
-5.32522183749592));
#47838=CARTESIAN_POINT('Ctrl Pts',(-0.72448653298707,-0.343968326347581,
-5.33050767435457));
#47839=CARTESIAN_POINT('Ctrl Pts',(-0.760625562692054,-0.217703771418954,
-5.33579351121322));
#47840=CARTESIAN_POINT('Ctrl Pts',(-0.780847767349863,-0.14705030640792,
-5.33875129053424));
#47841=CARTESIAN_POINT('Ctrl Pts',(-0.791013290219938,-0.0735184506872712,
-5.34170906985527));
#47842=CARTESIAN_POINT('Ctrl Pts',(-0.791036503466522,7.11594896907197E-6,
-5.3446668491763));
#47843=CARTESIAN_POINT('Ctrl Pts',(-0.791033090718594,2.41426438800759E-6,
-5.3731331508237));
#47844=CARTESIAN_POINT('Ctrl Pts',(-0.791025812481214,-0.0683046408737211,
-5.37038533517366));
#47845=CARTESIAN_POINT('Ctrl Pts',(-0.782268628123843,-0.13661352762463,
-5.36763751952363));
#47846=CARTESIAN_POINT('Ctrl Pts',(-0.764784413766543,-0.202610407135802,
-5.36488970387359));
#47847=CARTESIAN_POINT('Ctrl Pts',(-0.73115089665159,-0.329565335233317,
-5.35960386701494));
#47848=CARTESIAN_POINT('Ctrl Pts',(-0.665223606144103,-0.447964839792398,
-5.35431803015629));
#47849=CARTESIAN_POINT('Ctrl Pts',(-0.57501571214768,-0.543417985903174,
-5.34903219329764));
#47850=CARTESIAN_POINT('Ctrl Pts',(-0.484807818151257,-0.638871132013949,
-5.34374635643899));
#47851=CARTESIAN_POINT('Ctrl Pts',(-0.370319320665898,-0.71137791967642,
-5.33846051958035));
#47852=CARTESIAN_POINT('Ctrl Pts',(-0.245465789029923,-0.752125470274645,
-5.3331746827217));
#47853=CARTESIAN_POINT('Ctrl Pts',(-0.120612257393947,-0.792873020872871,
-5.32788884586305));
#47854=CARTESIAN_POINT('Ctrl Pts',(0.0146063083926455,-0.801861334406852,
-5.3226030090044));
#47855=CARTESIAN_POINT('Ctrl Pts',(0.143754691086471,-0.777997921212178,
-5.31731717214575));
#47856=CARTESIAN_POINT('Ctrl Pts',(0.272903073780296,-0.754134508017505,
-5.3120313352871));
#47857=CARTESIAN_POINT('Ctrl Pts',(0.395981273381354,-0.697419368094177,
-5.30674549842846));
#47858=CARTESIAN_POINT('Ctrl Pts',(0.498029680337536,-0.614745975279851,
-5.30145966156981));
#47859=CARTESIAN_POINT('Ctrl Pts',(0.600078087293719,-0.532072582465523,
-5.29617382471116));
#47860=CARTESIAN_POINT('Ctrl Pts',(0.681096701605026,-0.423440936760197,
-5.29088798785252));
#47861=CARTESIAN_POINT('Ctrl Pts',(0.731238069859886,-0.302054733132022,
-5.28560215099387));
#47862=CARTESIAN_POINT('Ctrl Pts',(0.781379438114745,-0.180668529503849,
-5.28031631413522));
#47863=CARTESIAN_POINT('Ctrl Pts',(0.800643560313157,-0.0465277679528264,
-5.27503047727657));
#47864=CARTESIAN_POINT('Ctrl Pts',(0.786688967800344,0.0840633366046011,
-5.26974464041792));
#47865=CARTESIAN_POINT('Ctrl Pts',(0.772734375287532,0.21465444116203,-5.26445880355928));
#47866=CARTESIAN_POINT('Ctrl Pts',(0.725561068063496,0.341695888725864,
-5.25917296670063));
#47867=CARTESIAN_POINT('Ctrl Pts',(0.650902752500616,0.449746354523297,
-5.25388712984198));
#47868=CARTESIAN_POINT('Ctrl Pts',(0.576244436937734,0.55779682032073,-5.24860129298333));
#47869=CARTESIAN_POINT('Ctrl Pts',(0.474101113036009,0.64685630435176,-5.24331545612469));
#47870=CARTESIAN_POINT('Ctrl Pts',(0.356887849011243,0.706100021135814,
-5.23802961926604));
#47871=CARTESIAN_POINT('Ctrl Pts',(0.239674584986477,0.765343737919869,
-5.23274378240739));
#47872=CARTESIAN_POINT('Ctrl Pts',(0.107391380838672,0.794771687456947,
-5.22745794554874));
#47873=CARTESIAN_POINT('Ctrl Pts',(-0.0238833263834611,0.790807032935806,
-5.22217210869009));
#47874=CARTESIAN_POINT('Ctrl Pts',(-0.155158033605592,0.786842378414665,
-5.21688627183145));
#47875=CARTESIAN_POINT('Ctrl Pts',(-0.285424243902055,0.749485119835303,
-5.2116004349728));
#47876=CARTESIAN_POINT('Ctrl Pts',(-0.398848676885365,0.683275866372188,
-5.20631459811415));
#47877=CARTESIAN_POINT('Ctrl Pts',(-0.512273109868676,0.617066612909072,
-5.2010287612555));
#47878=CARTESIAN_POINT('Ctrl Pts',(-0.608855765538835,0.522005364562204,
-5.19574292439686));
#47879=CARTESIAN_POINT('Ctrl Pts',(-0.676857450252979,0.409646394658744,
-5.19045708753821));
#47880=CARTESIAN_POINT('Ctrl Pts',(-0.744859134967124,0.297287424755283,
-5.18517125067956));
#47881=CARTESIAN_POINT('Ctrl Pts',(-0.78427984872525,0.167630733295234,
-5.17988541382091));
#47882=CARTESIAN_POINT('Ctrl Pts',(-0.790328178523278,0.0364355163535207,
-5.17459957696226));
#47883=CARTESIAN_POINT('Ctrl Pts',(-0.790887498907648,0.0243032151038108,
-5.17411076824941));
#47884=CARTESIAN_POINT('Ctrl Pts',(-0.791161430049627,0.0121577569090612,
-5.17362195953655));
#47885=CARTESIAN_POINT('Ctrl Pts',(-0.791152598342819,1.19001633874275E-5,
-5.1731331508237));
#47886=CARTESIAN_POINT('Origin',(0.,0.,-2.94));
#47887=CARTESIAN_POINT('',(-0.791060709844548,-1.70870917380883E-5,-4.9446668491763));
#47888=CARTESIAN_POINT('',(-0.791074454148617,-1.92722236624013E-5,-4.9731331508237));
#47889=CARTESIAN_POINT('',(-0.7911,-9.68818082805471E-17,-2.94));
#47890=CARTESIAN_POINT('Ctrl Pts',(-0.791060709844548,-1.70870917380883E-5,
-4.9446668491763));
#47891=CARTESIAN_POINT('Ctrl Pts',(-0.790991723705553,0.087364085980534,
-4.94818231858106));
#47892=CARTESIAN_POINT('Ctrl Pts',(-0.776551363288388,0.174767498638758,
-4.95169778798581));
#47893=CARTESIAN_POINT('Ctrl Pts',(-0.748137656794717,0.25736399358953,
-4.95521325739057));
#47894=CARTESIAN_POINT('Ctrl Pts',(-0.705414993109545,0.381555544457479,
-4.96049909424922));
#47895=CARTESIAN_POINT('Ctrl Pts',(-0.631101481703098,0.494879647795438,
-4.96578493110787));
#47896=CARTESIAN_POINT('Ctrl Pts',(-0.534229600452781,0.583562261211863,
-4.97107076796652));
#47897=CARTESIAN_POINT('Ctrl Pts',(-0.437357719202465,0.672244874628287,
-4.97635660482517));
#47898=CARTESIAN_POINT('Ctrl Pts',(-0.317927468108279,0.736285998123177,
-4.98164244168382));
#47899=CARTESIAN_POINT('Ctrl Pts',(-0.190455064752799,0.767901717031971,
-4.98692827854246));
#47900=CARTESIAN_POINT('Ctrl Pts',(-0.0629826613973188,0.799517435940764,
-4.99221411540111));
#47901=CARTESIAN_POINT('Ctrl Pts',(0.0725318942194566,0.798707750263462,
-4.99749995225976));
#47902=CARTESIAN_POINT('Ctrl Pts',(0.199617408602439,0.765571073704779,
-5.0027857891184));
#47903=CARTESIAN_POINT('Ctrl Pts',(0.326702922985424,0.732434397146095,
-5.00807162597705));
#47904=CARTESIAN_POINT('Ctrl Pts',(0.445359396134616,0.666970729706029,
-5.0133574628357));
#47905=CARTESIAN_POINT('Ctrl Pts',(0.541164659746473,0.5771368899595,-5.01864329969435));
#47906=CARTESIAN_POINT('Ctrl Pts',(0.636969923358331,0.487303050212971,
-5.023929136553));
#47907=CARTESIAN_POINT('Ctrl Pts',(0.709923977432854,0.373099038159977,
-5.02921497341164));
#47908=CARTESIAN_POINT('Ctrl Pts',(0.751159580104816,0.248405845195715,
-5.03450081027029));
#47909=CARTESIAN_POINT('Ctrl Pts',(0.792395182776778,0.123712652231453,
-5.03978664712894));
#47910=CARTESIAN_POINT('Ctrl Pts',(0.801912334046179,-0.0114697216440781,
-5.04507248398759));
#47911=CARTESIAN_POINT('Ctrl Pts',(0.778554266366044,-0.140710458153868,
-5.05035832084624));
#47912=CARTESIAN_POINT('Ctrl Pts',(0.755196198685909,-0.269951194663658,
-5.05564415770488));
#47913=CARTESIAN_POINT('Ctrl Pts',(0.698962912056239,-0.393250293807705,
-5.06092999456353));
#47914=CARTESIAN_POINT('Ctrl Pts',(0.616689313183004,-0.495621296673696,
-5.06621583142218));
#47915=CARTESIAN_POINT('Ctrl Pts',(0.534415714309769,-0.597992299539687,
-5.07150166828082));
#47916=CARTESIAN_POINT('Ctrl Pts',(0.42610180319297,-0.679435206127621,
-5.07678750513948));
#47917=CARTESIAN_POINT('Ctrl Pts',(0.304912655570005,-0.730050992180607,
-5.08207334199812));
#47918=CARTESIAN_POINT('Ctrl Pts',(0.183723507947039,-0.780666778233593,
-5.08735917885677));
#47919=CARTESIAN_POINT('Ctrl Pts',(0.0496591238179061,-0.800455443751631,
-5.09264501571542));
#47920=CARTESIAN_POINT('Ctrl Pts',(-0.0809855652379758,-0.787011764164759,
-5.09793085257406));
#47921=CARTESIAN_POINT('Ctrl Pts',(-0.211630254293858,-0.773568084577886,
-5.10321668943271));
#47922=CARTESIAN_POINT('Ctrl Pts',(-0.33885524827649,-0.726892059886103,
-5.10850252629136));
#47923=CARTESIAN_POINT('Ctrl Pts',(-0.447196913159535,-0.652656953974463,
-5.11378836315001));
#47924=CARTESIAN_POINT('Ctrl Pts',(-0.555538578042581,-0.578421848062822,
-5.11907420000866));
#47925=CARTESIAN_POINT('Ctrl Pts',(-0.644996913826041,-0.476627660931325,
-5.12436003686731));
#47926=CARTESIAN_POINT('Ctrl Pts',(-0.704698656366949,-0.359647024769088,
-5.12964587372595));
#47927=CARTESIAN_POINT('Ctrl Pts',(-0.761250938312779,-0.248837496656634,
-5.13465286554273));
#47928=CARTESIAN_POINT('Ctrl Pts',(-0.791103330902562,-0.124401525976414,
-5.13965985735951));
#47929=CARTESIAN_POINT('Ctrl Pts',(-0.791162299475494,7.14138476723761E-6,
-5.1446668491763));
#47930=CARTESIAN_POINT('Ctrl Pts',(-0.791152598342819,1.19001633874275E-5,
-5.1731331508237));
#47931=CARTESIAN_POINT('Ctrl Pts',(-0.791065926511851,-0.119184045267977,
-5.16833612267791));
#47932=CARTESIAN_POINT('Ctrl Pts',(-0.763746661094271,-0.238418374721096,
-5.16353909453211));
#47933=CARTESIAN_POINT('Ctrl Pts',(-0.711677133692105,-0.345632512937747,
-5.15874206638632));
#47934=CARTESIAN_POINT('Ctrl Pts',(-0.654301813224974,-0.463771582863925,
-5.15345622952767));
#47935=CARTESIAN_POINT('Ctrl Pts',(-0.566875226452784,-0.567315980292908,
-5.14817039266903));
#47936=CARTESIAN_POINT('Ctrl Pts',(-0.460023687432986,-0.643680342732655,
-5.14288455581038));
#47937=CARTESIAN_POINT('Ctrl Pts',(-0.353172148413187,-0.720044705172403,
-5.13759871895173));
#47938=CARTESIAN_POINT('Ctrl Pts',(-0.226895657145782,-0.769229032622914,
-5.13231288209308));
#47939=CARTESIAN_POINT('Ctrl Pts',(-0.0965425613568067,-0.785255188118193,
-5.12702704523443));
#47940=CARTESIAN_POINT('Ctrl Pts',(0.0338105344321687,-0.801281343613472,
-5.12174120837578));
#47941=CARTESIAN_POINT('Ctrl Pts',(0.168240234742713,-0.784149327153519,
-5.11645537151714));
#47942=CARTESIAN_POINT('Ctrl Pts',(0.290407205433014,-0.735941459392293,
-5.11116953465849));
#47943=CARTESIAN_POINT('Ctrl Pts',(0.412574176123315,-0.687733591631067,
-5.10588369779984));
#47944=CARTESIAN_POINT('Ctrl Pts',(0.522478417193373,-0.608449872568568,
-5.10059786094119));
#47945=CARTESIAN_POINT('Ctrl Pts',(0.606761555349955,-0.507726886789714,
-5.09531202408255));
#47946=CARTESIAN_POINT('Ctrl Pts',(0.691044693506536,-0.407003901010859,
-5.0900261872239));
#47947=CARTESIAN_POINT('Ctrl Pts',(0.74970672874964,-0.284841648515652,
-5.08474035036525));
#47948=CARTESIAN_POINT('Ctrl Pts',(0.775617550746048,-0.156088409545911,
-5.0794545135066));
#47949=CARTESIAN_POINT('Ctrl Pts',(0.801528372742457,-0.0273351705761713,
-5.07416867664796));
#47950=CARTESIAN_POINT('Ctrl Pts',(0.79468798149217,0.1080090548681,-5.06888283978931));
#47951=CARTESIAN_POINT('Ctrl Pts',(0.755927796227998,0.233493776169203,
-5.06359700293066));
#47952=CARTESIAN_POINT('Ctrl Pts',(0.717167610963826,0.358978497470306,
-5.05831116607201));
#47953=CARTESIAN_POINT('Ctrl Pts',(0.646487631685767,0.474603714628243,
-5.05302532921336));
#47954=CARTESIAN_POINT('Ctrl Pts',(0.552478696548582,0.566315695067557,
-5.04773949235472));
#47955=CARTESIAN_POINT('Ctrl Pts',(0.458469761411397,0.658027675506871,
-5.04245365549607));
#47956=CARTESIAN_POINT('Ctrl Pts',(0.341131870415083,0.725826419227564,
-5.03716781863742));
#47957=CARTESIAN_POINT('Ctrl Pts',(0.214726924047817,0.761471289484268,
-5.03188198177878));
#47958=CARTESIAN_POINT('Ctrl Pts',(0.0883219776805511,0.797116159740973,
-5.02659614492013));
#47959=CARTESIAN_POINT('Ctrl Pts',(-0.0471500240576684,0.80060715653369,
-5.02131030806148));
#47960=CARTESIAN_POINT('Ctrl Pts',(-0.175223059907049,0.77151996467796,
-5.01602447120283));
#47961=CARTESIAN_POINT('Ctrl Pts',(-0.30329609575643,0.74243277282223,-5.01073863434418));
#47962=CARTESIAN_POINT('Ctrl Pts',(-0.423970165716971,0.680767392318055,
-5.00545279748554));
#47963=CARTESIAN_POINT('Ctrl Pts',(-0.52257787153678,0.594018976801212,
-5.00016696062689));
#47964=CARTESIAN_POINT('Ctrl Pts',(-0.621185577356588,0.507270561284372,
-4.99488112376824));
#47965=CARTESIAN_POINT('Ctrl Pts',(-0.697726919035664,0.395439110754866,
-4.98959528690959));
#47966=CARTESIAN_POINT('Ctrl Pts',(-0.742898635803003,0.272117242272348,
-4.98430945005094));
#47967=CARTESIAN_POINT('Ctrl Pts',(-0.774735450338439,0.185200566617459,
-4.9805840169752));
#47968=CARTESIAN_POINT('Ctrl Pts',(-0.790989829011766,0.09257618163275,
-4.97685858389945));
#47969=CARTESIAN_POINT('Ctrl Pts',(-0.791074454148617,-1.92722236624013E-5,
-4.9731331508237));
#47970=CARTESIAN_POINT('Origin',(0.,0.,-2.94));
#47971=CARTESIAN_POINT('',(-0.791081199896583,1.98953686311731E-5,-4.7446668491763));
#47972=CARTESIAN_POINT('',(-0.791066624166131,1.81968424752065E-5,-4.7731331508237));
#47973=CARTESIAN_POINT('',(-0.7911,-9.68818082805471E-17,-2.94));
#47974=CARTESIAN_POINT('Ctrl Pts',(-0.791081199896583,1.98953686311731E-5,
-4.7446668491763));
#47975=CARTESIAN_POINT('Ctrl Pts',(-0.791116059373008,0.0364627458325065,
-4.7461331060853));
#47976=CARTESIAN_POINT('Ctrl Pts',(-0.78864369690631,0.0729009040620994,
-4.7475993629943));
#47977=CARTESIAN_POINT('Ctrl Pts',(-0.783625203153027,0.108984951686083,
-4.74906561990331));
#47978=CARTESIAN_POINT('Ctrl Pts',(-0.765533599223943,0.239067468446083,
-4.75435145676196));
#47979=CARTESIAN_POINT('Ctrl Pts',(-0.714352651056501,0.364547988526248,
-4.75963729362061));
#47980=CARTESIAN_POINT('Ctrl Pts',(-0.636303176013754,0.470174910969791,
-4.76492313047925));
#47981=CARTESIAN_POINT('Ctrl Pts',(-0.558253700971008,0.575801833413333,
-4.7702089673379));
#47982=CARTESIAN_POINT('Ctrl Pts',(-0.453335699052961,0.661575158220248,
-4.77549480419655));
#47983=CARTESIAN_POINT('Ctrl Pts',(-0.334301488288068,0.717069517996006,
-4.7807806410552));
#47984=CARTESIAN_POINT('Ctrl Pts',(-0.215267277523172,0.772563877771764,
-4.78606647791385));
#47985=CARTESIAN_POINT('Ctrl Pts',(-0.0821168579114289,0.797779272516364,
-4.79135231477249));
#47986=CARTESIAN_POINT('Ctrl Pts',(0.0489659273031979,0.789650882779206,
-4.79663815163114));
#47987=CARTESIAN_POINT('Ctrl Pts',(0.180048712517823,0.781522493042048,
-4.80192398848979));
#47988=CARTESIAN_POINT('Ctrl Pts',(0.309063863335332,0.740050318823134,
-4.80720982534844));
#47989=CARTESIAN_POINT('Ctrl Pts',(0.420330160101931,0.670275119051369,
-4.81249566220709));
#47990=CARTESIAN_POINT('Ctrl Pts',(0.53159645686853,0.600499919279603,-4.81778149906573));
#47991=CARTESIAN_POINT('Ctrl Pts',(0.625113899584218,0.502421693954985,
-4.82306733592438));
#47992=CARTESIAN_POINT('Ctrl Pts',(0.689515857652561,0.387961416581977,
-4.82835317278303));
#47993=CARTESIAN_POINT('Ctrl Pts',(0.753917815720905,0.273501139208968,
-4.83363900964167));
#47994=CARTESIAN_POINT('Ctrl Pts',(0.789204289141904,0.14265880978757,-4.83892484650033));
#47995=CARTESIAN_POINT('Ctrl Pts',(0.791086363497242,0.0113377334309409,
-4.84421068335897));
#47996=CARTESIAN_POINT('Ctrl Pts',(0.79296843785258,-0.119983342925686,
-4.84949652021762));
#47997=CARTESIAN_POINT('Ctrl Pts',(0.761446113142258,-0.251783166217544,
-4.85478235707627));
#47998=CARTESIAN_POINT('Ctrl Pts',(0.700350788195395,-0.36804205219612,
-4.86006819393491));
#47999=CARTESIAN_POINT('Ctrl Pts',(0.639255463248531,-0.484300938174695,
-4.86535403079356));
#48000=CARTESIAN_POINT('Ctrl Pts',(0.548587138065126,-0.585018886839986,
-4.87063986765221));
#48001=CARTESIAN_POINT('Ctrl Pts',(0.439366145635789,-0.657954078017449,
-4.87592570451086));
#48002=CARTESIAN_POINT('Ctrl Pts',(0.330145153206451,-0.730889269194912,
-4.88121154136951));
#48003=CARTESIAN_POINT('Ctrl Pts',(0.202371493531181,-0.776041702884544,
-4.88649737822815));
#48004=CARTESIAN_POINT('Ctrl Pts',(0.0715754885190008,-0.787923300933478,
-4.8917832150868));
#48005=CARTESIAN_POINT('Ctrl Pts',(-0.0592205164931791,-0.799804898982411,
-4.89706905194545));
#48006=CARTESIAN_POINT('Ctrl Pts',(-0.193038866842269,-0.778415661390645,
-4.9023548888041));
#48007=CARTESIAN_POINT('Ctrl Pts',(-0.313614535264138,-0.726355355168322,
-4.90764072566275));
#48008=CARTESIAN_POINT('Ctrl Pts',(-0.434190203686007,-0.674295048945999,
-4.91292656252139));
#48009=CARTESIAN_POINT('Ctrl Pts',(-0.541523190180656,-0.591563674093118,
-4.91821239938004));
#48010=CARTESIAN_POINT('Ctrl Pts',(-0.622567646050043,-0.488216862472354,
-4.92349823623868));
#48011=CARTESIAN_POINT('Ctrl Pts',(-0.70361210191943,-0.38487005085159,
-4.92878407309733));
#48012=CARTESIAN_POINT('Ctrl Pts',(-0.758368027163554,-0.260907802462944,
-4.93406990995598));
#48013=CARTESIAN_POINT('Ctrl Pts',(-0.780180081803669,-0.131397179069651,
-4.93935574681463));
#48014=CARTESIAN_POINT('Ctrl Pts',(-0.787485519460927,-0.0880206241891952,
-4.94112611426852));
#48015=CARTESIAN_POINT('Ctrl Pts',(-0.791095450814012,-0.0440216756909996,
-4.94289648172241));
#48016=CARTESIAN_POINT('Ctrl Pts',(-0.791060709844548,-1.70870917380883E-5,
-4.9446668491763));
#48017=CARTESIAN_POINT('Ctrl Pts',(-0.791074454148617,-1.92722236624013E-5,
-4.9731331508237));
#48018=CARTESIAN_POINT('Ctrl Pts',(-0.79110989952664,-0.0388030306590331,
-4.9715727470408));
#48019=CARTESIAN_POINT('Ctrl Pts',(-0.788308576656797,-0.0775817135126429,
-4.9700123432579));
#48020=CARTESIAN_POINT('Ctrl Pts',(-0.782627328289855,-0.115933781244964,
-4.968451939475));
#48021=CARTESIAN_POINT('Ctrl Pts',(-0.763382212153763,-0.245850649844223,
-4.96316610261635));
#48022=CARTESIAN_POINT('Ctrl Pts',(-0.711089888025977,-0.370872100607207,
-4.9578802657577));
#48023=CARTESIAN_POINT('Ctrl Pts',(-0.632106256090772,-0.475802330417557,
-4.95259442889906));
#48024=CARTESIAN_POINT('Ctrl Pts',(-0.553122624155568,-0.580732560227904,
-4.94730859204041));
#48025=CARTESIAN_POINT('Ctrl Pts',(-0.447447684412945,-0.665571569085619,
-4.94202275518176));
#48026=CARTESIAN_POINT('Ctrl Pts',(-0.327925757328409,-0.720007551557941,
-4.93673691832311));
#48027=CARTESIAN_POINT('Ctrl Pts',(-0.208403830243871,-0.774443534030264,
-4.93145108146446));
#48028=CARTESIAN_POINT('Ctrl Pts',(-0.0750349158174182,-0.798476490117193,
-4.92616524460582));
#48029=CARTESIAN_POINT('Ctrl Pts',(0.0559705856308531,-0.789185320545187,
-4.92087940774717));
#48030=CARTESIAN_POINT('Ctrl Pts',(0.186976087079124,-0.779894150973181,
-4.91559357088852));
#48031=CARTESIAN_POINT('Ctrl Pts',(0.315618175549214,-0.737278855742239,
-4.91030773402987));
#48032=CARTESIAN_POINT('Ctrl Pts',(0.426260975461859,-0.666519135072786,
-4.90502189717122));
#48033=CARTESIAN_POINT('Ctrl Pts',(0.536903775374505,-0.595759414403333,
-4.89973606031258));
#48034=CARTESIAN_POINT('Ctrl Pts',(0.629547286729707,-0.496855268295371,
-4.89445022345393));
#48035=CARTESIAN_POINT('Ctrl Pts',(0.692931101413733,-0.381828057263242,
-4.88916438659528));
#48036=CARTESIAN_POINT('Ctrl Pts',(0.75631491609776,-0.266800846231114,
-4.88387854973664));
#48037=CARTESIAN_POINT('Ctrl Pts',(0.790439034110611,-0.135650570274821,
-4.87859271287799));
#48038=CARTESIAN_POINT('Ctrl Pts',(0.791155820181074,-0.00431796404370287,
-4.87330687601934));
#48039=CARTESIAN_POINT('Ctrl Pts',(0.791872606251537,0.127014642187415,
-4.86802103916069));
#48040=CARTESIAN_POINT('Ctrl Pts',(0.759182060379613,0.258529578693358,
-4.86273520230204));
#48041=CARTESIAN_POINT('Ctrl Pts',(0.697057573497852,0.374241787951529,
-4.85744936544339));
#48042=CARTESIAN_POINT('Ctrl Pts',(0.634933086616092,0.4899539972097,-4.85216352858475));
#48043=CARTESIAN_POINT('Ctrl Pts',(0.543374658724495,0.589863479220098,
-4.8468776917261));
#48044=CARTESIAN_POINT('Ctrl Pts',(0.433510810852,0.661826679346121,-4.84159185486745));
#48045=CARTESIAN_POINT('Ctrl Pts',(0.323646962979506,0.733789879472143,
-4.83630601800881));
#48046=CARTESIAN_POINT('Ctrl Pts',(0.195477695126116,0.777806797713789,
-4.83102018115015));
#48047=CARTESIAN_POINT('Ctrl Pts',(0.0645814136211574,0.788527372787123,
-4.82573434429151));
#48048=CARTESIAN_POINT('Ctrl Pts',(-0.0663148678837991,0.799247947860457,
-4.82044850743286));
#48049=CARTESIAN_POINT('Ctrl Pts',(-0.199938163040322,0.776672179765479,
-4.81516267057421));
#48050=CARTESIAN_POINT('Ctrl Pts',(-0.320047152678255,0.723544053035068,
-4.80987683371557));
#48051=CARTESIAN_POINT('Ctrl Pts',(-0.440156142316193,0.670415926304655,
-4.80459099685692));
#48052=CARTESIAN_POINT('Ctrl Pts',(-0.54675082643554,0.586735440938804,
-4.79930515999826));
#48053=CARTESIAN_POINT('Ctrl Pts',(-0.626875093719053,0.482673588975613,
-4.79401932313962));
#48054=CARTESIAN_POINT('Ctrl Pts',(-0.706999361002566,0.378611737012422,
-4.78873348628097));
#48055=CARTESIAN_POINT('Ctrl Pts',(-0.760653211450246,0.254168518451889,
-4.78344764942233));
#48056=CARTESIAN_POINT('Ctrl Pts',(-0.781315257389323,0.124469454849486,
-4.77816181256368));
#48057=CARTESIAN_POINT('Ctrl Pts',(-0.787867511564775,0.0833398768034945,
-4.77648559198369));
#48058=CARTESIAN_POINT('Ctrl Pts',(-0.791102036830354,0.0416817593429142,
-4.7748093714037));
#48059=CARTESIAN_POINT('Ctrl Pts',(-0.791066624166131,1.81968424752065E-5,
-4.7731331508237));
#48060=CARTESIAN_POINT('Origin',(0.,0.,-2.94));
#48061=CARTESIAN_POINT('',(-0.791147068928682,-1.37605406554386E-5,-4.54466684917629));
#48062=CARTESIAN_POINT('',(-0.791158453049048,-9.36744769638833E-6,-4.5731331508237));
#48063=CARTESIAN_POINT('',(-0.7911,-9.68818082805471E-17,-2.94));
#48064=CARTESIAN_POINT('Ctrl Pts',(-0.791147068928682,-1.37605406554386E-5,
-4.54466684917629));
#48065=CARTESIAN_POINT('Ctrl Pts',(-0.791051964156756,0.116845203154218,
-4.54936973044819));
#48066=CARTESIAN_POINT('Ctrl Pts',(-0.764828877004105,0.233745430424912,
-4.55407261172009));
#48067=CARTESIAN_POINT('Ctrl Pts',(-0.71471592230546,0.339304183755074,
-4.55877549299199));
#48068=CARTESIAN_POINT('Ctrl Pts',(-0.658391110402443,0.457947695433684,
-4.56406132985064));
#48069=CARTESIAN_POINT('Ctrl Pts',(-0.571886716359079,0.562263754533416,
-4.56934716670928));
#48070=CARTESIAN_POINT('Ctrl Pts',(-0.465716965794738,0.639573206506951,
-4.57463300356793));
#48071=CARTESIAN_POINT('Ctrl Pts',(-0.359547215230401,0.716882658480484,
-4.57991884042658));
#48072=CARTESIAN_POINT('Ctrl Pts',(-0.233712108145087,0.767185503327821,
-4.58520467728523));
#48073=CARTESIAN_POINT('Ctrl Pts',(-0.103506343974174,0.784367653251803,
-4.59049051414388));
#48074=CARTESIAN_POINT('Ctrl Pts',(0.0266994201967425,0.801549803175786,
-4.59577635100253));
#48075=CARTESIAN_POINT('Ctrl Pts',(0.161275841453259,0.785611258176413,
-4.60106218786117));
#48076=CARTESIAN_POINT('Ctrl Pts',(0.283865752373001,0.738489277742304,
-4.60634802471982));
#48077=CARTESIAN_POINT('Ctrl Pts',(0.406455663292742,0.691367297308196,
-4.61163386157847));
#48078=CARTESIAN_POINT('Ctrl Pts',(0.517059063875708,0.613061881439353,
-4.61691969843712));
#48079=CARTESIAN_POINT('Ctrl Pts',(0.602232601089266,0.513090706304351,
-4.62220553529576));
#48080=CARTESIAN_POINT('Ctrl Pts',(0.687406138302824,0.413119531169349,
-4.62749137215441));
#48081=CARTESIAN_POINT('Ctrl Pts',(0.747149812146974,0.291482596768187,
-4.63277720901306));
#48082=CARTESIAN_POINT('Ctrl Pts',(0.774202043911476,0.162964333257111,
-4.63806304587171));
#48083=CARTESIAN_POINT('Ctrl Pts',(0.801254275675977,0.0344460697460355,
-4.64334888273035));
#48084=CARTESIAN_POINT('Ctrl Pts',(0.795615065360831,-0.100953522874955,
-4.648634719589));
#48085=CARTESIAN_POINT('Ctrl Pts',(0.757969833981053,-0.226777224353276,
-4.65392055644765));
#48086=CARTESIAN_POINT('Ctrl Pts',(0.720324602601275,-0.352600925831596,
-4.6592063933063));
#48087=CARTESIAN_POINT('Ctrl Pts',(0.650673350156865,-0.468848736167248,
-4.66449223016494));
#48088=CARTESIAN_POINT('Ctrl Pts',(0.557481877616328,-0.561391249343998,
-4.66977806702359));
#48089=CARTESIAN_POINT('Ctrl Pts',(0.46429040507579,-0.653933762520748,
-4.67506390388224));
#48090=CARTESIAN_POINT('Ctrl Pts',(0.347558712439126,-0.722770978538597,
-4.68034974074089));
#48091=CARTESIAN_POINT('Ctrl Pts',(0.221475019471191,-0.759536038948039,
-4.68563557759954));
#48092=CARTESIAN_POINT('Ctrl Pts',(0.0953913265032548,-0.796301099357482,
-4.69092141445819));
#48093=CARTESIAN_POINT('Ctrl Pts',(-0.0400443667959528,-0.800994004158517,
-4.69620725131683));
#48094=CARTESIAN_POINT('Ctrl Pts',(-0.168370452296446,-0.773044351576371,
-4.70149308817548));
#48095=CARTESIAN_POINT('Ctrl Pts',(-0.296696537796939,-0.745094698994224,
-4.70677892503413));
#48096=CARTESIAN_POINT('Ctrl Pts',(-0.417913015498719,-0.684502489028894,
-4.71206476189278));
#48097=CARTESIAN_POINT('Ctrl Pts',(-0.517286559893452,-0.598632436194564,
-4.71735059875143));
#48098=CARTESIAN_POINT('Ctrl Pts',(-0.616660104288183,-0.512762383360237,
-4.72263643561007));
#48099=CARTESIAN_POINT('Ctrl Pts',(-0.694190715375869,-0.401614487656911,
-4.72792227246872));
#48100=CARTESIAN_POINT('Ctrl Pts',(-0.74045489107435,-0.278698283085334,
-4.73320810932737));
#48101=CARTESIAN_POINT('Ctrl Pts',(-0.773885684080305,-0.189878237551815,
-4.73702768927701));
#48102=CARTESIAN_POINT('Ctrl Pts',(-0.790990391419302,-0.0949132504428775,
-4.74084726922665));
#48103=CARTESIAN_POINT('Ctrl Pts',(-0.791081199896583,1.98953686311731E-5,
-4.7446668491763));
#48104=CARTESIAN_POINT('Ctrl Pts',(-0.791066624166131,1.81968424752065E-5,
-4.7731331508237));
#48105=CARTESIAN_POINT('Ctrl Pts',(-0.790990365629054,-0.0897011844987339,
-4.76952353454505));
#48106=CARTESIAN_POINT('Ctrl Pts',(-0.775750614440565,-0.179445815806044,
-4.76591391826639));
#48107=CARTESIAN_POINT('Ctrl Pts',(-0.745824609176676,-0.263992100196821,
-4.76230430198773));
#48108=CARTESIAN_POINT('Ctrl Pts',(-0.70200167359448,-0.387799682996452,
-4.75701846512908));
#48109=CARTESIAN_POINT('Ctrl Pts',(-0.626685560999614,-0.50045993995144,
-4.75173262827044));
#48110=CARTESIAN_POINT('Ctrl Pts',(-0.529030610999373,-0.588279516255242,
-4.74644679141179));
#48111=CARTESIAN_POINT('Ctrl Pts',(-0.431375660999132,-0.676099092559043,
-4.74116095455315));
#48112=CARTESIAN_POINT('Ctrl Pts',(-0.311381873593517,-0.739077988211657,
-4.7358751176945));
#48113=CARTESIAN_POINT('Ctrl Pts',(-0.183633961705585,-0.769561397633862,
-4.73058928083585));
#48114=CARTESIAN_POINT('Ctrl Pts',(-0.0558860498176521,-0.800044807056067,
-4.7253034439772));
#48115=CARTESIAN_POINT('Ctrl Pts',(0.0796159865525981,-0.798032730247862,
-4.72001760711855));
#48116=CARTESIAN_POINT('Ctrl Pts',(0.206402475568996,-0.763769726225687,
-4.71473177025991));
#48117=CARTESIAN_POINT('Ctrl Pts',(0.333188964585392,-0.729506722203513,
-4.70944593340126));
#48118=CARTESIAN_POINT('Ctrl Pts',(0.451259906247936,-0.66299279096737,
-4.70416009654261));
#48119=CARTESIAN_POINT('Ctrl Pts',(0.546264301009608,-0.572312406000739,
-4.69887425968396));
#48120=CARTESIAN_POINT('Ctrl Pts',(0.641268695771284,-0.481632021034104,
-4.69358842282531));
#48121=CARTESIAN_POINT('Ctrl Pts',(0.713206543632088,-0.36678518233698,
-4.68830258596667));
#48122=CARTESIAN_POINT('Ctrl Pts',(0.753334118087197,-0.241731014033485,
-4.68301674910802));
#48123=CARTESIAN_POINT('Ctrl Pts',(0.793461692542305,-0.116676845729994,
-4.67773091224937));
#48124=CARTESIAN_POINT('Ctrl Pts',(0.801778993591721,0.0185846521798675,
-4.67244507539072));
#48125=CARTESIAN_POINT('Ctrl Pts',(0.777275090163736,0.147613044243476,
-4.66715923853207));
#48126=CARTESIAN_POINT('Ctrl Pts',(0.752771186735752,0.276641436307085,
-4.66187340167343));
#48127=CARTESIAN_POINT('Ctrl Pts',(0.695446078830367,0.39943672252444,-4.65658756481478));
#48128=CARTESIAN_POINT('Ctrl Pts',(0.61226737918954,0.501073680211048,-4.65130172795613));
#48129=CARTESIAN_POINT('Ctrl Pts',(0.529088679548712,0.602710637897657,
-4.64601589109748));
#48130=CARTESIAN_POINT('Ctrl Pts',(0.420056388172441,0.683189267053518,
-4.64073005423883));
#48131=CARTESIAN_POINT('Ctrl Pts',(0.29842289673406,0.732727747068938,-4.63544421738019));
#48132=CARTESIAN_POINT('Ctrl Pts',(0.17678940529568,0.782266227084359,-4.63015838052154));
#48133=CARTESIAN_POINT('Ctrl Pts',(0.0425547137951911,0.80086455795934,
-4.62487254366289));
#48134=CARTESIAN_POINT('Ctrl Pts',(-0.0879655460819782,0.78626219502299,
-4.61958670680424));
#48135=CARTESIAN_POINT('Ctrl Pts',(-0.218485805959148,0.77165983208664,
-4.6143008699456));
#48136=CARTESIAN_POINT('Ctrl Pts',(-0.345291634212997,0.72385677533896,
-4.60901503308695));
#48137=CARTESIAN_POINT('Ctrl Pts',(-0.452970344553351,0.648663274415231,
-4.6037291962283));
#48138=CARTESIAN_POINT('Ctrl Pts',(-0.560649054893706,0.573469773491501,
-4.59844335936965));
#48139=CARTESIAN_POINT('Ctrl Pts',(-0.649200647320564,0.470885828391724,
-4.59315752251101));
#48140=CARTESIAN_POINT('Ctrl Pts',(-0.707862068326336,0.353380062885038,
-4.58787168565236));
#48141=CARTESIAN_POINT('Ctrl Pts',(-0.762384081252103,0.244166021425364,
-4.58295884070947));
#48142=CARTESIAN_POINT('Ctrl Pts',(-0.791085453716163,0.122061757479741,
-4.57804599576659));
#48143=CARTESIAN_POINT('Ctrl Pts',(-0.791158453049048,-9.36744769638833E-6,
-4.5731331508237));
#48144=CARTESIAN_POINT('Origin',(0.,0.,-2.94));
#48145=CARTESIAN_POINT('',(-0.791032667499796,-2.47978686473971E-7,-4.34466684917629));
#48146=CARTESIAN_POINT('',(-0.791034555886587,-5.04054740280758E-6,-4.3731331508237));
#48147=CARTESIAN_POINT('',(-0.7911,-9.68818082805471E-17,-2.94));
#48148=CARTESIAN_POINT('Ctrl Pts',(-0.791032667499796,-2.47978686473971E-7,
-4.34466684917629));
#48149=CARTESIAN_POINT('Ctrl Pts',(-0.791031946004233,0.0659665420417525,
-4.34732051795244));
#48150=CARTESIAN_POINT('Ctrl Pts',(-0.782871044353607,0.131933507406664,
-4.34997418672858));
#48151=CARTESIAN_POINT('Ctrl Pts',(-0.766552074213921,0.195816486101084,
-4.35262785550472));
#48152=CARTESIAN_POINT('Ctrl Pts',(-0.734046354346008,0.323064847486256,
-4.35791369236337));
#48153=CARTESIAN_POINT('Ctrl Pts',(-0.669172219886227,0.442044665325261,
-4.36319952922202));
#48154=CARTESIAN_POINT('Ctrl Pts',(-0.57981483428916,0.538294470200906,
-4.36848536608067));
#48155=CARTESIAN_POINT('Ctrl Pts',(-0.490457448692093,0.634544275076551,
-4.37377120293932));
#48156=CARTESIAN_POINT('Ctrl Pts',(-0.376616811957741,0.708064066988836,
-4.37905703979796));
#48157=CARTESIAN_POINT('Ctrl Pts',(-0.25212974882217,0.749917841146289,
-4.38434287665661));
#48158=CARTESIAN_POINT('Ctrl Pts',(-0.127642685686599,0.791771615303741,
-4.38962871351526));
#48159=CARTESIAN_POINT('Ctrl Pts',(0.00749080385018974,0.801959371706361,
-4.39491455037391));
#48160=CARTESIAN_POINT('Ctrl Pts',(0.136845843185855,0.779242833726043,
-4.40020038723256));
#48161=CARTESIAN_POINT('Ctrl Pts',(0.266200882521519,0.756526295745724,
-4.4054862240912));
#48162=CARTESIAN_POINT('Ctrl Pts',(0.38977747165606,0.700905463382468,-4.41077206094985));
#48163=CARTESIAN_POINT('Ctrl Pts',(0.492555423998938,0.619140802241192,
-4.4160578978085));
#48164=CARTESIAN_POINT('Ctrl Pts',(0.595333376341813,0.537376141099918,
-4.42134373466715));
#48165=CARTESIAN_POINT('Ctrl Pts',(0.677312691893027,0.429467651180626,
-4.42662957152579));
#48166=CARTESIAN_POINT('Ctrl Pts',(0.72852914826412,0.308531131071399,-4.43191540838444));
#48167=CARTESIAN_POINT('Ctrl Pts',(0.779745604635215,0.187594610962168,
-4.43720124524309));
#48168=CARTESIAN_POINT('Ctrl Pts',(0.800199201826187,0.0536300606630008,
-4.44248708210174));
#48169=CARTESIAN_POINT('Ctrl Pts',(0.78740389576989,-0.0770797226061498,
-4.44777291896039));
#48170=CARTESIAN_POINT('Ctrl Pts',(0.774608589713593,-0.2077895058753,-4.45305875581904));
#48171=CARTESIAN_POINT('Ctrl Pts',(0.728564380410028,-0.335244522114434,
-4.45834459267768));
#48172=CARTESIAN_POINT('Ctrl Pts',(0.654867737384667,-0.443953179111636,
-4.46363042953633));
#48173=CARTESIAN_POINT('Ctrl Pts',(0.581171094359306,-0.552661836108837,
-4.46891626639497));
#48174=CARTESIAN_POINT('Ctrl Pts',(0.479822017612149,-0.642624133864105,
-4.47420210325363));
#48175=CARTESIAN_POINT('Ctrl Pts',(0.363139038138284,-0.702905553890879,
-4.47948794011227));
#48176=CARTESIAN_POINT('Ctrl Pts',(0.246456058664419,-0.763186973917653,
-4.48477377697092));
#48177=CARTESIAN_POINT('Ctrl Pts',(0.114439176463847,-0.793787516215932,
-4.49005961382957));
#48178=CARTESIAN_POINT('Ctrl Pts',(-0.0168655416667924,-0.790987820522495,
-4.49534545068821));
#48179=CARTESIAN_POINT('Ctrl Pts',(-0.148170259797432,-0.788188124829056,
-4.50063128754686));
#48180=CARTESIAN_POINT('Ctrl Pts',(-0.27876281385814,-0.751988191143901,
-4.50591712440551));
#48181=CARTESIAN_POINT('Ctrl Pts',(-0.392770257823586,-0.686787960931054,
-4.51120296126416));
#48182=CARTESIAN_POINT('Ctrl Pts',(-0.506777701789033,-0.621587730718207,
-4.51648879812281));
#48183=CARTESIAN_POINT('Ctrl Pts',(-0.604200035659218,-0.527387203977669,
-4.52177463498146));
#48184=CARTESIAN_POINT('Ctrl Pts',(-0.673196006628379,-0.415636037140963,
-4.5270604718401));
#48185=CARTESIAN_POINT('Ctrl Pts',(-0.74219197759754,-0.303884870304259,
-4.53234630869875));
#48186=CARTESIAN_POINT('Ctrl Pts',(-0.782761585665677,-0.174583063371387,
-4.53763214555739));
#48187=CARTESIAN_POINT('Ctrl Pts',(-0.789973774818412,-0.0434466777762086,
-4.54291798241604));
#48188=CARTESIAN_POINT('Ctrl Pts',(-0.790769180744043,-0.0289841261210445,
-4.54350093800279));
#48189=CARTESIAN_POINT('Ctrl Pts',(-0.791158857841673,-0.0144992603458212,
-4.54408389358954));
#48190=CARTESIAN_POINT('Ctrl Pts',(-0.791147068928682,-1.37605406554386E-5,
-4.54466684917629));
#48191=CARTESIAN_POINT('Ctrl Pts',(-0.791158453049048,-9.36744769638833E-6,
-4.5731331508237));
#48192=CARTESIAN_POINT('Ctrl Pts',(-0.791163995288084,-0.00927722411226468,
-4.57276015890794));
#48193=CARTESIAN_POINT('Ctrl Pts',(-0.791004520259269,-0.0185448897596832,
-4.57238716699218));
#48194=CARTESIAN_POINT('Ctrl Pts',(-0.790678799237191,-0.0278067088434459,
-4.57201417507641));
#48195=CARTESIAN_POINT('Ctrl Pts',(-0.786062859557592,-0.159060129151653,
-4.56672833821777));
#48196=CARTESIAN_POINT('Ctrl Pts',(-0.748059730613709,-0.289139383854475,
-4.56144250135912));
#48197=CARTESIAN_POINT('Ctrl Pts',(-0.681288524259648,-0.402233916188058,
-4.55615666450047));
#48198=CARTESIAN_POINT('Ctrl Pts',(-0.614517317905586,-0.515328448521644,
-4.55087082764182));
#48199=CARTESIAN_POINT('Ctrl Pts',(-0.51897803414135,-0.61143825848599,
-4.54558499078317));
#48200=CARTESIAN_POINT('Ctrl Pts',(-0.406283049379935,-0.678881624737636,
-4.54029915392453));
#48201=CARTESIAN_POINT('Ctrl Pts',(-0.293588064618524,-0.74632499098928,
-4.53501331706588));
#48202=CARTESIAN_POINT('Ctrl Pts',(-0.163737378859937,-0.785101913528223,
-4.52972748020723));
#48203=CARTESIAN_POINT('Ctrl Pts',(-0.0325137673261076,-0.790499229319128,
-4.52444164334859));
#48204=CARTESIAN_POINT('Ctrl Pts',(0.0987098442077254,-0.795896545110033,
-4.51915580648994));
#48205=CARTESIAN_POINT('Ctrl Pts',(0.231306381516804,-0.767914254152898,
-4.51386996963129));
#48206=CARTESIAN_POINT('Ctrl Pts',(0.349159323295675,-0.709953479867221,
-4.50858413277264));
#48207=CARTESIAN_POINT('Ctrl Pts',(0.467012265074544,-0.651992705581545,
-4.50329829591399));
#48208=CARTESIAN_POINT('Ctrl Pts',(0.570121611323203,-0.56405344796733,
-4.49801245905534));
#48209=CARTESIAN_POINT('Ctrl Pts',(0.645954878091993,-0.456824333950184,
-4.4927266221967));
#48210=CARTESIAN_POINT('Ctrl Pts',(0.721788144860783,-0.349595219933038,
-4.48744078533805));
#48211=CARTESIAN_POINT('Ctrl Pts',(0.770345332149699,-0.223076249512961,
-4.4821549484794));
#48212=CARTESIAN_POINT('Ctrl Pts',(0.785724529099256,-0.0926452426820873,
-4.47686911162076));
#48213=CARTESIAN_POINT('Ctrl Pts',(0.801103726048813,0.037785764148786,
-4.47158327476211));
#48214=CARTESIAN_POINT('Ctrl Pts',(0.783304932659011,0.172128807390459,
-4.46629743790346));
#48215=CARTESIAN_POINT('Ctrl Pts',(0.73449151336379,0.294055085683687,-4.46101160104481));
#48216=CARTESIAN_POINT('Ctrl Pts',(0.685678094068569,0.415981363976914,
-4.45572576418616));
#48217=CARTESIAN_POINT('Ctrl Pts',(0.605850048867929,0.525490877321699,
-4.45043992732752));
#48218=CARTESIAN_POINT('Ctrl Pts',(0.504710122775864,0.60927322982997,-4.44515409046887));
#48219=CARTESIAN_POINT('Ctrl Pts',(0.403570196683798,0.693055582338243,
-4.43986825361022));
#48220=CARTESIAN_POINT('Ctrl Pts',(0.28111838970031,0.751110774010002,-4.43458241675157));
#48221=CARTESIAN_POINT('Ctrl Pts',(0.152238176131666,0.776382453657973,
-4.42929657989292));
#48222=CARTESIAN_POINT('Ctrl Pts',(0.0233579625630229,0.801654133305943,
-4.42401074303427));
#48223=CARTESIAN_POINT('Ctrl Pts',(-0.111950657590775,0.794142300930125,
-4.41872490617563));
#48224=CARTESIAN_POINT('Ctrl Pts',(-0.237241521377244,0.754759986455616,
-4.41343906931698));
#48225=CARTESIAN_POINT('Ctrl Pts',(-0.362532385163711,0.715377671981108,
-4.40815323245834));
#48226=CARTESIAN_POINT('Ctrl Pts',(-0.477805492582847,0.644124875407914,
-4.40286739559969));
#48227=CARTESIAN_POINT('Ctrl Pts',(-0.569049908437045,0.549662058293695,
-4.39758155874104));
#48228=CARTESIAN_POINT('Ctrl Pts',(-0.660294324291243,0.455199241179475,
-4.39229572188239));
#48229=CARTESIAN_POINT('Ctrl Pts',(-0.727510048580498,0.337526403524228,
-4.38700988502374));
#48230=CARTESIAN_POINT('Ctrl Pts',(-0.762527307986792,0.210946157097699,
-4.38172404816509));
#48231=CARTESIAN_POINT('Ctrl Pts',(-0.78149810919141,0.14237058230678,-4.37886041571796));
#48232=CARTESIAN_POINT('Ctrl Pts',(-0.7910186841546,0.0711806894600302,
-4.37599678327083));
#48233=CARTESIAN_POINT('Ctrl Pts',(-0.791034555886587,-5.04054740280758E-6,
-4.3731331508237));
#48234=CARTESIAN_POINT('Origin',(0.,0.,-2.94));
#48235=CARTESIAN_POINT('',(-0.79114572203675,1.41578566767164E-5,-4.1446668491763));
#48236=CARTESIAN_POINT('',(-0.791131276639148,1.74428956908455E-5,-4.1731331508237));
#48237=CARTESIAN_POINT('',(-0.7911,-9.68818082805471E-17,-2.94));
#48238=CARTESIAN_POINT('Ctrl Pts',(-0.79114572203675,1.41578566767164E-5,
-4.1446668491763));
#48239=CARTESIAN_POINT('Ctrl Pts',(-0.79115820984817,0.015033989046388,
-4.14527130545668));
#48240=CARTESIAN_POINT('Ctrl Pts',(-0.790739241182227,0.030053123953994,
-4.14587576173707));
#48241=CARTESIAN_POINT('Ctrl Pts',(-0.789884112929677,0.0450473845182785,
-4.14648021801746));
#48242=CARTESIAN_POINT('Ctrl Pts',(-0.782406204960389,0.176168886156055,
-4.15176605487611));
#48243=CARTESIAN_POINT('Ctrl Pts',(-0.741574664137056,0.305388217716395,
-4.15705189173475));
#48244=CARTESIAN_POINT('Ctrl Pts',(-0.672352383239296,0.416999342281352,
-4.1623377285934));
#48245=CARTESIAN_POINT('Ctrl Pts',(-0.603130102341536,0.528610466846308,
-4.16762356545205));
#48246=CARTESIAN_POINT('Ctrl Pts',(-0.505517081369349,0.622613384415881,
-4.1729094023107));
#48247=CARTESIAN_POINT('Ctrl Pts',(-0.391377750300425,0.687582457077272,
-4.17819523916935));
#48248=CARTESIAN_POINT('Ctrl Pts',(-0.2772384192315,0.752551529738663,-4.183481076028));
#48249=CARTESIAN_POINT('Ctrl Pts',(-0.146572778065838,0.788486757491872,
-4.18876691288664));
#48250=CARTESIAN_POINT('Ctrl Pts',(-0.0152626562423773,0.791020372705449,
-4.19405274974529));
#48251=CARTESIAN_POINT('Ctrl Pts',(0.116047465581084,0.793553987919027,
-4.19933858660394));
#48252=CARTESIAN_POINT('Ctrl Pts',(0.248002068062344,0.762685990592973,
-4.20462442346258));
#48253=CARTESIAN_POINT('Ctrl Pts',(0.364562654228557,0.702168248963502,
-4.20991026032123));
#48254=CARTESIAN_POINT('Ctrl Pts',(0.48112324039477,0.641650507334031,-4.21519609717988));
#48255=CARTESIAN_POINT('Ctrl Pts',(0.582289810245937,0.551483021401144,
-4.22048193403853));
#48256=CARTESIAN_POINT('Ctrl Pts',(0.655766015691118,0.442625249364784,
-4.22576777089718));
#48257=CARTESIAN_POINT('Ctrl Pts',(0.7292422211363,0.333767477328423,-4.23105360775583));
#48258=CARTESIAN_POINT('Ctrl Pts',(0.775028062175496,0.206219419188591,
-4.23633944461447));
#48259=CARTESIAN_POINT('Ctrl Pts',(0.787558472800413,0.0754839759877756,
-4.24162528147312));
#48260=CARTESIAN_POINT('Ctrl Pts',(0.800088883425329,-0.0552514672130398,
-4.24691111833177));
#48261=CARTESIAN_POINT('Ctrl Pts',(0.779363863635967,-0.189174295474838,
-4.25219695519042));
#48262=CARTESIAN_POINT('Ctrl Pts',(0.727902447713082,-0.310006782706354,
-4.25748279204906));
#48263=CARTESIAN_POINT('Ctrl Pts',(0.676441031790198,-0.430839269937868,
-4.26276862890771));
#48264=CARTESIAN_POINT('Ctrl Pts',(0.594243219733788,-0.538581416139105,
-4.26805446576636));
#48265=CARTESIAN_POINT('Ctrl Pts',(0.491299791213923,-0.620137641063495,
-4.27334030262501));
#48266=CARTESIAN_POINT('Ctrl Pts',(0.388356362694056,-0.701693865987887,
-4.27862613948366));
#48267=CARTESIAN_POINT('Ctrl Pts',(0.264667317710735,-0.757064169635434,
-4.2839119763423));
#48268=CARTESIAN_POINT('Ctrl Pts',(0.135266511364388,-0.779518537056015,
-4.28919781320095));
#48269=CARTESIAN_POINT('Ctrl Pts',(0.00586570501804362,-0.801972904476595,
-4.2944836500596));
#48270=CARTESIAN_POINT('Ctrl Pts',(-0.129246862691322,-0.791511335670206,
-4.29976948691825));
#48271=CARTESIAN_POINT('Ctrl Pts',(-0.253648858116741,-0.749405387948815,
-4.3050553237769));
#48272=CARTESIAN_POINT('Ctrl Pts',(-0.378050853542157,-0.707299440227425,
-4.31034116063554));
#48273=CARTESIAN_POINT('Ctrl Pts',(-0.491742276683628,-0.633549113591034,
-4.31562699749419));
#48274=CARTESIAN_POINT('Ctrl Pts',(-0.580904439055834,-0.537118433304861,
-4.32091283435284));
#48275=CARTESIAN_POINT('Ctrl Pts',(-0.670066601428042,-0.440687753018685,
-4.32619867121149));
#48276=CARTESIAN_POINT('Ctrl Pts',(-0.734699503030983,-0.321576719082726,
-4.33148450807013));
#48277=CARTESIAN_POINT('Ctrl Pts',(-0.766947301194431,-0.194262749649077,
-4.33677034492878));
#48278=CARTESIAN_POINT('Ctrl Pts',(-0.783005614632164,-0.130864696367882,
-4.33940251301129));
#48279=CARTESIAN_POINT('Ctrl Pts',(-0.79103338314962,-0.0654325584305906,
-4.34203468109379));
#48280=CARTESIAN_POINT('Ctrl Pts',(-0.791032667499796,-2.47978686473971E-7,
-4.34466684917629));
#48281=CARTESIAN_POINT('Ctrl Pts',(-0.791034555886587,-5.04054740280758E-6,
-4.3731331508237));
#48282=CARTESIAN_POINT('Ctrl Pts',(-0.791047980996111,-0.0602175127988069,
-4.37071094641218));
#48283=CARTESIAN_POINT('Ctrl Pts',(-0.784261144919877,-0.120427006693712,
-4.36828874200067));
#48284=CARTESIAN_POINT('Ctrl Pts',(-0.770641079578282,-0.179048884627327,
-4.36586653758915));
#48285=CARTESIAN_POINT('Ctrl Pts',(-0.740918797240146,-0.306976024728015,
-4.3605807007305));
#48286=CARTESIAN_POINT('Ctrl Pts',(-0.678655438040537,-0.427342649731578,
-4.35529486387185));
#48287=CARTESIAN_POINT('Ctrl Pts',(-0.591418837274813,-0.525518729957724,
-4.3500090270132));
#48288=CARTESIAN_POINT('Ctrl Pts',(-0.504182236509089,-0.623694810183869,
-4.34472319015456));
#48289=CARTESIAN_POINT('Ctrl Pts',(-0.39197239417725,-0.6996803456326,-4.33943735329591));
#48290=CARTESIAN_POINT('Ctrl Pts',(-0.268427919185097,-0.744239631316306,
-4.33415151643726));
#48291=CARTESIAN_POINT('Ctrl Pts',(-0.144883444192945,-0.788798917000011,
-4.32886567957861));
#48292=CARTESIAN_POINT('Ctrl Pts',(-0.0100043365404776,-0.80193195291869,
-4.32357984271997));
#48293=CARTESIAN_POINT('Ctrl Pts',(0.119815446160315,-0.782042476775574,
-4.31829400586132));
#48294=CARTESIAN_POINT('Ctrl Pts',(0.249635228861107,-0.762153000632459,
-4.31300816900267));
#48295=CARTESIAN_POINT('Ctrl Pts',(0.374395686610229,-0.709241012427549,
-4.30772233214402));
#48296=CARTESIAN_POINT('Ctrl Pts',(0.478932738835162,-0.629737729766704,
-4.30243649528538));
#48297=CARTESIAN_POINT('Ctrl Pts',(0.583469791060094,-0.550234447105859,
-4.29715065842673));
#48298=CARTESIAN_POINT('Ctrl Pts',(0.667783437760838,-0.44413986998908,
-4.29186482156808));
#48299=CARTESIAN_POINT('Ctrl Pts',(0.721625728945871,-0.324349323944434,
-4.28657898470943));
#48300=CARTESIAN_POINT('Ctrl Pts',(0.775468020130904,-0.204558777899789,
-4.28129314785078));
#48301=CARTESIAN_POINT('Ctrl Pts',(0.798838955800226,-0.0710722629272758,
-4.27600731099214));
#48302=CARTESIAN_POINT('Ctrl Pts',(0.788897902327297,0.0598855268279594,
-4.27072147413349));
#48303=CARTESIAN_POINT('Ctrl Pts',(0.778956848854367,0.190843316583198,
-4.26543563727484));
#48304=CARTESIAN_POINT('Ctrl Pts',(0.735703806239186,0.319272381121158,
-4.26014980041619));
#48305=CARTESIAN_POINT('Ctrl Pts',(0.664395990069578,0.429562736977192,
-4.25486396355754));
#48306=CARTESIAN_POINT('Ctrl Pts',(0.593088173899971,0.539853092833225,
-4.2495781266989));
#48307=CARTESIAN_POINT('Ctrl Pts',(0.493725584175939,0.632004740007326,
-4.24429228984025));
#48308=CARTESIAN_POINT('Ctrl Pts',(0.378385303201064,0.694817054296532,
-4.2390064529816));
#48309=CARTESIAN_POINT('Ctrl Pts',(0.263045022226192,0.757629368585737,
-4.23372061612296));
#48310=CARTESIAN_POINT('Ctrl Pts',(0.131727050000475,0.791102349990045,
-4.2284347792643));
#48311=CARTESIAN_POINT('Ctrl Pts',(0.000392503911405343,0.791167506006503,
-4.22314894240566));
#48312=CARTESIAN_POINT('Ctrl Pts',(-0.130942042177665,0.791232662022961,
-4.21786310554701));
#48313=CARTESIAN_POINT('Ctrl Pts',(-0.262293162130093,0.75788999265157,
-4.21257726868836));
#48314=CARTESIAN_POINT('Ctrl Pts',(-0.377695709599153,0.695192151545358,
-4.20729143182972));
#48315=CARTESIAN_POINT('Ctrl Pts',(-0.493098257068215,0.632494310439145,
-4.20200559497107));
#48316=CARTESIAN_POINT('Ctrl Pts',(-0.592552232053908,0.540441297598112,
-4.19671975811242));
#48317=CARTESIAN_POINT('Ctrl Pts',(-0.663969444779212,0.430221748659288,
-4.19143392125377));
#48318=CARTESIAN_POINT('Ctrl Pts',(-0.735386657504514,0.320002199720466,
-4.18614808439512));
#48319=CARTESIAN_POINT('Ctrl Pts',(-0.778767107969428,0.191616114683848,
-4.18086224753648));
#48320=CARTESIAN_POINT('Ctrl Pts',(-0.788838094726788,0.0606682530462416,
-4.17557641067783));
#48321=CARTESIAN_POINT('Ctrl Pts',(-0.790389790846925,0.0404923463810076,
-4.17476199072645));
#48322=CARTESIAN_POINT('Ctrl Pts',(-0.791150741084666,0.0202556247378911,
-4.17394757077508));
#48323=CARTESIAN_POINT('Ctrl Pts',(-0.791131276639148,1.74428956908455E-5,
-4.1731331508237));
#48324=CARTESIAN_POINT('Origin',(0.,0.,-2.94));
#48325=CARTESIAN_POINT('',(-0.791082780681432,-2.0004826913167E-5,-3.9446668491763));
#48326=CARTESIAN_POINT('',(-0.791098791730102,-2.0404891719479E-5,-3.9731331508237));
#48327=CARTESIAN_POINT('',(-0.7911,-9.68818082805471E-17,-2.94));
#48328=CARTESIAN_POINT('Ctrl Pts',(-0.791082780681432,-2.0004826913167E-5,
-3.9446668491763));
#48329=CARTESIAN_POINT('Ctrl Pts',(-0.790990652476222,0.0954469785790556,
-3.94850792981958));
#48330=CARTESIAN_POINT('Ctrl Pts',(-0.773688524716814,0.190946450742593,
-3.95234901046286));
#48331=CARTESIAN_POINT('Ctrl Pts',(-0.739888619060256,0.280198162191953,
-3.95619009110614));
#48332=CARTESIAN_POINT('Ctrl Pts',(-0.693375462027023,0.403020365079478,
-3.96147592796479));
#48333=CARTESIAN_POINT('Ctrl Pts',(-0.615619780996831,0.514010925229607,
-3.96676176482343));
#48334=CARTESIAN_POINT('Ctrl Pts',(-0.516072434305609,0.59967943208061,
-3.97204760168208));
#48335=CARTESIAN_POINT('Ctrl Pts',(-0.416525087614387,0.685347938931613,
-3.97733343854073));
#48336=CARTESIAN_POINT('Ctrl Pts',(-0.295186075262136,0.745694392483489,
-3.98261927539938));
#48337=CARTESIAN_POINT('Ctrl Pts',(-0.166803616300752,0.773383948824665,
-3.98790511225803));
#48338=CARTESIAN_POINT('Ctrl Pts',(-0.0384211573393675,0.801073505165841,
-3.99319094911668));
#48339=CARTESIAN_POINT('Ctrl Pts',(0.0970047482311494,0.796106164296317,
-3.99847678597532));
#48340=CARTESIAN_POINT('Ctrl Pts',(0.223013681935846,0.759085684478411,
-4.00376262283397));
#48341=CARTESIAN_POINT('Ctrl Pts',(0.349022615640543,0.722065204660505,
-4.00904845969262));
#48342=CARTESIAN_POINT('Ctrl Pts',(0.46561457747942,0.652991585894218,-4.01433429655127));
#48343=CARTESIAN_POINT('Ctrl Pts',(0.558618331346661,0.560260420335145,
-4.01962013340991));
#48344=CARTESIAN_POINT('Ctrl Pts',(0.6516220852139,0.467529254776075,-4.02490597026856));
#48345=CARTESIAN_POINT('Ctrl Pts',(0.721037631109505,0.351140542424221,
-4.03019180712721));
#48346=CARTESIAN_POINT('Ctrl Pts',(0.758427817151085,0.225240815311261,
-4.03547764398585));
#48347=CARTESIAN_POINT('Ctrl Pts',(0.795818003192665,0.0993410881982974,
-4.0407634808445));
#48348=CARTESIAN_POINT('Ctrl Pts',(0.801182829380219,-0.036069653675772,
-4.04604931770315));
#48349=CARTESIAN_POINT('Ctrl Pts',(0.773870224873085,-0.164532834916077,
-4.0513351545618));
#48350=CARTESIAN_POINT('Ctrl Pts',(0.746557620365952,-0.292996016156382,
-4.05662099142045));
#48351=CARTESIAN_POINT('Ctrl Pts',(0.686567585164131,-0.414511636762924,
-4.0619068282791));
#48352=CARTESIAN_POINT('Ctrl Pts',(0.601191642108759,-0.514310011733404,
-4.06719266513774));
#48353=CARTESIAN_POINT('Ctrl Pts',(0.515815699053388,-0.614108386703885,
-4.07247850199639));
#48354=CARTESIAN_POINT('Ctrl Pts',(0.405053848144467,-0.692189516038305,
-4.07776433885504));
#48355=CARTESIAN_POINT('Ctrl Pts',(0.282368701349333,-0.739062984602079,
-4.08305017571368));
#48356=CARTESIAN_POINT('Ctrl Pts',(0.159683554554199,-0.785936453165852,
-4.08833601257233));
#48357=CARTESIAN_POINT('Ctrl Pts',(0.0250751118728523,-0.801602260958979,
-4.09362184943098));
#48358=CARTESIAN_POINT('Ctrl Pts',(-0.105095567210095,-0.784156298491206,
-4.09890768628963));
#48359=CARTESIAN_POINT('Ctrl Pts',(-0.235266246293042,-0.766710336023433,
-4.10419352314828));
#48360=CARTESIAN_POINT('Ctrl Pts',(-0.360999161777591,-0.716152603294759,
-4.10947936000693));
#48361=CARTESIAN_POINT('Ctrl Pts',(-0.467012035164418,-0.638628168594394,
-4.11476519686557));
#48362=CARTESIAN_POINT('Ctrl Pts',(-0.573024908551245,-0.561103733894028,
-4.12005103372422));
#48363=CARTESIAN_POINT('Ctrl Pts',(-0.659317739840351,-0.456612597221972,
-4.12533687058287));
#48364=CARTESIAN_POINT('Ctrl Pts',(-0.715402017927282,-0.337855193028336,
-4.13062270744152));
#48365=CARTESIAN_POINT('Ctrl Pts',(-0.76507283774313,-0.23267816611971,
-4.13530408801978));
#48366=CARTESIAN_POINT('Ctrl Pts',(-0.791049006691502,-0.116311122071119,
-4.13998546859804));
#48367=CARTESIAN_POINT('Ctrl Pts',(-0.79114572203675,1.41578566767164E-5,
-4.1446668491763));
#48368=CARTESIAN_POINT('Ctrl Pts',(-0.791131276639148,1.74428956908455E-5,
-4.1731331508237));
#48369=CARTESIAN_POINT('Ctrl Pts',(-0.791024410825469,-0.111096422019725,
-4.16866173391643));
#48370=CARTESIAN_POINT('Ctrl Pts',(-0.767393123498328,-0.222254302430152,
-4.16419031700916));
#48371=CARTESIAN_POINT('Ctrl Pts',(-0.721947197732644,-0.323633156993923,
-4.15971890010188));
#48372=CARTESIAN_POINT('Ctrl Pts',(-0.668223790931328,-0.443477067157891,
-4.15443306324324));
#48373=CARTESIAN_POINT('Ctrl Pts',(-0.584015454278886,-0.549655249247222,
-4.14914722638459));
#48374=CARTESIAN_POINT('Ctrl Pts',(-0.479557337797311,-0.629262215920062,
-4.14386138952594));
#48375=CARTESIAN_POINT('Ctrl Pts',(-0.375099221315737,-0.7088691825929,
-4.13857555266729));
#48376=CARTESIAN_POINT('Ctrl Pts',(-0.250391325005029,-0.761904933849247,
-4.13328971580864));
#48377=CARTESIAN_POINT('Ctrl Pts',(-0.120591340827875,-0.781923209232982,
-4.12800387895));
#48378=CARTESIAN_POINT('Ctrl Pts',(0.0092086433492808,-0.801941484616718,
-4.12271804209135));
#48379=CARTESIAN_POINT('Ctrl Pts',(0.144100715392882,-0.788942284127844,
-4.1174322052327));
#48380=CARTESIAN_POINT('Ctrl Pts',(0.26768934192668,-0.744505602959932,
-4.11214636837406));
#48381=CARTESIAN_POINT('Ctrl Pts',(0.391277968460475,-0.700068921792021,
-4.10686053151541));
#48382=CARTESIAN_POINT('Ctrl Pts',(0.503563149484464,-0.624194759945072,
-4.10157469465676));
#48383=CARTESIAN_POINT('Ctrl Pts',(0.590897119008789,-0.526105285439125,
-4.09628885779811));
#48384=CARTESIAN_POINT('Ctrl Pts',(0.678231088533113,-0.42801581093318,
-4.09100302093946));
#48385=CARTESIAN_POINT('Ctrl Pts',(0.740613846557776,-0.307711023768233,
-4.08571718408082));
#48386=CARTESIAN_POINT('Ctrl Pts',(0.770463045389535,-0.179813437509422,
-4.08043134722217));
#48387=CARTESIAN_POINT('Ctrl Pts',(0.800312244221295,-0.0519158512506065,
-4.07514551036352));
#48388=CARTESIAN_POINT('Ctrl Pts',(0.79762788386015,0.0835745341020731,
-4.06985967350487));
#48389=CARTESIAN_POINT('Ctrl Pts',(0.762736236408148,0.21018946284199,-4.06457383664622));
#48390=CARTESIAN_POINT('Ctrl Pts',(0.727844588956147,0.336804391581905,
-4.05928799978757));
#48391=CARTESIAN_POINT('Ctrl Pts',(0.660745654413287,0.454543863709056,
-4.05400216292893));
#48392=CARTESIAN_POINT('Ctrl Pts',(0.569595010821645,0.549097168329032,
-4.04871632607028));
#48393=CARTESIAN_POINT('Ctrl Pts',(0.478444367230003,0.643650472949008,
-4.04343048921163));
#48394=CARTESIAN_POINT('Ctrl Pts',(0.363242014589576,0.715017610061812,
-4.03814465235298));
#48395=CARTESIAN_POINT('Ctrl Pts',(0.23799028816829,0.754524220524063,-4.03285881549434));
#48396=CARTESIAN_POINT('Ctrl Pts',(0.112738561747003,0.794030830986314,
-4.02757297863569));
#48397=CARTESIAN_POINT('Ctrl Pts',(-0.0225625384551408,0.801676914798013,
-4.02228714177704));
#48398=CARTESIAN_POINT('Ctrl Pts',(-0.151467763502455,0.776533124367168,
-4.01700130491839));
#48399=CARTESIAN_POINT('Ctrl Pts',(-0.280372988549768,0.751389333936323,
-4.01171546805975));
#48400=CARTESIAN_POINT('Ctrl Pts',(-0.40288233844225,0.693455669262934,
-4.0064296312011));
#48401=CARTESIAN_POINT('Ctrl Pts',(-0.504105344788126,0.609773710466362,
-4.00114379434245));
#48402=CARTESIAN_POINT('Ctrl Pts',(-0.605328351134004,0.526091751669789,
-3.9958579574838));
#48403=CARTESIAN_POINT('Ctrl Pts',(-0.685265013933277,0.416661498750035,
-3.99057212062515));
#48404=CARTESIAN_POINT('Ctrl Pts',(-0.734199386184346,0.294783713841862,
-3.98528628376651));
#48405=CARTESIAN_POINT('Ctrl Pts',(-0.771702494165381,0.201377064943841,
-3.98123523945224));
#48406=CARTESIAN_POINT('Ctrl Pts',(-0.790996008268795,0.100659198123538,
-3.97718419513797));
#48407=CARTESIAN_POINT('Ctrl Pts',(-0.791098791730102,-2.0404891719479E-5,
-3.9731331508237));
#48408=CARTESIAN_POINT('Origin',(0.,0.,-2.94));
#48409=CARTESIAN_POINT('',(-0.791059421552401,1.68056895702706E-5,-3.7446668491763));
#48410=CARTESIAN_POINT('',(-0.791048214887112,1.35633341352688E-5,-3.7731331508237));
#48411=CARTESIAN_POINT('',(-0.7911,-9.68818082805471E-17,-2.94));
#48412=CARTESIAN_POINT('Ctrl Pts',(-0.791059421552401,1.68056895702706E-5,
-3.7446668491763));
#48413=CARTESIAN_POINT('Ctrl Pts',(-0.791093925544372,0.0445560275500737,
-3.74645871732382));
#48414=CARTESIAN_POINT('Ctrl Pts',(-0.787395328553636,0.0890895801141432,
-3.74825058547135));
#48415=CARTESIAN_POINT('Ctrl Pts',(-0.77991221789656,0.132977859383846,
-3.75004245361888));
#48416=CARTESIAN_POINT('Ctrl Pts',(-0.757837768845652,0.262444017117988,
-3.75532829047752));
#48417=CARTESIAN_POINT('Ctrl Pts',(-0.702830760007432,0.386295054067948,
-3.76061412733617));
#48418=CARTESIAN_POINT('Ctrl Pts',(-0.621577049458446,0.489477425727861,
-3.76589996419482));
#48419=CARTESIAN_POINT('Ctrl Pts',(-0.54032333890946,0.592659797387773,
-3.77118580105346));
#48420=CARTESIAN_POINT('Ctrl Pts',(-0.43282292664971,0.675173503757637,
-3.77647163791212));
#48421=CARTESIAN_POINT('Ctrl Pts',(-0.31214201123678,0.726989369613957,
-3.78175747477076));
#48422=CARTESIAN_POINT('Ctrl Pts',(-0.191461095823851,0.778805235470277,
-3.78704331162941));
#48423=CARTESIAN_POINT('Ctrl Pts',(-0.0575996772577453,0.799923260813052,
-3.79232914848806));
#48424=CARTESIAN_POINT('Ctrl Pts',(0.0731719824465547,0.787776643278716,
-3.7976149853467));
#48425=CARTESIAN_POINT('Ctrl Pts',(0.203943642150855,0.77563002574438,-3.80290082220535));
#48426=CARTESIAN_POINT('Ctrl Pts',(0.331625542993347,0.730218765332932,
-3.808186659064));
#48427=CARTESIAN_POINT('Ctrl Pts',(0.440698515944364,0.657062399437889,
-3.81347249592265));
#48428=CARTESIAN_POINT('Ctrl Pts',(0.549771488895381,0.583906033542846,
-3.8187583327813));
#48429=CARTESIAN_POINT('Ctrl Pts',(0.640235533954922,0.483004562164209,
-3.82404416963994));
#48430=CARTESIAN_POINT('Ctrl Pts',(0.701095147475853,0.36662211184877,-3.82933000649859));
#48431=CARTESIAN_POINT('Ctrl Pts',(0.761954760996783,0.250239661533333,
-3.83461584335724));
#48432=CARTESIAN_POINT('Ctrl Pts',(0.793209942979106,0.11837623228109,-3.83990168021589));
#48433=CARTESIAN_POINT('Ctrl Pts',(0.791061764608035,-0.0129407606369183,
-3.84518751707453));
#48434=CARTESIAN_POINT('Ctrl Pts',(0.788913586236965,-0.144257753554929,
-3.85047335393318));
#48435=CARTESIAN_POINT('Ctrl Pts',(0.753362047512502,-0.275028310138708,
-3.85575919079183));
#48436=CARTESIAN_POINT('Ctrl Pts',(0.688728280365558,-0.38935784894534,
-3.86104502765048));
#48437=CARTESIAN_POINT('Ctrl Pts',(0.624094513218613,-0.503687387751972,
-3.86633086450913));
#48438=CARTESIAN_POINT('Ctrl Pts',(0.530378517649187,-0.601575908781457,
-3.87161670136777));
#48439=CARTESIAN_POINT('Ctrl Pts',(0.418971057472893,-0.671125496245439,
-3.87690253822642));
#48440=CARTESIAN_POINT('Ctrl Pts',(0.307563597296602,-0.74067508370942,
-3.88218837508507));
#48441=CARTESIAN_POINT('Ctrl Pts',(0.178464672513446,-0.781885737607901,
-3.88747421194372));
#48442=CARTESIAN_POINT('Ctrl Pts',(0.0473656851313694,-0.789748485647599,
-3.89276004880236));
#48443=CARTESIAN_POINT('Ctrl Pts',(-0.0837333022507111,-0.797611233687299,
-3.89804588566101));
#48444=CARTESIAN_POINT('Ctrl Pts',(-0.216832352231711,-0.772126075868214,
-3.90333172251966));
#48445=CARTESIAN_POINT('Ctrl Pts',(-0.335753865318564,-0.716390620146778,
-3.90861755937831));
#48446=CARTESIAN_POINT('Ctrl Pts',(-0.454675378405417,-0.660655164425341,
-3.91390339623696));
#48447=CARTESIAN_POINT('Ctrl Pts',(-0.559419354598121,-0.574669410801554,
-3.91918923309561));
#48448=CARTESIAN_POINT('Ctrl Pts',(-0.637254627923676,-0.468884546450935,
-3.92447506995425));
#48449=CARTESIAN_POINT('Ctrl Pts',(-0.71508990124923,-0.363099682100315,
-3.9297609068129));
#48450=CARTESIAN_POINT('Ctrl Pts',(-0.766016471707633,-0.237515707022865,
-3.93504674367155));
#48451=CARTESIAN_POINT('Ctrl Pts',(-0.783844440418698,-0.107396796671679,
-3.94033258053019));
#48452=CARTESIAN_POINT('Ctrl Pts',(-0.788717286344795,-0.0718319259626912,
-3.94177733674556));
#48453=CARTESIAN_POINT('Ctrl Pts',(-0.791117433116371,-0.0359282635819957,
-3.94322209296093));
#48454=CARTESIAN_POINT('Ctrl Pts',(-0.791082780681432,-2.0004826913167E-5,
-3.9446668491763));
#48455=CARTESIAN_POINT('Ctrl Pts',(-0.791098791730102,-2.0404891719479E-5,
-3.9731331508237));
#48456=CARTESIAN_POINT('Ctrl Pts',(-0.791130120997783,-0.0307083987841548,
-3.97189835827932));
#48457=CARTESIAN_POINT('Ctrl Pts',(-0.789378474176348,-0.0613928376556407,
-3.97066356573494));
#48458=CARTESIAN_POINT('Ctrl Pts',(-0.785816066255412,-0.0918655900473206,
-3.96942877319056));
#48459=CARTESIAN_POINT('Ctrl Pts',(-0.770566292372547,-0.222311792131744,
-3.96414293633192));
#48460=CARTESIAN_POINT('Ctrl Pts',(-0.722134662903953,-0.348878879404003,
-3.95885709947327));
#48461=CARTESIAN_POINT('Ctrl Pts',(-0.64640782771266,-0.456183183481889,
-3.95357126261462));
#48462=CARTESIAN_POINT('Ctrl Pts',(-0.570680992521369,-0.563487487559772,
-3.94828542575597));
#48463=CARTESIAN_POINT('Ctrl Pts',(-0.467658951607378,-0.651529008443283,
-3.94299958889732));
#48464=CARTESIAN_POINT('Ctrl Pts',(-0.349863577343953,-0.709606689559761,
-3.93771375203868));
#48465=CARTESIAN_POINT('Ctrl Pts',(-0.232068203080525,-0.767684370676241,
-3.93242791518003));
#48466=CARTESIAN_POINT('Ctrl Pts',(-0.0994994954676606,-0.795798212025687,
-3.92714207832138));
#48467=CARTESIAN_POINT('Ctrl Pts',(0.0317294067653929,-0.790531100821585,
-3.92185624146273));
#48468=CARTESIAN_POINT('Ctrl Pts',(0.162958308998446,-0.785263989617483,
-3.91657040460409));
#48469=CARTESIAN_POINT('Ctrl Pts',(0.292847405851691,-0.746615925859833,
-3.91128456774544));
#48470=CARTESIAN_POINT('Ctrl Pts',(0.405609253404915,-0.679284410370338,
-3.90599873088679));
#48471=CARTESIAN_POINT('Ctrl Pts',(0.518371100958137,-0.611952894880846,
-3.90071289402814));
#48472=CARTESIAN_POINT('Ctrl Pts',(0.614005699211341,-0.515937927659511,
-3.89542705716949));
#48473=CARTESIAN_POINT('Ctrl Pts',(0.680889086697923,-0.402909702334828,
-3.89014122031085));
#48474=CARTESIAN_POINT('Ctrl Pts',(0.747772474184507,-0.289881477010141,
-3.8848553834522));
#48475=CARTESIAN_POINT('Ctrl Pts',(0.785904650904467,-0.159839993582104,
-3.87956954659355));
#48476=CARTESIAN_POINT('Ctrl Pts',(0.790650819818588,-0.0285912178835576,
-3.8742837097349));
#48477=CARTESIAN_POINT('Ctrl Pts',(0.795396988732709,0.102657557814991,
-3.86899787287626));
#48478=CARTESIAN_POINT('Ctrl Pts',(0.766757149840992,0.235113625784043,
-3.86371203601761));
#48479=CARTESIAN_POINT('Ctrl Pts',(0.708212348599448,0.352677538143735,
-3.85842619915896));
#48480=CARTESIAN_POINT('Ctrl Pts',(0.649667547357904,0.470241450503425,
-3.85314036230031));
#48481=CARTESIAN_POINT('Ctrl Pts',(0.561217783766536,0.572913207253749,
-3.84785452544167));
#48482=CARTESIAN_POINT('Ctrl Pts',(0.453613734489391,0.648213511508715,
-3.84256868858302));
#48483=CARTESIAN_POINT('Ctrl Pts',(0.346009685212246,0.723513815763681,
-3.83728285172437));
#48484=CARTESIAN_POINT('Ctrl Pts',(0.219251350249323,0.771442667523289,
-3.83199701486572));
#48485=CARTESIAN_POINT('Ctrl Pts',(0.0887456432918277,0.786174527326211,
-3.82671117800707));
#48486=CARTESIAN_POINT('Ctrl Pts',(-0.041760063665668,0.800906387129132,
-3.82142534114842));
#48487=CARTESIAN_POINT('Ctrl Pts',(-0.176013142617738,0.782441254975367,
-3.81613950428978));
#48488=CARTESIAN_POINT('Ctrl Pts',(-0.297695726965726,0.733023485821715,
-3.81085366743113));
#48489=CARTESIAN_POINT('Ctrl Pts',(-0.419378311313713,0.683605716668064,
-3.80556783057248));
#48490=CARTESIAN_POINT('Ctrl Pts',(-0.528490401057619,0.603235310514526,
-3.80028199371383));
#48491=CARTESIAN_POINT('Ctrl Pts',(-0.611769905386271,0.501680933944618,
-3.79499615685519));
#48492=CARTESIAN_POINT('Ctrl Pts',(-0.695049409714923,0.40012655737471,
-3.78971031999654));
#48493=CARTESIAN_POINT('Ctrl Pts',(-0.752496328628322,0.277388210388431,
-3.78442448313789));
#48494=CARTESIAN_POINT('Ctrl Pts',(-0.777128243796476,0.148384194959152,
-3.77913864627924));
#48495=CARTESIAN_POINT('Ctrl Pts',(-0.786456748033961,0.0995282900744009,
-3.77713681446073));
#48496=CARTESIAN_POINT('Ctrl Pts',(-0.791078729935658,0.0497737258841513,
-3.77513498264221));
#48497=CARTESIAN_POINT('Ctrl Pts',(-0.791048214887112,1.35633341352688E-5,
-3.7731331508237));
#48498=CARTESIAN_POINT('Origin',(0.,0.,-2.94));
#48499=CARTESIAN_POINT('',(-0.791163048520337,-6.61538243201809E-6,-3.54466684917629));
#48500=CARTESIAN_POINT('',(-0.791167436263867,-1.24420514395741E-6,-3.5731331508237));
#48501=CARTESIAN_POINT('',(-0.7911,-9.68818082805471E-17,-2.94));
#48502=CARTESIAN_POINT('Ctrl Pts',(-0.791163048520337,-6.61538243201809E-6,
-3.54466684917629));
#48503=CARTESIAN_POINT('Ctrl Pts',(-0.791107674076706,0.124935935430854,
-3.54969534168672));
#48504=CARTESIAN_POINT('Ctrl Pts',(-0.760988940033902,0.249904240112934,
-3.55472383419714));
#48505=CARTESIAN_POINT('Ctrl Pts',(-0.703968423943417,0.361074281556113,
-3.55975232670756));
#48506=CARTESIAN_POINT('Ctrl Pts',(-0.644029755440748,0.477933698452947,
-3.5650381635662));
#48507=CARTESIAN_POINT('Ctrl Pts',(-0.554365328477183,0.579546398998705,
-3.57032400042485));
#48508=CARTESIAN_POINT('Ctrl Pts',(-0.44587345666502,0.653561809894234,
-3.5756098372835));
#48509=CARTESIAN_POINT('Ctrl Pts',(-0.337381584852852,0.727577220789767,
-3.58089567414214));
#48510=CARTESIAN_POINT('Ctrl Pts',(-0.210062268192083,0.773995342035067,
-3.58618151100079));
#48511=CARTESIAN_POINT('Ctrl Pts',(-0.0793906052124412,0.787174256765707,
-3.59146734785944));
#48512=CARTESIAN_POINT('Ctrl Pts',(0.0512810577672008,0.800353171496347,
-3.59675318471809));
#48513=CARTESIAN_POINT('Ctrl Pts',(0.185305067065716,0.780292879712326,
-3.60203902157673));
#48514=CARTESIAN_POINT('Ctrl Pts',(0.306391398485365,0.72943162095211,-3.60732485843538));
#48515=CARTESIAN_POINT('Ctrl Pts',(0.427477729905014,0.678570362191895,
-3.61261069529403));
#48516=CARTESIAN_POINT('Ctrl Pts',(0.535626383445797,0.596908136455485,
-3.61789653215268));
#48517=CARTESIAN_POINT('Ctrl Pts',(0.61769236969609,0.49437062527002,-3.62318236901133));
#48518=CARTESIAN_POINT('Ctrl Pts',(0.699758355946382,0.391833114084555,
-3.62846820586998));
#48519=CARTESIAN_POINT('Ctrl Pts',(0.755741674906185,0.268420317450034,
-3.63375404272862));
#48520=CARTESIAN_POINT('Ctrl Pts',(0.778837802331684,0.139132513704717,
-3.63903987958727));
#48521=CARTESIAN_POINT('Ctrl Pts',(0.801933929757183,0.00984470995939934,
-3.64432571644592));
#48522=CARTESIAN_POINT('Ctrl Pts',(0.792142865648378,-0.125318100896716,
-3.64961155330457));
#48523=CARTESIAN_POINT('Ctrl Pts',(0.75065467044361,-0.249927478384903,
-3.65489739016321));
#48524=CARTESIAN_POINT('Ctrl Pts',(0.709166475238842,-0.374536855873091,
-3.66018322702186));
#48525=CARTESIAN_POINT('Ctrl Pts',(0.635981148938111,-0.488592799993352,
-3.66546906388051));
#48526=CARTESIAN_POINT('Ctrl Pts',(0.539994043520502,-0.578232316351325,
-3.67075490073916));
#48527=CARTESIAN_POINT('Ctrl Pts',(0.444006938102892,-0.667871832709299,
-3.67604073759781));
#48528=CARTESIAN_POINT('Ctrl Pts',(0.325218053568405,-0.733094921304985,
-3.68132657445645));
#48529=CARTESIAN_POINT('Ctrl Pts',(0.19806565223748,-0.765974004855506,
-3.6866124113151));
#48530=CARTESIAN_POINT('Ctrl Pts',(0.0709132509065556,-0.798853088406027,
-3.69189824817375));
#48531=CARTESIAN_POINT('Ctrl Pts',(-0.0646026672208058,-0.799388166911383,
-3.69718408503239));
#48532=CARTESIAN_POINT('Ctrl Pts',(-0.192010743042395,-0.767514203951268,
-3.70246992189104));
#48533=CARTESIAN_POINT('Ctrl Pts',(-0.31941881886398,-0.735640240991153,
-3.70775575874969));
#48534=CARTESIAN_POINT('Ctrl Pts',(-0.438719052379794,-0.671357236565569,
-3.71304159560834));
#48535=CARTESIAN_POINT('Ctrl Pts',(-0.535411029067541,-0.582478504893938,
-3.71832743246699));
#48536=CARTESIAN_POINT('Ctrl Pts',(-0.632103005755294,-0.493599773222301,
-3.72361326932564));
#48537=CARTESIAN_POINT('Ctrl Pts',(-0.706186725614977,-0.380125314304615,
-3.72889910618428));
#48538=CARTESIAN_POINT('Ctrl Pts',(-0.74865764091302,-0.255847445586608,
-3.73418494304293));
#48539=CARTESIAN_POINT('Ctrl Pts',(-0.776731161370101,-0.173699056145654,
-3.73767891175405));
#48540=CARTESIAN_POINT('Ctrl Pts',(-0.79099214212198,-0.086830347552772,
-3.74117288046517));
#48541=CARTESIAN_POINT('Ctrl Pts',(-0.791059421552401,1.68056895702706E-5,
-3.7446668491763));
#48542=CARTESIAN_POINT('Ctrl Pts',(-0.791048214887112,1.35633341352688E-5,
-3.7731331508237));
#48543=CARTESIAN_POINT('Ctrl Pts',(-0.790998154950857,-0.0816179818839992,
-3.76984914578357));
#48544=CARTESIAN_POINT('Ctrl Pts',(-0.778427108402436,-0.163264593632743,
-3.76656514074343));
#48545=CARTESIAN_POINT('Ctrl Pts',(-0.753573596205868,-0.240983426237628,
-3.7632811357033));
#48546=CARTESIAN_POINT('Ctrl Pts',(-0.713570122024198,-0.366077348132835,
-3.75799529884465));
#48547=CARTESIAN_POINT('Ctrl Pts',(-0.641746262237952,-0.480995508050975,
-3.752709461986));
#48548=CARTESIAN_POINT('Ctrl Pts',(-0.5468318886068,-0.571770113089685,
-3.74742362512736));
#48549=CARTESIAN_POINT('Ctrl Pts',(-0.451917514975644,-0.662544718128397,
-3.74213778826871));
#48550=CARTESIAN_POINT('Ctrl Pts',(-0.333912627499583,-0.729175768287678,
-3.73685195141006));
#48551=CARTESIAN_POINT('Ctrl Pts',(-0.207160197132085,-0.76356455479813,
-3.73156611455141));
#48552=CARTESIAN_POINT('Ctrl Pts',(-0.0804077667645874,-0.797953341308583,
-3.72628027769276));
#48553=CARTESIAN_POINT('Ctrl Pts',(0.0550922064943439,-0.800099864170207,
-3.72099444083412));
#48554=CARTESIAN_POINT('Ctrl Pts',(0.182870301570576,-0.769743223044774,
-3.71570860397547));
#48555=CARTESIAN_POINT('Ctrl Pts',(0.310648396646807,-0.739386581919342,
-3.71042276711682));
#48556=CARTESIAN_POINT('Ctrl Pts',(0.430704613540337,-0.676526776806852,
-3.70513693025817));
#48557=CARTESIAN_POINT('Ctrl Pts',(0.528446651300607,-0.588804138359307,
-3.69985109339953));
#48558=CARTESIAN_POINT('Ctrl Pts',(0.626188689060877,-0.501081499911761,
-3.69456525654088));
#48559=CARTESIAN_POINT('Ctrl Pts',(0.701616547687885,-0.388496028129161,
-3.68927941968223));
#48560=CARTESIAN_POINT('Ctrl Pts',(0.745562305339503,-0.264731988011871,
-3.68399358282358));
#48561=CARTESIAN_POINT('Ctrl Pts',(0.78950806299112,-0.140967947894581,
-3.67870774596493));
#48562=CARTESIAN_POINT('Ctrl Pts',(0.801971719667347,-0.00602533944260349,
-3.67342190910629));
#48563=CARTESIAN_POINT('Ctrl Pts',(0.781438373150955,0.123694161491399,
-3.66813607224764));
#48564=CARTESIAN_POINT('Ctrl Pts',(0.760905026634563,0.253413662425401,
-3.66285023538899));
#48565=CARTESIAN_POINT('Ctrl Pts',(0.707374676925553,0.377910055841426,
-3.65756439853034));
#48566=CARTESIAN_POINT('Ctrl Pts',(0.627353700729391,0.482051357016042,
-3.65227856167169));
#48567=CARTESIAN_POINT('Ctrl Pts',(0.547332724533233,0.586192658190656,
-3.64699272481305));
#48568=CARTESIAN_POINT('Ctrl Pts',(0.440821121849916,0.669978867123868,
-3.6417068879544));
#48569=CARTESIAN_POINT('Ctrl Pts',(0.32076490581645,0.723226141546637,-3.63642105109575));
#48570=CARTESIAN_POINT('Ctrl Pts',(0.200708689782987,0.776473415969404,
-3.6311352142371));
#48571=CARTESIAN_POINT('Ctrl Pts',(0.067107860399371,0.799181755881737,
-3.62584937737845));
#48572=CARTESIAN_POINT('Ctrl Pts',(-0.063798993779351,0.788591063234052,
-3.62056354051981));
#48573=CARTESIAN_POINT('Ctrl Pts',(-0.19470584795808,0.778000370586367,
-3.61527770366116));
#48574=CARTESIAN_POINT('Ctrl Pts',(-0.322918726931912,0.73411064537866,
-3.60999186680251));
#48575=CARTESIAN_POINT('Ctrl Pts',(-0.432853923633158,0.662256489145445,
-3.60470602994387));
#48576=CARTESIAN_POINT('Ctrl Pts',(-0.542789120334404,0.59040233291223,
-3.59942019308522));
#48577=CARTESIAN_POINT('Ctrl Pts',(-0.634446634763061,0.490583745653509,
-3.59413435622657));
#48578=CARTESIAN_POINT('Ctrl Pts',(-0.696685902360868,0.374933234151754,
-3.58884851936792));
#48579=CARTESIAN_POINT('Ctrl Pts',(-0.75836727558384,0.26031937960796,-3.58361006318651));
#48580=CARTESIAN_POINT('Ctrl Pts',(-0.791155431195283,0.130156154124652,
-3.57837160700511));
#48581=CARTESIAN_POINT('Ctrl Pts',(-0.791167436263867,-1.24420514395741E-6,
-3.5731331508237));
#48582=CARTESIAN_POINT('Origin',(0.,0.,-2.94));
#48583=CARTESIAN_POINT('',(-0.791037041324519,-7.57978170876084E-6,-3.3446668491763));
#48584=CARTESIAN_POINT('',(-0.791044053170824,-1.18405052558484E-5,-3.3731331508237));
#48585=CARTESIAN_POINT('',(-0.7911,-9.68818082805471E-17,-2.94));
#48586=CARTESIAN_POINT('Ctrl Pts',(-0.791037041324519,-7.57978170876084E-6,
-3.3446668491763));
#48587=CARTESIAN_POINT('Ctrl Pts',(-0.791012114368536,0.0740523149147727,
-3.34764612919096));
#48588=CARTESIAN_POINT('Ctrl Pts',(-0.780696222431574,0.148119012240718,
-3.35062540920562));
#48589=CARTESIAN_POINT('Ctrl Pts',(-0.760182848009542,0.219244649427855,
-3.35360468922029));
#48590=CARTESIAN_POINT('Ctrl Pts',(-0.723788031113677,0.345435713305053,
-3.35889052607894));
#48591=CARTESIAN_POINT('Ctrl Pts',(-0.655293746461191,0.46236895641775,
-3.36417636293758));
#48592=CARTESIAN_POINT('Ctrl Pts',(-0.563025170714357,0.555831661434206,
-3.36946219979623));
#48593=CARTESIAN_POINT('Ctrl Pts',(-0.470756594967522,0.649294366450663,
-3.37474803665488));
#48594=CARTESIAN_POINT('Ctrl Pts',(-0.354713728126337,0.71928653337088,
-3.38003387351353));
#48595=CARTESIAN_POINT('Ctrl Pts',(-0.229001066233802,0.757300924583103,
-3.38531971037218));
#48596=CARTESIAN_POINT('Ctrl Pts',(-0.103288404341268,0.795315315795325,
-3.39060554723082));
#48597=CARTESIAN_POINT('Ctrl Pts',(0.0320940526026171,0.801351931299553,
-3.39589138408947));
#48598=CARTESIAN_POINT('Ctrl Pts',(0.160691167110856,0.774677047241747,
-3.40117722094812));
#48599=CARTESIAN_POINT('Ctrl Pts',(0.289288281619095,0.748002163183941,
-3.40646305780677));
#48600=CARTESIAN_POINT('Ctrl Pts',(0.41110005369169,0.6886157795641,-3.41174889466542));
#48601=CARTESIAN_POINT('Ctrl Pts',(0.511320802428493,0.603736048049579,
-3.41703473152406));
#48602=CARTESIAN_POINT('Ctrl Pts',(0.611541551165295,0.518856316535058,
-3.42232056838271));
#48603=CARTESIAN_POINT('Ctrl Pts',(0.690171276566308,0.408483237125855,
-3.42760640524136));
#48604=CARTESIAN_POINT('Ctrl Pts',(0.73765288407699,0.286032168336954,-3.43289224210001));
#48605=CARTESIAN_POINT('Ctrl Pts',(0.785134491587671,0.163581099548057,
-3.43817807895865));
#48606=CARTESIAN_POINT('Ctrl Pts',(0.801467981208026,0.0290520413794619,
-3.4434639158173));
#48607=CARTESIAN_POINT('Ctrl Pts',(0.784668089681554,-0.101203595519831,
-3.44874975267595));
#48608=CARTESIAN_POINT('Ctrl Pts',(0.767868198155081,-0.231459232419131,
-3.4540355895346));
#48609=CARTESIAN_POINT('Ctrl Pts',(0.717934925481783,-0.357441448049119,
-3.45932142639325));
#48610=CARTESIAN_POINT('Ctrl Pts',(0.64093743959938,-0.463837662582968,
-3.46460726325189));
#48611=CARTESIAN_POINT('Ctrl Pts',(0.56393995371698,-0.570233877116814,
-3.46989310011054));
#48612=CARTESIAN_POINT('Ctrl Pts',(0.45987825462548,-0.657044090554512,
-3.47517893696919));
#48613=CARTESIAN_POINT('Ctrl Pts',(0.341400580540787,-0.713716906285016,
-3.48046477382784));
#48614=CARTESIAN_POINT('Ctrl Pts',(0.222922906456093,-0.770389722015521,
-3.48575061068648));
#48615=CARTESIAN_POINT('Ctrl Pts',(0.0900292573782051,-0.796925140038832,
-3.49103644754513));
#48616=CARTESIAN_POINT('Ctrl Pts',(-0.0411277327690323,-0.790097897926529,
-3.49632228440378));
#48617=CARTESIAN_POINT('Ctrl Pts',(-0.17228472291627,-0.783270655814226,
-3.50160812126243));
#48618=CARTESIAN_POINT('Ctrl Pts',(-0.301705054132859,-0.743080753566308,
-3.50689395812107));
#48619=CARTESIAN_POINT('Ctrl Pts',(-0.413658258883671,-0.674413095637956,
-3.51217979497972));
#48620=CARTESIAN_POINT('Ctrl Pts',(-0.525611463634484,-0.605745437709604,
-3.51746563183837));
#48621=CARTESIAN_POINT('Ctrl Pts',(-0.620097541919521,-0.508600024100816,
-3.52275146869702));
#48622=CARTESIAN_POINT('Ctrl Pts',(-0.685632129782885,-0.39478444918718,
-3.52803730555567));
#48623=CARTESIAN_POINT('Ctrl Pts',(-0.751166717646251,-0.28096887427354,
-3.53332314241432));
#48624=CARTESIAN_POINT('Ctrl Pts',(-0.787749815087943,-0.15048313805505,
-3.53860897927296));
#48625=CARTESIAN_POINT('Ctrl Pts',(-0.790934908787902,-0.0191872033218446,
-3.54389481613161));
#48626=CARTESIAN_POINT('Ctrl Pts',(-0.791089977111837,-0.0127949767638775,
-3.54415216047984));
#48627=CARTESIAN_POINT('Ctrl Pts',(-0.791165882431311,-0.00640082979925586,
-3.54440950482807));
#48628=CARTESIAN_POINT('Ctrl Pts',(-0.791163048520337,-6.61538243201809E-6,
-3.54466684917629));
#48629=CARTESIAN_POINT('Ctrl Pts',(-0.791167436263867,-1.24420514395741E-6,
-3.5731331508237));
#48630=CARTESIAN_POINT('Ctrl Pts',(-0.791167544847056,-0.00117848907790079,
-3.57308577014646));
#48631=CARTESIAN_POINT('Ctrl Pts',(-0.79116497207817,-0.0023557334739497,
-3.57303838946922));
#48632=CARTESIAN_POINT('Ctrl Pts',(-0.791159715084089,-0.00353296588344793,
-3.57299100879198));
#48633=CARTESIAN_POINT('Ctrl Pts',(-0.790573239442549,-0.13486621867211,
-3.56770517193333));
#48634=CARTESIAN_POINT('Ctrl Pts',(-0.756579267392514,-0.266050288504648,
-3.56241933507468));
#48635=CARTESIAN_POINT('Ctrl Pts',(-0.693309615540358,-0.381140333235874,
-3.55713349821603));
#48636=CARTESIAN_POINT('Ctrl Pts',(-0.630039963688201,-0.496230377967099,
-3.55184766135739));
#48637=CARTESIAN_POINT('Ctrl Pts',(-0.537494632033922,-0.595226397597014,
-3.54656182449874));
#48638=CARTESIAN_POINT('Ctrl Pts',(-0.426922095383839,-0.666095864791955,
-3.54127598764009));
#48639=CARTESIAN_POINT('Ctrl Pts',(-0.316349558733757,-0.736965331986896,
-3.53599015078144));
#48640=CARTESIAN_POINT('Ctrl Pts',(-0.18774981708787,-0.779708246746866,
-3.53070431392279));
#48641=CARTESIAN_POINT('Ctrl Pts',(-0.0567535989566851,-0.789129397263424,
-3.52541847706415));
#48642=CARTESIAN_POINT('Ctrl Pts',(0.0742426191744998,-0.798550547779982,
-3.5201326402055));
#48643=CARTESIAN_POINT('Ctrl Pts',(0.207635313790985,-0.77464993405313,
-3.51484680334685));
#48644=CARTESIAN_POINT('Ctrl Pts',(0.327211194195991,-0.720332569729222,
-3.50956096648821));
#48645=CARTESIAN_POINT('Ctrl Pts',(0.446787074600998,-0.666015205405313,
-3.50427512962956));
#48646=CARTESIAN_POINT('Ctrl Pts',(0.552546140794528,-0.581281090484348,
-3.49898929277091));
#48647=CARTESIAN_POINT('Ctrl Pts',(0.631633847113903,-0.476429281006071,
-3.49370345591226));
#48648=CARTESIAN_POINT('Ctrl Pts',(0.710721553433278,-0.371577471527794,
-3.48841761905361));
#48649=CARTESIAN_POINT('Ctrl Pts',(0.763137899878498,-0.246607967492202,
-3.48313178219496));
#48650=CARTESIAN_POINT('Ctrl Pts',(0.782511911902399,-0.116710258121227,
-3.47784594533632));
#48651=CARTESIAN_POINT('Ctrl Pts',(0.8018859239263,0.0131874512497518,-3.47256010847767));
#48652=CARTESIAN_POINT('Ctrl Pts',(0.788217601528883,0.148013365956107,
-3.46727427161902));
#48653=CARTESIAN_POINT('Ctrl Pts',(0.743168268705463,0.271379993752664,
-3.46198843476038));
#48654=CARTESIAN_POINT('Ctrl Pts',(0.698118935882044,0.394746621549218,
-3.45670259790173));
#48655=CARTESIAN_POINT('Ctrl Pts',(0.621688592632625,0.506653962435966,
-3.45141676104308));
#48656=CARTESIAN_POINT('Ctrl Pts',(0.523167008361145,0.593500175216756,
-3.44613092418443));
#48657=CARTESIAN_POINT('Ctrl Pts',(0.424645424089665,0.680346387997547,
-3.44084508732578));
#48658=CARTESIAN_POINT('Ctrl Pts',(0.304032598796122,0.74213147267238,-3.43555925046714));
#48659=CARTESIAN_POINT('Ctrl Pts',(0.17598848671464,0.771345726094183,-3.43027341360849));
#48660=CARTESIAN_POINT('Ctrl Pts',(0.0479443746331568,0.800559979515985,
-3.42498757674984));
#48661=CARTESIAN_POINT('Ctrl Pts',(-0.0875310242362685,0.797203401684758,
-3.41970173989119));
#48662=CARTESIAN_POINT('Ctrl Pts',(-0.213971275727604,0.761683969756075,
-3.41441590303254));
#48663=CARTESIAN_POINT('Ctrl Pts',(-0.34041152721894,0.726164537827391,
-3.40913006617389));
#48664=CARTESIAN_POINT('Ctrl Pts',(-0.457816631332189,0.658482251801251,
-3.40384422931525));
#48665=CARTESIAN_POINT('Ctrl Pts',(-0.551916518122767,0.566863593506508,
-3.3985583924566));
#48666=CARTESIAN_POINT('Ctrl Pts',(-0.646016404913346,0.475244935211765,
-3.39327255559795));
#48667=CARTESIAN_POINT('Ctrl Pts',(-0.716811074381257,0.359689904648418,
-3.38798671873931));
#48668=CARTESIAN_POINT('Ctrl Pts',(-0.755695748287589,0.234243703522489,
-3.38270088188066));
#48669=CARTESIAN_POINT('Ctrl Pts',(-0.779157066531176,0.158554930764511,
-3.37951163819501));
#48670=CARTESIAN_POINT('Ctrl Pts',(-0.791001902275285,0.0792653862822654,
-3.37632239450935));
#48671=CARTESIAN_POINT('Ctrl Pts',(-0.791044053170824,-1.18405052558484E-5,
-3.3731331508237));
#48672=CARTESIAN_POINT('Origin',(0.,0.,-2.94));
#48673=CARTESIAN_POINT('',(-0.791122594563005,1.8755956602709E-5,-3.1446668491763));
#48674=CARTESIAN_POINT('',(-0.791106220557104,2.01772645531753E-5,-3.1731331508237));
#48675=CARTESIAN_POINT('',(-0.7911,-9.68818082805471E-17,-2.94));
#48676=CARTESIAN_POINT('Ctrl Pts',(-0.791122594563005,1.8755956602709E-5,
-3.1446668491763));
#48677=CARTESIAN_POINT('Ctrl Pts',(-0.791145783735659,0.0231314904601002,
-3.1455969166952));
#48678=CARTESIAN_POINT('Ctrl Pts',(-0.790153058855057,0.046242239724187,
-3.14652698421411));
#48679=CARTESIAN_POINT('Ctrl Pts',(-0.788129997515042,0.0692624409588715,
-3.14745705173302));
#48680=CARTESIAN_POINT('Ctrl Pts',(-0.776632367524814,0.200092757796941,
-3.15274288859167));
#48681=CARTESIAN_POINT('Ctrl Pts',(-0.731855173927621,0.32799840000426,
-3.15802872545032));
#48682=CARTESIAN_POINT('Ctrl Pts',(-0.659240886106545,0.437433003780121,
-3.16331456230897));
#48683=CARTESIAN_POINT('Ctrl Pts',(-0.586626598285466,0.546867607555985,
-3.16860039916762));
#48684=CARTESIAN_POINT('Ctrl Pts',(-0.486175216240504,0.637831172900387,
-3.17388623602626));
#48685=CARTESIAN_POINT('Ctrl Pts',(-0.3700961601552,0.699267481689959,-3.17917207288491));
#48686=CARTESIAN_POINT('Ctrl Pts',(-0.2540171040699,0.76070379047953,-3.18445790974356));
#48687=CARTESIAN_POINT('Ctrl Pts',(-0.122310373944261,0.792612842714271,
-3.18974374660221));
#48688=CARTESIAN_POINT('Ctrl Pts',(0.00901566103487368,0.791116234548847,
-3.19502958346085));
#48689=CARTESIAN_POINT('Ctrl Pts',(0.140341696014012,0.789619626383422,
-3.2003154203195));
#48690=CARTESIAN_POINT('Ctrl Pts',(0.271287035846645,0.754717357817829,
-3.20560125717815));
#48691=CARTESIAN_POINT('Ctrl Pts',(0.385935854960777,0.690651644873401,
-3.2108870940368));
#48692=CARTESIAN_POINT('Ctrl Pts',(0.500584674074912,0.626585931928972,
-3.21617293089545));
#48693=CARTESIAN_POINT('Ctrl Pts',(0.598936972470544,0.533356774605708,
-3.22145876775409));
#48694=CARTESIAN_POINT('Ctrl Pts',(0.669038464276404,0.422295763688569,
-3.22674460461274));
#48695=CARTESIAN_POINT('Ctrl Pts',(0.739139956082262,0.311234752771435,
-3.23203044147139));
#48696=CARTESIAN_POINT('Ctrl Pts',(0.780990641298351,0.182341888260418,
-3.23731627833004));
#48697=CARTESIAN_POINT('Ctrl Pts',(0.789503754662005,0.051283526450878,
-3.24260211518869));
#48698=CARTESIAN_POINT('Ctrl Pts',(0.798016868025659,-0.0797748353586617,
-3.24788795204733));
#48699=CARTESIAN_POINT('Ctrl Pts',(0.773192409536883,-0.212998694466734,
-3.25317378890598));
#48700=CARTESIAN_POINT('Ctrl Pts',(0.71804768207741,-0.332195281384159,
-3.25845962576463));
#48701=CARTESIAN_POINT('Ctrl Pts',(0.662902954617938,-0.45139186830158,
-3.26374546262328));
#48702=CARTESIAN_POINT('Ctrl Pts',(0.577437958187772,-0.556561183028352,
-3.26903129948193));
#48703=CARTESIAN_POINT('Ctrl Pts',(0.472040584234078,-0.6349203615782,-3.27431713634057));
#48704=CARTESIAN_POINT('Ctrl Pts',(0.366643210280383,-0.713279540128047,
-3.27960297319922));
#48705=CARTESIAN_POINT('Ctrl Pts',(0.241313458803161,-0.764828582500967,
-3.28488881005787));
#48706=CARTESIAN_POINT('Ctrl Pts',(0.111284605503879,-0.783301931115,-3.29017464691652));
#48707=CARTESIAN_POINT('Ctrl Pts',(-0.0187442477954065,-0.801775279729033,
-3.29546048377516));
#48708=CARTESIAN_POINT('Ctrl Pts',(-0.153472202916751,-0.787172934584176,
-3.30074632063381));
#48709=CARTESIAN_POINT('Ctrl Pts',(-0.276523674168264,-0.741269746000149,
-3.30603215749246));
#48710=CARTESIAN_POINT('Ctrl Pts',(-0.399575145419777,-0.695366557416121,
-3.31131799435111));
#48711=CARTESIAN_POINT('Ctrl Pts',(-0.510950132801457,-0.618162525392924,
-3.31660383120975));
#48712=CARTESIAN_POINT('Ctrl Pts',(-0.597111500325757,-0.519041457775161,
-3.3218896680684));
#48713=CARTESIAN_POINT('Ctrl Pts',(-0.683272867850058,-0.419920390157398,
-3.32717550492705));
#48714=CARTESIAN_POINT('Ctrl Pts',(-0.744220615516977,-0.298882286945071,
-3.3324613417857));
#48715=CARTESIAN_POINT('Ctrl Pts',(-0.772546814780815,-0.170638793018057,
-3.33774717864434));
#48716=CARTESIAN_POINT('Ctrl Pts',(-0.78490739088697,-0.114677756662999,
-3.34005373548833));
#48717=CARTESIAN_POINT('Ctrl Pts',(-0.791056339759254,-0.0573447069184797,
-3.34236029233231));
#48718=CARTESIAN_POINT('Ctrl Pts',(-0.791037041324519,-7.57978170876084E-6,
-3.3446668491763));
#48719=CARTESIAN_POINT('Ctrl Pts',(-0.791044053170824,-1.18405052558484E-5,
-3.3731331508237));
#48720=CARTESIAN_POINT('Ctrl Pts',(-0.791071762963029,-0.0521283009703081,
-3.3710365576507));
#48721=CARTESIAN_POINT('Ctrl Pts',(-0.78599872629567,-0.104239438117949,
-3.36893996447771));
#48722=CARTESIAN_POINT('Ctrl Pts',(-0.775772042088009,-0.155318753968962,
-3.36684337130471));
#48723=CARTESIAN_POINT('Ctrl Pts',(-0.749988983637343,-0.284097638645987,
-3.36155753444606));
#48724=CARTESIAN_POINT('Ctrl Pts',(-0.691448188391254,-0.406318036311524,
-3.35627169758742));
#48725=CARTESIAN_POINT('Ctrl Pts',(-0.607265030498785,-0.507124599436057,
-3.35098586072877));
#48726=CARTESIAN_POINT('Ctrl Pts',(-0.523081872606318,-0.607931162560587,
-3.34570002387012));
#48727=CARTESIAN_POINT('Ctrl Pts',(-0.413256352067474,-0.687323891144112,
-3.34041418701147));
#48728=CARTESIAN_POINT('Ctrl Pts',(-0.291137274043885,-0.735652950977678,
-3.33512835015283));
#48729=CARTESIAN_POINT('Ctrl Pts',(-0.169018196020292,-0.783982010811247,
-3.32984251329418));
#48730=CARTESIAN_POINT('Ctrl Pts',(-0.0346055605119571,-0.801247401894854,
-3.32455667643553));
#48731=CARTESIAN_POINT('Ctrl Pts',(0.0957633724903723,-0.785350592480289,
-3.31927083957688));
#48732=CARTESIAN_POINT('Ctrl Pts',(0.226132305492698,-0.769453783065725,
-3.31398500271823));
#48733=CARTESIAN_POINT('Ctrl Pts',(0.352457535989015,-0.720394773152992,
-3.30869916585959));
#48734=CARTESIAN_POINT('Ctrl Pts',(0.459384792216076,-0.644136467916903,
-3.30341332900094));
#48735=CARTESIAN_POINT('Ctrl Pts',(0.566312048443142,-0.56787816268081,
-3.29812749214229));
#48736=CARTESIAN_POINT('Ctrl Pts',(0.653841330400947,-0.46442056212136,
-3.29284165528365));
#48737=CARTESIAN_POINT('Ctrl Pts',(0.71133384188748,-0.346338478955874,
-3.287555818425));
#48738=CARTESIAN_POINT('Ctrl Pts',(0.768826353374009,-0.228256395790395,
-3.28226998156635));
#48739=CARTESIAN_POINT('Ctrl Pts',(0.79628209438927,-0.0955498300188732,
-3.2769841447077));
#48740=CARTESIAN_POINT('Ctrl Pts',(0.790363941324987,0.0356513235813738,
-3.27169830784905));
#48741=CARTESIAN_POINT('Ctrl Pts',(0.784445788260703,0.166852477181624,
-3.2664124709904));
#48742=CARTESIAN_POINT('Ctrl Pts',(0.745153741116876,0.296548218610608,
-3.26112663413176));
#48743=CARTESIAN_POINT('Ctrl Pts',(0.677263574041,0.408974605442786,-3.25584079727311));
#48744=CARTESIAN_POINT('Ctrl Pts',(0.609373406965123,0.521400992274967,
-3.25055496041446));
#48745=CARTESIAN_POINT('Ctrl Pts',(0.512885119957205,0.616558024510333,
-3.24526912355581));
#48746=CARTESIAN_POINT('Ctrl Pts',(0.399526436567544,0.682879786714698,
-3.23998328669717));
#48747=CARTESIAN_POINT('Ctrl Pts',(0.286167753177889,0.749201548919059,
-3.23469744983852));
#48748=CARTESIAN_POINT('Ctrl Pts',(0.15593867340649,0.786688041092416,-3.22941161297987));
#48749=CARTESIAN_POINT('Ctrl Pts',(0.0246679645901216,0.790782946289847,
-3.22412577612122));
#48750=CARTESIAN_POINT('Ctrl Pts',(-0.106602744226251,0.794877851487278,
-3.21883993926257));
#48751=CARTESIAN_POINT('Ctrl Pts',(-0.238915082087602,0.765581169708787,
-3.21355410240393));
#48752=CARTESIAN_POINT('Ctrl Pts',(-0.35618707087149,0.706453782751469,
-3.20826826554528));
#48753=CARTESIAN_POINT('Ctrl Pts',(-0.473459059655378,0.64732639579415,
-3.20298242868663));
#48754=CARTESIAN_POINT('Ctrl Pts',(-0.575690699361802,0.558368303658006,
-3.19769659182798));
#48755=CARTESIAN_POINT('Ctrl Pts',(-0.650456187380403,0.450391968088266,
-3.19241075496933));
#48756=CARTESIAN_POINT('Ctrl Pts',(-0.725221675399004,0.342415632518525,
-3.18712491811069));
#48757=CARTESIAN_POINT('Ctrl Pts',(-0.772521011729782,0.215421053515189,
-3.18183908125204));
#48758=CARTESIAN_POINT('Ctrl Pts',(-0.786605171721123,0.0848438591852945,
-3.17655324439339));
#48759=CARTESIAN_POINT('Ctrl Pts',(-0.789642795110382,0.05668141713378,
-3.1754132132035));
#48760=CARTESIAN_POINT('Ctrl Pts',(-0.791135368568485,0.0283523247683521,
-3.1742731820136));
#48761=CARTESIAN_POINT('Ctrl Pts',(-0.791106220557104,2.01772645531753E-5,
-3.1731331508237));
#48762=CARTESIAN_POINT('Origin',(0.,0.,-2.94));
#48763=CARTESIAN_POINT('',(-0.791107863766246,-2.00924285314041E-5,-2.9446668491763));
#48764=CARTESIAN_POINT('',(-0.791124187626007,-1.85461628832581E-5,-2.9731331508237));
#48765=CARTESIAN_POINT('',(-0.7911,-9.68818082805471E-17,-2.94));
#48766=CARTESIAN_POINT('Ctrl Pts',(-0.791107863766246,-2.00924285314041E-5,
-2.9446668491763));
#48767=CARTESIAN_POINT('Ctrl Pts',(-0.791001312710621,0.103530253044447,
-2.9488335410581));
#48768=CARTESIAN_POINT('Ctrl Pts',(-0.770561409006878,0.207121421232705,
-2.9530002329399));
#48769=CARTESIAN_POINT('Ctrl Pts',(-0.73094283724062,0.302768471603754,
-2.9571669248217));
#48770=CARTESIAN_POINT('Ctrl Pts',(-0.680682987731794,0.424105666340949,
-2.96245276168035));
#48771=CARTESIAN_POINT('Ctrl Pts',(-0.599558358653987,0.53265816484695,
-2.967738598539));
#48772=CARTESIAN_POINT('Ctrl Pts',(-0.497429289043663,0.61523189214487,
-2.97302443539765));
#48773=CARTESIAN_POINT('Ctrl Pts',(-0.395300219433336,0.697805619442793,
-2.9783102722563));
#48774=CARTESIAN_POINT('Ctrl Pts',(-0.272166709290493,0.754400575532634,
-2.98359610911494));
#48775=CARTESIAN_POINT('Ctrl Pts',(-0.142995090918413,0.778137894388827,
-2.98888194597359));
#48776=CARTESIAN_POINT('Ctrl Pts',(-0.013823472546338,0.801875213245019,
-2.99416778283224));
#48777=CARTESIAN_POINT('Ctrl Pts',(0.121386254054973,0.792754894867565,
-2.99945361969088));
#48778=CARTESIAN_POINT('Ctrl Pts',(0.246199946005947,0.751885473524598,
-3.00473945654953));
#48779=CARTESIAN_POINT('Ctrl Pts',(0.371013637956925,0.71101605218163,-3.01002529340818));
#48780=CARTESIAN_POINT('Ctrl Pts',(0.485431295257566,0.638397527873147,
-3.01531113026683));
#48781=CARTESIAN_POINT('Ctrl Pts',(0.575545958879919,0.542856360308726,
-3.02059696712548));
#48782=CARTESIAN_POINT('Ctrl Pts',(0.665660622502271,0.447315192744304,
-3.02588280398412));
#48783=CARTESIAN_POINT('Ctrl Pts',(0.731472292446335,0.328851381923943,
-3.03116864084277));
#48784=CARTESIAN_POINT('Ctrl Pts',(0.764981851975537,0.201863678899196,
-3.03645447770142));
#48785=CARTESIAN_POINT('Ctrl Pts',(0.79849141150474,0.0748759758744486,
-3.04174031456007));
#48786=CARTESIAN_POINT('Ctrl Pts',(0.799698860619082,-0.0606356193546861,
-3.04702615141872));
#48787=CARTESIAN_POINT('Ctrl Pts',(0.768457439231372,-0.188200273115115,
-3.05231198827736));
#48788=CARTESIAN_POINT('Ctrl Pts',(0.737216017843662,-0.315764926875544,
-3.05759782513601));
#48789=CARTESIAN_POINT('Ctrl Pts',(0.6735257259539,-0.435382639167268,-3.06288366199466));
#48790=CARTESIAN_POINT('Ctrl Pts',(0.585127836200294,-0.532514407330171,
-3.06816949885331));
#48791=CARTESIAN_POINT('Ctrl Pts',(0.496729946446687,-0.629646175493074,
-3.07345533571196));
#48792=CARTESIAN_POINT('Ctrl Pts',(0.383624458829236,-0.704291999527155,
-3.0787411725706));
#48793=CARTESIAN_POINT('Ctrl Pts',(0.259558843967787,-0.747379010428274,
-3.08402700942925));
#48794=CARTESIAN_POINT('Ctrl Pts',(0.135493229106338,-0.790466021329393,
-3.0893128462879));
#48795=CARTESIAN_POINT('Ctrl Pts',(0.00046748700088986,-0.801994219097549,
-3.09459868314655));
#48796=CARTESIAN_POINT('Ctrl Pts',(-0.129106601968846,-0.780562402398873,
-3.09988452000519));
#48797=CARTESIAN_POINT('Ctrl Pts',(-0.258680690938578,-0.759130585700196,
-3.10517035686384));
#48798=CARTESIAN_POINT('Ctrl Pts',(-0.382803126772598,-0.704738754534689,
-3.11045619372249));
#48799=CARTESIAN_POINT('Ctrl Pts',(-0.486387377633802,-0.623997994859883,
-3.11574203058114));
#48800=CARTESIAN_POINT('Ctrl Pts',(-0.589971628495012,-0.543257235185072,
-3.12102786743978));
#48801=CARTESIAN_POINT('Ctrl Pts',(-0.673017694383403,-0.436167547000958,
-3.12631370429843));
#48802=CARTESIAN_POINT('Ctrl Pts',(-0.725431694135968,-0.315745207174489,
-3.13159954115708));
#48803=CARTESIAN_POINT('Ctrl Pts',(-0.768623207457408,-0.216511736739724,
-3.13595531049682));
#48804=CARTESIAN_POINT('Ctrl Pts',(-0.791013993106437,-0.10822471912554,
-3.14031107983656));
#48805=CARTESIAN_POINT('Ctrl Pts',(-0.791122594563005,1.8755956602709E-5,
-3.1446668491763));
#48806=CARTESIAN_POINT('Ctrl Pts',(-0.791106220557104,2.01772645531753E-5,
-3.1731331508237));
#48807=CARTESIAN_POINT('Ctrl Pts',(-0.791000221710857,-0.10301172113433,
-3.16898734515495));
#48808=CARTESIAN_POINT('Ctrl Pts',(-0.770769978441601,-0.206084022690134,
-3.1648415394862));
#48809=CARTESIAN_POINT('Ctrl Pts',(-0.731537412905569,-0.301329039654824,
-3.16069573381745));
#48810=CARTESIAN_POINT('Ctrl Pts',(-0.681516510446771,-0.422764934508594,
-3.1554098969588));
#48811=CARTESIAN_POINT('Ctrl Pts',(-0.600605721877271,-0.531476914559684,
-3.15012406010015));
#48812=CARTESIAN_POINT('Ctrl Pts',(-0.498639394867715,-0.614251520556384,
-3.14483822324151));
#48813=CARTESIAN_POINT('Ctrl Pts',(-0.396673067858159,-0.697026126553084,
-3.13955238638286));
#48814=CARTESIAN_POINT('Ctrl Pts',(-0.273651202408545,-0.753863358495396,
-3.13426654952421));
#48815=CARTESIAN_POINT('Ctrl Pts',(-0.144526560904618,-0.777854902801901,
-3.12898071266556));
#48816=CARTESIAN_POINT('Ctrl Pts',(-0.0154019194006878,-0.801846447108407,
-3.12369487580691));
#48817=CARTESIAN_POINT('Ctrl Pts',(0.119825498157559,-0.792992303779106,
-3.11840903894826));
#48818=CARTESIAN_POINT('Ctrl Pts',(0.244719398633153,-0.752368654684988,
-3.11312320208962));
#48819=CARTESIAN_POINT('Ctrl Pts',(0.36961329910874,-0.711745005590873,
-3.10783736523097));
#48820=CARTESIAN_POINT('Ctrl Pts',(0.484173682501678,-0.639351850731945,
-3.10255152837232));
#48821=CARTESIAN_POINT('Ctrl Pts',(0.574476242060206,-0.543988257160257,
-3.09726569151368));
#48822=CARTESIAN_POINT('Ctrl Pts',(0.664778801618738,-0.448624663588567,
-3.09197985465503));
#48823=CARTESIAN_POINT('Ctrl Pts',(0.73082353734286,-0.330290631304114,
-3.08669401779638));
#48824=CARTESIAN_POINT('Ctrl Pts',(0.764583004383618,-0.203369137352724,
-3.08140818093773));
#48825=CARTESIAN_POINT('Ctrl Pts',(0.798342471424376,-0.0764476434013388,
-3.07612234407908));
#48826=CARTESIAN_POINT('Ctrl Pts',(0.799816669781773,0.0590613122169849,
-3.07083650722044));
#48827=CARTESIAN_POINT('Ctrl Pts',(0.768826417180635,0.186687216662146,
-3.06555067036179));
#48828=CARTESIAN_POINT('Ctrl Pts',(0.737836164579496,0.31431312110731,-3.06026483350314));
#48829=CARTESIAN_POINT('Ctrl Pts',(0.674381461019825,0.434055974379303,
-3.05497899664449));
#48830=CARTESIAN_POINT('Ctrl Pts',(0.586174944422666,0.531361563486629,
-3.04969315978585));
#48831=CARTESIAN_POINT('Ctrl Pts',(0.497968427825508,0.628667152593956,
-3.0444073229272));
#48832=CARTESIAN_POINT('Ctrl Pts',(0.385010098190864,0.703535477536607,
-3.03912148606855));
#48833=CARTESIAN_POINT('Ctrl Pts',(0.261029539738131,0.746866625311354,
-3.0338356492099));
#48834=CARTESIAN_POINT('Ctrl Pts',(0.137048981285398,0.790197773086102,
-3.02854981235125));
#48835=CARTESIAN_POINT('Ctrl Pts',(0.00204619401457248,0.801991743692947,
-3.0232639754926));
#48836=CARTESIAN_POINT('Ctrl Pts',(-0.127569831753022,0.780815032287658,
-3.01797813863396));
#48837=CARTESIAN_POINT('Ctrl Pts',(-0.257185857520617,0.759638320882368,
-3.01269230177531));
#48838=CARTESIAN_POINT('Ctrl Pts',(-0.381415121784982,0.705490927464944,
-3.00740646491666));
#48839=CARTESIAN_POINT('Ctrl Pts',(-0.485158108186877,0.624954227668236,
-3.00212062805802));
#48840=CARTESIAN_POINT('Ctrl Pts',(-0.588901094588771,0.544417527871529,
-2.99683479119937));
#48841=CARTESIAN_POINT('Ctrl Pts',(-0.672157803128195,0.437491521695538,
-2.99154895434072));
#48842=CARTESIAN_POINT('Ctrl Pts',(-0.724808749961695,0.317172591184729,
-2.98626311748207));
#48843=CARTESIAN_POINT('Ctrl Pts',(-0.768403560959603,0.217548912019442,
-2.98188646192928));
#48844=CARTESIAN_POINT('Ctrl Pts',(-0.791015717938958,0.108743331083034,
-2.97750980637649));
#48845=CARTESIAN_POINT('Ctrl Pts',(-0.791124187626007,-1.85461628832581E-5,
-2.9731331508237));
#48846=CARTESIAN_POINT('Origin',(0.,0.,-2.94));
#48847=CARTESIAN_POINT('',(-0.79104321788868,1.14421256602881E-5,-2.74466684917629));
#48848=CARTESIAN_POINT('',(-0.791036517039322,7.12926283942606E-6,-2.7731331508237));
#48849=CARTESIAN_POINT('',(-0.7911,-9.68818082805471E-17,-2.94));
#48850=CARTESIAN_POINT('Ctrl Pts',(-0.79104321788868,1.14421256602881E-5,
-2.74466684917629));
#48851=CARTESIAN_POINT('Ctrl Pts',(-0.791070225503421,0.0526472450371811,
-2.74678432856234));
#48852=CARTESIAN_POINT('Ctrl Pts',(-0.785894891195464,0.105277808041528,
-2.74890180794839));
#48853=CARTESIAN_POINT('Ctrl Pts',(-0.775464798820223,0.156845543453911,
-2.75101928733444));
#48854=CARTESIAN_POINT('Ctrl Pts',(-0.749428291886831,0.28557342546107,
-2.75630512419308));
#48855=CARTESIAN_POINT('Ctrl Pts',(-0.690647021806916,0.407678350270431,
-2.76159096105174));
#48856=CARTESIAN_POINT('Ctrl Pts',(-0.606265591379539,0.508319005566248,
-2.76687679791038));
#48857=CARTESIAN_POINT('Ctrl Pts',(-0.52188416095216,0.608959660862067,
-2.77216263476903));
#48858=CARTESIAN_POINT('Ctrl Pts',(-0.411902570177317,0.688136046644342,
-2.77744847162768));
#48859=CARTESIAN_POINT('Ctrl Pts',(-0.289688593861968,0.736224624212554,
-2.78273430848632));
#48860=CARTESIAN_POINT('Ctrl Pts',(-0.16747461754662,0.784313201780766,
-2.78802014534497));
#48861=CARTESIAN_POINT('Ctrl Pts',(-0.0330282556907639,0.801313971134916,
-2.79330598220362));
#48862=CARTESIAN_POINT('Ctrl Pts',(0.0973091324268148,0.785160564124932,
-2.79859181906227));
#48863=CARTESIAN_POINT('Ctrl Pts',(0.227646520544393,0.769007157114948,
-2.80387765592092));
#48864=CARTESIAN_POINT('Ctrl Pts',(0.353874934923697,0.71969957374083,-2.80916349277956));
#48865=CARTESIAN_POINT('Ctrl Pts',(0.460651871371306,0.643230932179692,
-2.81444932963821));
#48866=CARTESIAN_POINT('Ctrl Pts',(0.567428807818914,0.566762290618553,
-2.81973516649686));
#48867=CARTESIAN_POINT('Ctrl Pts',(0.654754266334829,0.463132590870392,
-2.82502100335551));
#48868=CARTESIAN_POINT('Ctrl Pts',(0.712014224552845,0.344937563546001,
-2.83030684021416));
#48869=CARTESIAN_POINT('Ctrl Pts',(0.769274182770862,0.226742536221606,
-2.8355926770728));
#48870=CARTESIAN_POINT('Ctrl Pts',(0.796468640690977,0.0939821813209887,
-2.84087851393145));
#48871=CARTESIAN_POINT('Ctrl Pts',(0.790292232506861,-0.0372070685483761,
-2.8461643507901));
#48872=CARTESIAN_POINT('Ctrl Pts',(0.784115824322744,-0.168396318417734,
-2.85145018764875));
#48873=CARTESIAN_POINT('Ctrl Pts',(0.744568550034392,-0.298014463255841,
-2.85673602450739));
#48874=CARTESIAN_POINT('Ctrl Pts',(0.676457205517293,-0.410306992158768,
-2.86202186136604));
#48875=CARTESIAN_POINT('Ctrl Pts',(0.608345861000192,-0.522599521061702,
-2.86730769822469));
#48876=CARTESIAN_POINT('Ctrl Pts',(0.511670446254346,-0.617566434029459,
-2.87259353508334));
#48877=CARTESIAN_POINT('Ctrl Pts',(0.398181429377058,-0.683664923782026,
-2.87787937194199));
#48878=CARTESIAN_POINT('Ctrl Pts',(0.28469241249978,-0.749763413534587,
-2.88316520880063));
#48879=CARTESIAN_POINT('Ctrl Pts',(0.154389793491068,-0.786993480071955,
-2.88845104565928));
#48880=CARTESIAN_POINT('Ctrl Pts',(0.0231112780559711,-0.790829973848526,
-2.89373688251793));
#48881=CARTESIAN_POINT('Ctrl Pts',(-0.108167237379137,-0.794666467625097,
-2.89902271937658));
#48882=CARTESIAN_POINT('Ctrl Pts',(-0.240421649240631,-0.765109388640866,
-2.90430855623523));
#48883=CARTESIAN_POINT('Ctrl Pts',(-0.35757702005456,-0.705751268818939,
-2.90959439309387));
#48884=CARTESIAN_POINT('Ctrl Pts',(-0.474732390868486,-0.646393148997013,
-2.91488022995252));
#48885=CARTESIAN_POINT('Ctrl Pts',(-0.576788720634849,-0.557233988337392,
-2.92016606681117));
#48886=CARTESIAN_POINT('Ctrl Pts',(-0.65134151488935,-0.449110687572994,
-2.92545190366982));
#48887=CARTESIAN_POINT('Ctrl Pts',(-0.725894309143851,-0.340987386808595,
-2.93073774052846));
#48888=CARTESIAN_POINT('Ctrl Pts',(-0.772943567886491,-0.213899945939417,
-2.93602357738711));
#48889=CARTESIAN_POINT('Ctrl Pts',(-0.786770662287891,-0.0832952800206322,
-2.94130941424576));
#48890=CARTESIAN_POINT('Ctrl Pts',(-0.789698206905234,-0.0556429782708374,
-2.94242855922261));
#48891=CARTESIAN_POINT('Ctrl Pts',(-0.791136482651938,-0.0278330078717755,
-2.94354770419945));
#48892=CARTESIAN_POINT('Ctrl Pts',(-0.791107863766246,-2.00924285314041E-5,
-2.9446668491763));
#48893=CARTESIAN_POINT('Ctrl Pts',(-0.791124187626007,-1.85461628832581E-5,
-2.9731331508237));
#48894=CARTESIAN_POINT('Ctrl Pts',(-0.79114672049626,-0.0226121143313561,
-2.97222396951784));
#48895=CARTESIAN_POINT('Ctrl Pts',(-0.790198139977264,-0.045203796531612,
-2.97131478821199));
#48896=CARTESIAN_POINT('Ctrl Pts',(-0.788264810819136,-0.067710890144367,
-2.97040560690613));
#48897=CARTESIAN_POINT('Ctrl Pts',(-0.777024739715503,-0.19856358611703,
-2.96511977004748));
#48898=CARTESIAN_POINT('Ctrl Pts',(-0.732499412380662,-0.326557123216728,
-2.95983393318883));
#48899=CARTESIAN_POINT('Ctrl Pts',(-0.660100684970037,-0.436134454408224,
-2.95454809633018));
#48900=CARTESIAN_POINT('Ctrl Pts',(-0.587701957559412,-0.54571178559972,
-2.94926225947154));
#48901=CARTESIAN_POINT('Ctrl Pts',(-0.487429830073004,-0.636872910883013,
-2.94397642261289));
#48902=CARTESIAN_POINT('Ctrl Pts',(-0.371471935097405,-0.69853759959995,
-2.93869058575424));
#48903=CARTESIAN_POINT('Ctrl Pts',(-0.255514040121806,-0.760202288316887,
-2.93340474889559));
#48904=CARTESIAN_POINT('Ctrl Pts',(-0.123870377657018,-0.792370540467468,
-2.92811891203694));
#48905=CARTESIAN_POINT('Ctrl Pts',(0.00745834870471288,-0.791132447605627,
-2.9228330751783));
#48906=CARTESIAN_POINT('Ctrl Pts',(0.138787075066443,-0.789894354743785,
-2.91754723831965));
#48907=CARTESIAN_POINT('Ctrl Pts',(0.269800865325114,-0.755249916869522,
-2.912261401461));
#48908=CARTESIAN_POINT('Ctrl Pts',(0.384575574062887,-0.691410011826609,
-2.90697556460235));
#48909=CARTESIAN_POINT('Ctrl Pts',(0.499350282800658,-0.627570106783698,
-2.90168972774371));
#48910=CARTESIAN_POINT('Ctrl Pts',(0.597885910017537,-0.534534734572132,
-2.89640389088506));
#48911=CARTESIAN_POINT('Ctrl Pts',(0.668205887036723,-0.423611932255616,
-2.89111805402641));
#48912=CARTESIAN_POINT('Ctrl Pts',(0.738525864055913,-0.312689129939094,
-2.88583221716776));
#48913=CARTESIAN_POINT('Ctrl Pts',(0.780630190877411,-0.183878897517624,
-2.88054638030912));
#48914=CARTESIAN_POINT('Ctrl Pts',(0.789401273225829,-0.0528375477223508,
-2.87526054345047));
#48915=CARTESIAN_POINT('Ctrl Pts',(0.798172355574245,0.078203802072915,
-2.86997470659182));
#48916=CARTESIAN_POINT('Ctrl Pts',(0.773610193449577,0.211476269241981,
-2.86468886973317));
#48917=CARTESIAN_POINT('Ctrl Pts',(0.718700208773271,0.330781176201317,
-2.85940303287452));
#48918=CARTESIAN_POINT('Ctrl Pts',(0.663790224096964,0.450086083160657,
-2.85411719601588));
#48919=CARTESIAN_POINT('Ctrl Pts',(0.578532416869019,0.555423429910273,
-2.84883135915723));
#48920=CARTESIAN_POINT('Ctrl Pts',(0.473289495607546,0.633989928916403,
-2.84354552229858));
#48921=CARTESIAN_POINT('Ctrl Pts',(0.368046574346073,0.712556427922533,
-2.83825968543993));
#48922=CARTESIAN_POINT('Ctrl Pts',(0.242818539051075,0.764352079185176,
-2.83297384858128));
#48923=CARTESIAN_POINT('Ctrl Pts',(0.112826302272981,0.783081350905049,
-2.82768801172263));
#48924=CARTESIAN_POINT('Ctrl Pts',(-0.0171659345051129,0.801810622624923,
-2.82240217486399));
#48925=CARTESIAN_POINT('Ctrl Pts',(-0.1519223727663,0.787473514802027,-2.81711633800534));
#48926=CARTESIAN_POINT('Ctrl Pts',(-0.275063964819311,0.7418126393354,-2.81183050114669));
#48927=CARTESIAN_POINT('Ctrl Pts',(-0.398205556872314,0.696151763868776,
-2.80654466428805));
#48928=CARTESIAN_POINT('Ctrl Pts',(-0.50973230271714,0.619167120758426,
-2.8012588274294));
#48929=CARTESIAN_POINT('Ctrl Pts',(-0.596088620797797,0.520215852099155,
-2.79597299057075));
#48930=CARTESIAN_POINT('Ctrl Pts',(-0.682444938878462,0.421264583439876,
-2.7906871537121));
#48931=CARTESIAN_POINT('Ctrl Pts',(-0.743630829194953,0.300346689231674,
-2.78540131685345));
#48932=CARTESIAN_POINT('Ctrl Pts',(-0.772209418018207,0.172159203482865,
-2.78011547999481));
#48933=CARTESIAN_POINT('Ctrl Pts',(-0.784793052344291,0.115716093019316,
-2.77778803693777));
#48934=CARTESIAN_POINT('Ctrl Pts',(-0.791054817880501,0.0578635619115849,
-2.77546059388074));
#48935=CARTESIAN_POINT('Ctrl Pts',(-0.791036517039322,7.12926283942606E-6,
-2.7731331508237));
#48936=CARTESIAN_POINT('Origin',(0.,0.,-2.94));
#48937=CARTESIAN_POINT('',(-0.791167260441282,1.79117177186508E-6,-2.5446668491763));
#48938=CARTESIAN_POINT('',(-0.791162320258143,7.12643492048928E-6,-2.5731331508237));
#48939=CARTESIAN_POINT('',(-0.7911,-9.68818082805471E-17,-2.94));
#48940=CARTESIAN_POINT('Ctrl Pts',(-0.791167260441282,1.79117177186508E-6,
-2.5446668491763));
#48941=CARTESIAN_POINT('Ctrl Pts',(-0.791167483212997,0.00169798683385348,
-2.54473511606659));
#48942=CARTESIAN_POINT('Ctrl Pts',(-0.791162142242542,0.00339418108704642,
-2.54480338295688));
#48943=CARTESIAN_POINT('Ctrl Pts',(-0.791151229004,0.00509033948775599,
-2.54487164984718));
#48944=CARTESIAN_POINT('Ctrl Pts',(-0.790306227887311,0.136422183579185,
-2.55015748670582));
#48945=CARTESIAN_POINT('Ctrl Pts',(-0.756054088695197,0.267539083083683,
-2.55544332356447));
#48946=CARTESIAN_POINT('Ctrl Pts',(-0.69255800710569,0.382504360111667,
-2.56072916042312));
#48947=CARTESIAN_POINT('Ctrl Pts',(-0.629061925516182,0.497469637139652,
-2.56601499728176));
#48948=CARTESIAN_POINT('Ctrl Pts',(-0.53632190152928,0.596283291691123,
-2.57130083414041));
#48949=CARTESIAN_POINT('Ctrl Pts',(-0.425610073941255,0.666934962099274,
-2.57658667099906));
#48950=CARTESIAN_POINT('Ctrl Pts',(-0.31489824635323,0.737586632507426,
-2.58187250785771));
#48951=CARTESIAN_POINT('Ctrl Pts',(-0.186214615164082,0.780076318772257,
-2.58715834471636));
#48952=CARTESIAN_POINT('Ctrl Pts',(-0.0552001052864145,0.789239587886346,
-2.592444181575));
#48953=CARTESIAN_POINT('Ctrl Pts',(0.0758144045912454,0.798402857000435,
-2.59773001843365));
#48954=CARTESIAN_POINT('Ctrl Pts',(0.209159793157424,0.774239708963784,
-2.6030158552923));
#48955=CARTESIAN_POINT('Ctrl Pts',(0.328628519556054,0.719687067304282,
-2.60830169215095));
#48956=CARTESIAN_POINT('Ctrl Pts',(0.448097245954693,0.665134425644775,
-2.6135875290096));
#48957=CARTESIAN_POINT('Ctrl Pts',(0.553689310185781,0.580192290362409,
-2.61887336586824));
#48958=CARTESIAN_POINT('Ctrl Pts',(0.632570464934848,0.475185001449699,
-2.62415920272689));
#48959=CARTESIAN_POINT('Ctrl Pts',(0.711451619683911,0.370177712536995,
-2.62944503958554));
#48960=CARTESIAN_POINT('Ctrl Pts',(0.763621864950956,0.245105269993949,
-2.63473087644419));
#48961=CARTESIAN_POINT('Ctrl Pts',(0.782740138696053,0.115169674761737,
-2.64001671330283));
#48962=CARTESIAN_POINT('Ctrl Pts',(0.801858412441151,-0.0147659204704824,
-2.64530255016148));
#48963=CARTESIAN_POINT('Ctrl Pts',(0.787924714664298,-0.149564668391867,
-2.65058838702013));
#48964=CARTESIAN_POINT('Ctrl Pts',(0.742632624561765,-0.272842378759507,
-2.65587422387878));
#48965=CARTESIAN_POINT('Ctrl Pts',(0.697340534459234,-0.396120089127139,
-2.66116006073743));
#48966=CARTESIAN_POINT('Ctrl Pts',(0.620690052031027,-0.507876761941027,
-2.66644589759607));
#48967=CARTESIAN_POINT('Ctrl Pts',(0.52199770362238,-0.594528869041363,
-2.67173173445472));
#48968=CARTESIAN_POINT('Ctrl Pts',(0.423305355213725,-0.681180976141705,
-2.67701757131337));
#48969=CARTESIAN_POINT('Ctrl Pts',(0.302571140824627,-0.74272851752849,
-2.68230340817202));
#48970=CARTESIAN_POINT('Ctrl Pts',(0.17446976899565,-0.771690662388269,
-2.68758924503066));
#48971=CARTESIAN_POINT('Ctrl Pts',(0.0463683971666843,-0.800652807248045,
-2.69287508188931));
#48972=CARTESIAN_POINT('Ctrl Pts',(-0.0891001321021591,-0.797029555580821,
-2.69816091874796));
#48973=CARTESIAN_POINT('Ctrl Pts',(-0.215470219614348,-0.761261297564762,
-2.70344675560661));
#48974=CARTESIAN_POINT('Ctrl Pts',(-0.341840307126537,-0.725493039548704,
-2.70873259246526));
#48975=CARTESIAN_POINT('Ctrl Pts',(-0.459111952882072,-0.657579775183812,
-2.7140184293239));
#48976=CARTESIAN_POINT('Ctrl Pts',(-0.553031308208128,-0.565776060692079,
-2.71930426618255));
#48977=CARTESIAN_POINT('Ctrl Pts',(-0.646950663534187,-0.473972346200343,
-2.7245901030412));
#48978=CARTESIAN_POINT('Ctrl Pts',(-0.717517728430766,-0.358278181581765,
-2.72987593989985));
#48979=CARTESIAN_POINT('Ctrl Pts',(-0.756155388985624,-0.232755679669995,
-2.7351617767585));
#48980=CARTESIAN_POINT('Ctrl Pts',(-0.779314999056162,-0.157516854192255,
-2.7383301342311));
#48981=CARTESIAN_POINT('Ctrl Pts',(-0.791002806738258,-0.0787468402830678,
-2.7414984917037));
#48982=CARTESIAN_POINT('Ctrl Pts',(-0.79104321788868,1.14421256602881E-5,
-2.74466684917629));
#48983=CARTESIAN_POINT('Ctrl Pts',(-0.791036517039322,7.12926283942606E-6,
-2.7731331508237));
#48984=CARTESIAN_POINT('Ctrl Pts',(-0.791013254990033,-0.0735337082730062,
-2.77017475702209));
#48985=CARTESIAN_POINT('Ctrl Pts',(-0.780843450574848,-0.14708084942872,
-2.76721636322048));
#48986=CARTESIAN_POINT('Ctrl Pts',(-0.760612952173891,-0.217747821126159,
-2.76425796941886));
#48987=CARTESIAN_POINT('Ctrl Pts',(-0.724466610176304,-0.34401028269698,
-2.75897213256022));
#48988=CARTESIAN_POINT('Ctrl Pts',(-0.65620263885111,-0.461078128549208,
-2.75368629570157));
#48989=CARTESIAN_POINT('Ctrl Pts',(-0.564118221296634,-0.554722280984812,
-2.74840045884292));
#48990=CARTESIAN_POINT('Ctrl Pts',(-0.472033803742163,-0.64836643342041,
-2.74311462198427));
#48991=CARTESIAN_POINT('Ctrl Pts',(-0.356128939958412,-0.718586892439387,
-2.73782878512563));
#48992=CARTESIAN_POINT('Ctrl Pts',(-0.230491352328523,-0.75684867253741,
-2.73254294826698));
#48993=CARTESIAN_POINT('Ctrl Pts',(-0.104853764698629,-0.795110452635434,
-2.72725711140833));
#48994=CARTESIAN_POINT('Ctrl Pts',(0.0305165467774051,-0.801413553812501,
-2.72197127454968));
#48995=CARTESIAN_POINT('Ctrl Pts',(0.15916592084036,-0.774991862062378,
-2.71668543769103));
#48996=CARTESIAN_POINT('Ctrl Pts',(0.287815294903315,-0.748570170312255,
-2.71139960083238));
#48997=CARTESIAN_POINT('Ctrl Pts',(0.409743731553193,-0.68942368563494,
-2.70611376397374));
#48998=CARTESIAN_POINT('Ctrl Pts',(0.510131369827653,-0.604741401044805,
-2.70082792711509));
#48999=CARTESIAN_POINT('Ctrl Pts',(0.610519008102113,-0.520059116454669,
-2.69554209025644));
#49000=CARTESIAN_POINT('Ctrl Pts',(0.689365848001159,-0.40984103195171,
-2.69025625339779));
#49001=CARTESIAN_POINT('Ctrl Pts',(0.737088405665489,-0.287483667107157,
-2.68497041653915));
#49002=CARTESIAN_POINT('Ctrl Pts',(0.784810963329821,-0.165126302262599,
-2.6796845796805));
#49003=CARTESIAN_POINT('Ctrl Pts',(0.801409238759436,-0.0306296570764548,
-2.67439874282185));
#49004=CARTESIAN_POINT('Ctrl Pts',(0.784865785156526,0.0996587974566231,
-2.6691129059632));
#49005=CARTESIAN_POINT('Ctrl Pts',(0.768322331553618,0.229947251989694,
-2.66382706910455));
#49006=CARTESIAN_POINT('Ctrl Pts',(0.718637148918179,0.3560275158697,-2.65854123224591));
#49007=CARTESIAN_POINT('Ctrl Pts',(0.641849250943637,0.462575091939637,
-2.65325539538726));
#49008=CARTESIAN_POINT('Ctrl Pts',(0.56506135296909,0.56912266800958,-2.64796955852861));
#49009=CARTESIAN_POINT('Ctrl Pts',(0.461170739655441,0.656137556269456,
-2.64268372166996));
#49010=CARTESIAN_POINT('Ctrl Pts',(0.342804854500712,0.713043482790928,
-2.63739788481132));
#49011=CARTESIAN_POINT('Ctrl Pts',(0.224438969345987,0.769949409312398,
-2.63211204795267));
#49012=CARTESIAN_POINT('Ctrl Pts',(0.0915978123501881,0.796746374095458,
-2.62682621109402));
#49013=CARTESIAN_POINT('Ctrl Pts',(-0.0395723627427169,0.790177324862483,
-2.62154037423537));
#49014=CARTESIAN_POINT('Ctrl Pts',(-0.170742537835622,0.783608275629508,
-2.61625453737672));
#49015=CARTESIAN_POINT('Ctrl Pts',(-0.300241731025636,0.743673212380498,
-2.61096870051808));
#49016=CARTESIAN_POINT('Ctrl Pts',(-0.412329889454358,0.675226065020025,
-2.60568286365943));
#49017=CARTESIAN_POINT('Ctrl Pts',(-0.524418047883078,0.606778917659555,
-2.60039702680078));
#49018=CARTESIAN_POINT('Ctrl Pts',(-0.619095171550508,0.509819686187622,
-2.59511118994213));
#49019=CARTESIAN_POINT('Ctrl Pts',(-0.684853675781432,0.39613333536643,
-2.58982535308349));
#49020=CARTESIAN_POINT('Ctrl Pts',(-0.75061218001236,0.282446984545231,
-2.58453951622484));
#49021=CARTESIAN_POINT('Ctrl Pts',(-0.787452064806777,0.152033514374769,
-2.57925367936619));
#49022=CARTESIAN_POINT('Ctrl Pts',(-0.79089560548025,0.0207441040273998,
-2.57396784250754));
#49023=CARTESIAN_POINT('Ctrl Pts',(-0.791076863108889,0.013833424165714,
-2.57368961194626));
#49024=CARTESIAN_POINT('Ctrl Pts',(-0.791165591053067,0.00692031737765905,
-2.57341138138498));
#49025=CARTESIAN_POINT('Ctrl Pts',(-0.791162320258143,7.12643492048928E-6,
-2.5731331508237));
#49026=CARTESIAN_POINT('Origin',(0.,0.,-2.94));
#49027=CARTESIAN_POINT('',(-0.791049211918833,-1.3923086196882E-5,-2.3446668491763));
#49028=CARTESIAN_POINT('',(-0.791060671368687,-1.7079190050548E-5,-2.3731331508237));
#49029=CARTESIAN_POINT('',(-0.7911,-9.68818082805471E-17,-2.94));
#49030=CARTESIAN_POINT('Ctrl Pts',(-0.791049211918833,-1.3923086196882E-5,
-2.3446668491763));
#49031=CARTESIAN_POINT('Ctrl Pts',(-0.790997411345824,0.0821365012599493,
-2.34797174042948));
#49032=CARTESIAN_POINT('Ctrl Pts',(-0.778263259369705,0.164302615906683,
-2.35127663168267));
#49033=CARTESIAN_POINT('Ctrl Pts',(-0.753097766892199,0.242466352743269,
-2.35458152293585));
#49034=CARTESIAN_POINT('Ctrl Pts',(-0.712848125523398,0.367481286527303,
-2.3598673597945));
#49035=CARTESIAN_POINT('Ctrl Pts',(-0.640798190910364,0.48225784030536,
-2.36515319665315));
#49036=CARTESIAN_POINT('Ctrl Pts',(-0.545705313205766,0.572845432773656,
-2.3704390335118));
#49037=CARTESIAN_POINT('Ctrl Pts',(-0.450612435501175,0.663433025241947,
-2.37572487037045));
#49038=CARTESIAN_POINT('Ctrl Pts',(-0.332476614705023,0.729831656400481,
-2.38101070722909));
#49039=CARTESIAN_POINT('Ctrl Pts',(-0.205656736135409,0.763970866979082,
-2.38629654408774));
#49040=CARTESIAN_POINT('Ctrl Pts',(-0.0788368575657881,0.798110077557686,
-2.39158238094639));
#49041=CARTESIAN_POINT('Ctrl Pts',(0.0566670787772957,0.799989867556354,
-2.39686821780504));
#49042=CARTESIAN_POINT('Ctrl Pts',(0.184385170124397,0.769381756833913,
-2.40215405466368));
#49043=CARTESIAN_POINT('Ctrl Pts',(0.312103261471486,0.738773646111475,
-2.40743989152233));
#49044=CARTESIAN_POINT('Ctrl Pts',(0.432035507822595,0.675677634667934,
-2.41272572838098));
#49045=CARTESIAN_POINT('Ctrl Pts',(0.529604676297028,0.587762762987721,
-2.41801156523963));
#49046=CARTESIAN_POINT('Ctrl Pts',(0.627173844771468,0.499847891307504,
-2.42329740209827));
#49047=CARTESIAN_POINT('Ctrl Pts',(0.70237993536923,0.387114159390612,-2.42858323895692));
#49048=CARTESIAN_POINT('Ctrl Pts',(0.746081981169035,0.263263852599493,
-2.43386907581557));
#49049=CARTESIAN_POINT('Ctrl Pts',(0.789784026968842,0.139413545808374,
-2.43915491267422));
#49050=CARTESIAN_POINT('Ctrl Pts',(0.801982027970691,0.00444666414302769,
-2.44444074953287));
#49051=CARTESIAN_POINT('Ctrl Pts',(0.781193371226918,-0.125232166242399,
-2.44972658639151));
#49052=CARTESIAN_POINT('Ctrl Pts',(0.760404714483145,-0.254910996627825,
-2.45501242325016));
#49053=CARTESIAN_POINT('Ctrl Pts',(0.706629399993748,-0.379301775733332,
-2.46029826010881));
#49054=CARTESIAN_POINT('Ctrl Pts',(0.626403578847316,-0.483285355786739,
-2.46558409696746));
#49055=CARTESIAN_POINT('Ctrl Pts',(0.546177757700884,-0.587268935840146,
-2.4708699338261));
#49056=CARTESIAN_POINT('Ctrl Pts',(0.439501429897416,-0.670845316841453,
-2.47615577068475));
#49057=CARTESIAN_POINT('Ctrl Pts',(0.31934063018203,-0.723856160176581,
-2.4814416075434));
#49058=CARTESIAN_POINT('Ctrl Pts',(0.199179830466644,-0.776867003511709,
-2.48672744440205));
#49059=CARTESIAN_POINT('Ctrl Pts',(0.0655345588393392,-0.799312309180659,
-2.4920132812607));
#49060=CARTESIAN_POINT('Ctrl Pts',(-0.0653511943871243,-0.788463949780088,
-2.49729911811934));
#49061=CARTESIAN_POINT('Ctrl Pts',(-0.196236947613588,-0.777615590379518,
-2.50258495497799));
#49062=CARTESIAN_POINT('Ctrl Pts',(-0.32436318243921,-0.733473565909427,
-2.50787079183664));
#49063=CARTESIAN_POINT('Ctrl Pts',(-0.434156723008419,-0.661403143761225,
-2.51315662869529));
#49064=CARTESIAN_POINT('Ctrl Pts',(-0.543950263577628,-0.589332721613023,
-2.51844246555394));
#49065=CARTESIAN_POINT('Ctrl Pts',(-0.635411109890424,-0.489333901786708,
-2.52372830241258));
#49066=CARTESIAN_POINT('Ctrl Pts',(-0.697422601526189,-0.373561097534371,
-2.52901413927123));
#49067=CARTESIAN_POINT('Ctrl Pts',(-0.758633211142775,-0.25928350577878,
-2.53423170923958));
#49068=CARTESIAN_POINT('Ctrl Pts',(-0.79115023422254,-0.129636742368248,
-2.53944927920794));
#49069=CARTESIAN_POINT('Ctrl Pts',(-0.791167260441282,1.79117177186508E-6,
-2.5446668491763));
#49070=CARTESIAN_POINT('Ctrl Pts',(-0.791162320258143,7.12643492048928E-6,
-2.5731331508237));
#49071=CARTESIAN_POINT('Ctrl Pts',(-0.791103452342327,-0.124416798601764,
-2.56812554452633));
#49072=CARTESIAN_POINT('Ctrl Pts',(-0.761243465869951,-0.248867983834946,
-2.56311793822897));
#49073=CARTESIAN_POINT('Ctrl Pts',(-0.704677825615191,-0.359687835082198,
-2.5581103319316));
#49074=CARTESIAN_POINT('Ctrl Pts',(-0.644969308524131,-0.476665013320157,
-2.55282449507295));
#49075=CARTESIAN_POINT('Ctrl Pts',(-0.555505077789481,-0.578454019271802,
-2.5475386582143));
#49076=CARTESIAN_POINT('Ctrl Pts',(-0.447159114059393,-0.65268285049746,
-2.54225282135565));
#49077=CARTESIAN_POINT('Ctrl Pts',(-0.338813150329307,-0.726911681723116,
-2.53696698449701));
#49078=CARTESIAN_POINT('Ctrl Pts',(-0.211585453603786,-0.773580338222786,
-2.53168114763836));
#49079=CARTESIAN_POINT('Ctrl Pts',(-0.0809399864155768,-0.787016451682503,
-2.52639531077971));
#49080=CARTESIAN_POINT('Ctrl Pts',(0.0497054807726323,-0.80045256514222,
-2.52110947392107));
#49081=CARTESIAN_POINT('Ctrl Pts',(0.183768718423527,-0.780656135561986,
-2.51582363706242));
#49082=CARTESIAN_POINT('Ctrl Pts',(0.304954934307039,-0.730033331199104,
-2.51053780020377));
#49083=CARTESIAN_POINT('Ctrl Pts',(0.426141150190555,-0.67941052683622,
-2.50525196334512));
#49084=CARTESIAN_POINT('Ctrl Pts',(0.534450344306686,-0.597961347690689,
-2.49996612648647));
#49085=CARTESIAN_POINT('Ctrl Pts',(0.616718014248558,-0.495585580420968,
-2.49468028962783));
#49086=CARTESIAN_POINT('Ctrl Pts',(0.698985684190429,-0.393209813151246,
-2.48939445276918));
#49087=CARTESIAN_POINT('Ctrl Pts',(0.75521182995804,-0.269907457757338,
-2.48410861591053));
#49088=CARTESIAN_POINT('Ctrl Pts',(0.778562412785546,-0.14066536893429,
-2.47882277905188));
#49089=CARTESIAN_POINT('Ctrl Pts',(0.801912995613052,-0.0114232801112452,
-2.47353694219323));
#49090=CARTESIAN_POINT('Ctrl Pts',(0.792388015500453,0.123758542140946,
-2.46825110533458));
#49091=CARTESIAN_POINT('Ctrl Pts',(0.751145191555912,0.248449346592627,
-2.46296526847594));
#49092=CARTESIAN_POINT('Ctrl Pts',(0.709902367611368,0.373140151044316,
-2.45767943161729));
#49093=CARTESIAN_POINT('Ctrl Pts',(0.636941699834886,0.487339937695493,
-2.45239359475864));
#49094=CARTESIAN_POINT('Ctrl Pts',(0.541131233957833,0.577168228729843,
-2.4471077579));
#49095=CARTESIAN_POINT('Ctrl Pts',(0.445320768080786,0.666996519764187,
-2.44182192104135));
#49096=CARTESIAN_POINT('Ctrl Pts',(0.326660504103166,0.732453315181701,
-2.4365360841827));
#49097=CARTESIAN_POINT('Ctrl Pts',(0.199573071086925,0.765582631671333,
-2.43125024732405));
#49098=CARTESIAN_POINT('Ctrl Pts',(0.0724856380706798,0.798711948160966,
-2.4259644104654));
#49099=CARTESIAN_POINT('Ctrl Pts',(-0.0630289639841951,0.799513785722722,
-2.42067857360676));
#49100=CARTESIAN_POINT('Ctrl Pts',(-0.19049953593827,0.767890684555539,
-2.41539273674811));
#49101=CARTESIAN_POINT('Ctrl Pts',(-0.317970107892348,0.736267583388355,
-2.41010689988946));
#49102=CARTESIAN_POINT('Ctrl Pts',(-0.437396649745624,0.672219543492232,
-2.40482106303081));
#49103=CARTESIAN_POINT('Ctrl Pts',(-0.534263394757312,0.58353132018964,
-2.39953522617216));
#49104=CARTESIAN_POINT('Ctrl Pts',(-0.631130139768997,0.49484309688705,
-2.39424938931352));
#49105=CARTESIAN_POINT('Ctrl Pts',(-0.705437087939093,0.381514690177995,
-2.38896355245487));
#49106=CARTESIAN_POINT('Ctrl Pts',(-0.748152559122481,0.257320665509696,
-2.38367771559622));
#49107=CARTESIAN_POINT('Ctrl Pts',(-0.77655651638456,0.174736962903699,
-2.38016286067205));
#49108=CARTESIAN_POINT('Ctrl Pts',(-0.790991733797414,0.0873488318552603,
-2.37664800574787));
#49109=CARTESIAN_POINT('Ctrl Pts',(-0.791060671368687,-1.7079190050548E-5,
-2.3731331508237));
#49110=CARTESIAN_POINT('Origin',(0.,0.,-2.94));
#49111=CARTESIAN_POINT('',(-0.791097165546451,2.04205267731045E-5,-2.14466684917629));
#49112=CARTESIAN_POINT('',(-0.791081243560257,1.98986687146829E-5,-2.1731331508237));
#49113=CARTESIAN_POINT('',(-0.7911,-9.68818082805471E-17,-2.94));
#49114=CARTESIAN_POINT('Ctrl Pts',(-0.791097165546451,2.04205267731045E-5,
-2.14466684917629));
#49115=CARTESIAN_POINT('Ctrl Pts',(-0.791128923376164,0.0312276790823086,
-2.14592252793373));
#49116=CARTESIAN_POINT('Ctrl Pts',(-0.789317367433578,0.0624312734019356,
-2.14717820669116));
#49117=CARTESIAN_POINT('Ctrl Pts',(-0.785633709697737,0.0934122738038864,
-2.14843388544859));
#49118=CARTESIAN_POINT('Ctrl Pts',(-0.770127184864448,0.223828204529152,
-2.15371972230724));
#49119=CARTESIAN_POINT('Ctrl Pts',(-0.721446504630274,0.350299710200771,
-2.15900555916588));
#49120=CARTESIAN_POINT('Ctrl Pts',(-0.645508589874747,0.457454739956378,
-2.16429139602453));
#49121=CARTESIAN_POINT('Ctrl Pts',(-0.569570675119224,0.564609769711979,
-2.16957723288318));
#49122=CARTESIAN_POINT('Ctrl Pts',(-0.466375525842352,0.652448323551568,
-2.17486306974183));
#49123=CARTESIAN_POINT('Ctrl Pts',(-0.348466054971509,0.710294014646916,
-2.18014890660048));
#49124=CARTESIAN_POINT('Ctrl Pts',(-0.230556584100659,0.768139705742269,
-2.18543474345912));
#49125=CARTESIAN_POINT('Ctrl Pts',(-0.097932791635837,0.795992534093376,
-2.19072058031777));
#49126=CARTESIAN_POINT('Ctrl Pts',(0.0332854883741506,0.790467111886595,
-2.19600641717642));
#49127=CARTESIAN_POINT('Ctrl Pts',(0.164503768384138,0.784941689679814,
-2.20129225403507));
#49128=CARTESIAN_POINT('Ctrl Pts',(0.29431653593929,0.746038016915144,-2.20657809089371));
#49129=CARTESIAN_POINT('Ctrl Pts',(0.406945624607212,0.67848466255597,-2.21186392775236));
#49130=CARTESIAN_POINT('Ctrl Pts',(0.51957471327513,0.610931308196797,-2.21714976461101));
#49131=CARTESIAN_POINT('Ctrl Pts',(0.615020123055817,0.514728272243123,
-2.22243560146966));
#49132=CARTESIAN_POINT('Ctrl Pts',(0.681680887502828,0.40156860724414,-2.22772143832831));
#49133=CARTESIAN_POINT('Ctrl Pts',(0.748341651949842,0.288408942245151,
-2.23300727518695));
#49134=CARTESIAN_POINT('Ctrl Pts',(0.786217771063174,0.158292648200854,
-2.2382931120456));
#49135=CARTESIAN_POINT('Ctrl Pts',(0.790705570470584,0.0270347838428554,
-2.24357894890425));
#49136=CARTESIAN_POINT('Ctrl Pts',(0.795193369877993,-0.104223080515135,
-2.2488647857629));
#49137=CARTESIAN_POINT('Ctrl Pts',(0.766292849579479,-0.236622515186834,
-2.25415062262155));
#49138=CARTESIAN_POINT('Ctrl Pts',(0.70751673970045,-0.354070955818585,
-2.25943645948019));
#49139=CARTESIAN_POINT('Ctrl Pts',(0.648740629821416,-0.471519396450344,
-2.26472229633884));
#49140=CARTESIAN_POINT('Ctrl Pts',(0.560088930361871,-0.574016843042153,
-2.27000813319749));
#49141=CARTESIAN_POINT('Ctrl Pts',(0.452336862395436,-0.649105185335084,
-2.27529397005613));
#49142=CARTESIAN_POINT('Ctrl Pts',(0.344584794429007,-0.72419352762801,
-2.28057980691478));
#49143=CARTESIAN_POINT('Ctrl Pts',(0.217732357955687,-0.771872765622055,
-2.28586564377343));
#49144=CARTESIAN_POINT('Ctrl Pts',(0.0871979042881309,-0.786347699302541,
-2.29115148063208));
#49145=CARTESIAN_POINT('Ctrl Pts',(-0.0433365493794288,-0.800822632983027,
-2.29643731749073));
#49146=CARTESIAN_POINT('Ctrl Pts',(-0.177553020241233,-0.782093262349958,
-2.30172315434938));
#49147=CARTESIAN_POINT('Ctrl Pts',(-0.299138091249714,-0.732436059375915,
-2.30700899120802));
#49148=CARTESIAN_POINT('Ctrl Pts',(-0.420723162258195,-0.682778856401872,
-2.31229482806667));
#49149=CARTESIAN_POINT('Ctrl Pts',(-0.529676833413351,-0.602193821086856,
-2.31758066492532));
#49150=CARTESIAN_POINT('Ctrl Pts',(-0.612756268981202,-0.500475707237502,
-2.32286650178397));
#49151=CARTESIAN_POINT('Ctrl Pts',(-0.69583570454905,-0.398757593388151,
-2.32815233864261));
#49152=CARTESIAN_POINT('Ctrl Pts',(-0.753040904529592,-0.275906401004465,
-2.33343817550126));
#49153=CARTESIAN_POINT('Ctrl Pts',(-0.77741883045758,-0.146854147917619,
-2.33872401235991));
#49154=CARTESIAN_POINT('Ctrl Pts',(-0.786554819049114,-0.0984899057997243,
-2.34070495796537));
#49155=CARTESIAN_POINT('Ctrl Pts',(-0.791080261084932,-0.0492547330337058,
-2.34268590357083));
#49156=CARTESIAN_POINT('Ctrl Pts',(-0.791049211918833,-1.3923086196882E-5,
-2.3446668491763));
#49157=CARTESIAN_POINT('Ctrl Pts',(-0.791060671368687,-1.7079190050548E-5,
-2.3731331508237));
#49158=CARTESIAN_POINT('Ctrl Pts',(-0.791095406000973,-0.0440369472892742,
-2.37136216888922));
#49159=CARTESIAN_POINT('Ctrl Pts',(-0.78748295578056,-0.0880511743694083,
-2.36959118695475));
#49160=CARTESIAN_POINT('Ctrl Pts',(-0.780172469530915,-0.131442361535027,
-2.36782020502028));
#49161=CARTESIAN_POINT('Ctrl Pts',(-0.758352914559283,-0.260951721283921,
-2.36253436816163));
#49162=CARTESIAN_POINT('Ctrl Pts',(-0.703589810419337,-0.384910798154171,
-2.35724853130298));
#49163=CARTESIAN_POINT('Ctrl Pts',(-0.62253936965279,-0.488252915866539,
-2.35196269444433));
#49164=CARTESIAN_POINT('Ctrl Pts',(-0.541488928886243,-0.591595033578908,
-2.34667685758569));
#49165=CARTESIAN_POINT('Ctrl Pts',(-0.434151151493092,-0.674320192133397,
-2.34139102072704));
#49166=CARTESIAN_POINT('Ctrl Pts',(-0.313572468483857,-0.726373515230843,
-2.33610518386839));
#49167=CARTESIAN_POINT('Ctrl Pts',(-0.192993785474619,-0.77842683832829,
-2.33081934700974));
#49168=CARTESIAN_POINT('Ctrl Pts',(-0.059174196849305,-0.799808325968691,
-2.32553351015109));
#49169=CARTESIAN_POINT('Ctrl Pts',(0.0716211196209889,-0.787919153114142,
-2.32024767329245));
#49170=CARTESIAN_POINT('Ctrl Pts',(0.202416436091275,-0.776029980259594,
-2.3149618364338));
#49171=CARTESIAN_POINT('Ctrl Pts',(0.330187480406542,-0.730870146910091,
-2.30967599957515));
#49172=CARTESIAN_POINT('Ctrl Pts',(0.43940424854316,-0.657928630614363,
-2.3043901627165));
#49173=CARTESIAN_POINT('Ctrl Pts',(0.548621016679781,-0.584987114318634,
-2.29910432585786));
#49174=CARTESIAN_POINT('Ctrl Pts',(0.639283508637765,-0.484263915076674,
-2.29381848899921));
#49175=CARTESIAN_POINT('Ctrl Pts',(0.700372100429191,-0.368001491247351,
-2.28853265214056));
#49176=CARTESIAN_POINT('Ctrl Pts',(0.761460692220617,-0.251739067418028,
-2.28324681528191));
#49177=CARTESIAN_POINT('Ctrl Pts',(0.792975383845487,-0.11993741900134,
-2.27796097842326));
#49178=CARTESIAN_POINT('Ctrl Pts',(0.791085704242379,0.0113835479183653,
-2.27267514156462));
#49179=CARTESIAN_POINT('Ctrl Pts',(0.789196024639272,0.142704514838074,
-2.26738930470597));
#49180=CARTESIAN_POINT('Ctrl Pts',(0.75390197380819,0.273544800260791,-2.26210346784732));
#49181=CARTESIAN_POINT('Ctrl Pts',(0.689493387168049,0.388001347512353,
-2.25681763098867));
#49182=CARTESIAN_POINT('Ctrl Pts',(0.625084800527912,0.502457894763909,
-2.25153179413003));
#49183=CARTESIAN_POINT('Ctrl Pts',(0.531561678078721,0.600530703844302,
-2.24624595727138));
#49184=CARTESIAN_POINT('Ctrl Pts',(0.420291340763339,0.670299459569546,
-2.24096012041273));
#49185=CARTESIAN_POINT('Ctrl Pts',(0.309021003447957,0.74006821529479,-2.23567428355408));
#49186=CARTESIAN_POINT('Ctrl Pts',(0.180003451266383,0.781532917664886,
-2.23038844669544));
#49187=CARTESIAN_POINT('Ctrl Pts',(0.0489201957475688,0.78965371592103,
-2.22510260983679));
#49188=CARTESIAN_POINT('Ctrl Pts',(-0.0821630597712489,0.797774514177174,
-2.21981677297814));
#49189=CARTESIAN_POINT('Ctrl Pts',(-0.215312018627309,0.772551408319364,
-2.21453093611949));
#49190=CARTESIAN_POINT('Ctrl Pts',(-0.334343015125024,0.717050155049826,
-2.20924509926084));
#49191=CARTESIAN_POINT('Ctrl Pts',(-0.453374011622743,0.661548901780285,
-2.20395926240219));
#49192=CARTESIAN_POINT('Ctrl Pts',(-0.558287045762119,0.575769501099013,
-2.19867342554355));
#49193=CARTESIAN_POINT('Ctrl Pts',(-0.636330403326168,0.470138058896137,
-2.1933875886849));
#49194=CARTESIAN_POINT('Ctrl Pts',(-0.714373760890212,0.364506616693267,
-2.18810175182625));
#49195=CARTESIAN_POINT('Ctrl Pts',(-0.765547441878935,0.239023132968793,
-2.1828159149676));
#49196=CARTESIAN_POINT('Ctrl Pts',(-0.783631512222635,0.10893956889734,
-2.17753007810896));
#49197=CARTESIAN_POINT('Ctrl Pts',(-0.788645813927934,0.0728703530207205,
-2.17606443568054));
#49198=CARTESIAN_POINT('Ctrl Pts',(-0.791116097488508,0.036447470611259,
-2.17459879325212));
#49199=CARTESIAN_POINT('Ctrl Pts',(-0.791081243560257,1.98986687146829E-5,
-2.1731331508237));
#49200=CARTESIAN_POINT('Origin',(0.,0.,-2.94));
#49201=CARTESIAN_POINT('',(-0.791132802071856,-1.71669250316198E-5,-1.94466684917629));
#49202=CARTESIAN_POINT('',(-0.791147029519077,-1.37720429744394E-5,-1.9731331508237));
#49203=CARTESIAN_POINT('',(-0.7911,-9.68818082805471E-17,-2.94));
#49204=CARTESIAN_POINT('Ctrl Pts',(-0.791132802071856,-1.71669250316198E-5,
-1.94466684917629));
#49205=CARTESIAN_POINT('Ctrl Pts',(-0.791026522766624,0.111615095251917,
-1.94915915229662));
#49206=CARTESIAN_POINT('Ctrl Pts',(-0.767167347256203,0.223291341687766,
-1.95365145541694));
#49207=CARTESIAN_POINT('Ctrl Pts',(-0.721308735469413,0.32505366763991,
-1.95814375853727));
#49208=CARTESIAN_POINT('Ctrl Pts',(-0.667349522572057,0.444791592470935,
-1.96342959539592));
#49209=CARTESIAN_POINT('Ctrl Pts',(-0.582932339520027,0.550803806769426,
-1.96871543225456));
#49210=CARTESIAN_POINT('Ctrl Pts',(-0.47831772068937,0.630204995842756,
-1.97400126911321));
#49211=CARTESIAN_POINT('Ctrl Pts',(-0.373703101858712,0.709606184916085,
-1.97928710597186));
#49212=CARTESIAN_POINT('Ctrl Pts',(-0.248891047249423,0.762396348764255,
-1.98457294283051));
#49213=CARTESIAN_POINT('Ctrl Pts',(-0.119051908803644,0.782159076991918,
-1.98985877968915));
#49214=CARTESIAN_POINT('Ctrl Pts',(0.0107872296421378,0.801921805219581,
-1.9951446165478));
#49215=CARTESIAN_POINT('Ctrl Pts',(0.145653451924402,0.788657097826737,
-2.00043045340645));
#49216=CARTESIAN_POINT('Ctrl Pts',(0.269154366590807,0.743977221194132,
-2.0057162902651));
#49217=CARTESIAN_POINT('Ctrl Pts',(0.392655281257209,0.699297344561529,
-2.01100212712375));
#49218=CARTESIAN_POINT('Ctrl Pts',(0.504790888307744,0.623202298689167,
-2.01628796398239));
#49219=CARTESIAN_POINT('Ctrl Pts',(0.591931601805962,0.524941099071189,
-2.02157380084104));
#49220=CARTESIAN_POINT('Ctrl Pts',(0.67907231530418,0.426679899453212,-2.02685963769969));
#49221=CARTESIAN_POINT('Ctrl Pts',(0.741218135250083,0.306252546089617,
-2.03214547455834));
#49222=CARTESIAN_POINT('Ctrl Pts',(0.770815512723548,0.178296449923644,
-2.03743131141698));
#49223=CARTESIAN_POINT('Ctrl Pts',(0.800412890197013,0.0503403537576715,
-2.04271714827563));
#49224=CARTESIAN_POINT('Ctrl Pts',(0.797461825198041,-0.0851444852106823,
-2.04800298513428));
#49225=CARTESIAN_POINT('Ctrl Pts',(0.762321006595096,-0.211690485413207,
-2.05328882199293));
#49226=CARTESIAN_POINT('Ctrl Pts',(0.727180187992152,-0.338236485615732,
-2.05857465885158));
#49227=CARTESIAN_POINT('Ctrl Pts',(0.659849615785234,-0.455843647052432,
-2.06386049571022));
#49228=CARTESIAN_POINT('Ctrl Pts',(0.568513022547629,-0.550217340606783,
-2.06914633256887));
#49229=CARTESIAN_POINT('Ctrl Pts',(0.477176429310023,-0.644591034161134,
-2.07443216942752));
#49230=CARTESIAN_POINT('Ctrl Pts',(0.361833815041726,-0.715731259833139,
-2.07971800628617));
#49231=CARTESIAN_POINT('Ctrl Pts',(0.236504563189749,-0.754991238559142,
-2.08500384314482));
#49232=CARTESIAN_POINT('Ctrl Pts',(0.111175311337768,-0.794251217285145,
-2.09028968000346));
#49233=CARTESIAN_POINT('Ctrl Pts',(-0.0241405780978863,-0.801630949065144,
-2.09557551686211));
#49234=CARTESIAN_POINT('Ctrl Pts',(-0.152996058615766,-0.776233460215857,
-2.10086135372076));
#49235=CARTESIAN_POINT('Ctrl Pts',(-0.281851539133642,-0.75083597136657,
-2.10614719057941));
#49236=CARTESIAN_POINT('Ctrl Pts',(-0.404246610733737,-0.692661261887995,
-2.11143302743805));
#49237=CARTESIAN_POINT('Ctrl Pts',(-0.505304695044117,-0.608780209827005,
-2.1167188642967));
#49238=CARTESIAN_POINT('Ctrl Pts',(-0.606362779354498,-0.524899157766015,
-2.12200470115535));
#49239=CARTESIAN_POINT('Ctrl Pts',(-0.686083876375167,-0.415311763122608,
-2.127290538014));
#49240=CARTESIAN_POINT('Ctrl Pts',(-0.734778240169299,-0.293337887911449,
-2.13257637487265));
#49241=CARTESIAN_POINT('Ctrl Pts',(-0.771904997951733,-0.200339557757781,
-2.13660653297386));
#49242=CARTESIAN_POINT('Ctrl Pts',(-0.790995237347112,-0.10014069563447,
-2.14063669107508));
#49243=CARTESIAN_POINT('Ctrl Pts',(-0.791097165546451,2.04205267731045E-5,
-2.14466684917629));
#49244=CARTESIAN_POINT('Ctrl Pts',(-0.791081243560257,1.98986687146829E-5,
-2.1731331508237));
#49245=CARTESIAN_POINT('Ctrl Pts',(-0.790990396857139,-0.0949285039861595,
-2.16931295639347));
#49246=CARTESIAN_POINT('Ctrl Pts',(-0.773880064045768,-0.189908766546335,
-2.16549276196324));
#49247=CARTESIAN_POINT('Ctrl Pts',(-0.740438748222271,-0.278741164435588,
-2.16167256753301));
#49248=CARTESIAN_POINT('Ctrl Pts',(-0.694167454179532,-0.401654689278622,
-2.15638673067437));
#49249=CARTESIAN_POINT('Ctrl Pts',(-0.61663040639538,-0.512798094546253,
-2.15110089381572));
#49250=CARTESIAN_POINT('Ctrl Pts',(-0.517251889303895,-0.598662392030284,
-2.14581505695707));
#49251=CARTESIAN_POINT('Ctrl Pts',(-0.41787337221241,-0.684526689514316,
-2.14052922009842));
#49252=CARTESIAN_POINT('Ctrl Pts',(-0.296653385813593,-0.745111879214747,
-2.13524338323977));
#49253=CARTESIAN_POINT('Ctrl Pts',(-0.168325682082346,-0.773054099899473,
-2.12995754638113));
#49254=CARTESIAN_POINT('Ctrl Pts',(-0.0399979783510983,-0.800996320584199,
-2.12467170952248));
#49255=CARTESIAN_POINT('Ctrl Pts',(0.095437442712579,-0.79629557225322,
-2.11938587266383));
#49256=CARTESIAN_POINT('Ctrl Pts',(0.221519006067722,-0.759523210027606,
-2.11410003580518));
#49257=CARTESIAN_POINT('Ctrl Pts',(0.347600569422865,-0.722750847801993,
-2.10881419894653));
#49258=CARTESIAN_POINT('Ctrl Pts',(0.464328275069475,-0.653906871681745,
-2.10352836208789));
#49259=CARTESIAN_POINT('Ctrl Pts',(0.557514387843661,-0.561358961776846,
-2.09824252522924));
#49260=CARTESIAN_POINT('Ctrl Pts',(0.650700500617848,-0.468811051871947,
-2.09295668837059));
#49261=CARTESIAN_POINT('Ctrl Pts',(0.720345020519613,-0.352559208182397,
-2.08767085151194));
#49262=CARTESIAN_POINT('Ctrl Pts',(0.757982964891162,-0.226733326960715,
-2.08238501465329));
#49263=CARTESIAN_POINT('Ctrl Pts',(0.795620909262712,-0.100907445739033,
-2.07709917779465));
#49264=CARTESIAN_POINT('Ctrl Pts',(0.801252278104046,0.0344924730147816,
-2.071813340936));
#49265=CARTESIAN_POINT('Ctrl Pts',(0.774192603496531,0.163009169408146,
-2.06652750407735));
#49266=CARTESIAN_POINT('Ctrl Pts',(0.747132928889016,0.29152586580151,-2.0612416672187));
#49267=CARTESIAN_POINT('Ctrl Pts',(0.687382210832651,0.413159339834423,
-2.05595583036006));
#49268=CARTESIAN_POINT('Ctrl Pts',(0.602202884230443,0.513125581943063,
-2.05066999350141));
#49269=CARTESIAN_POINT('Ctrl Pts',(0.517023557628235,0.613091824051702,
-2.04538415664276));
#49270=CARTESIAN_POINT('Ctrl Pts',(0.406415622480184,0.691390834236067,
-2.04009831978411));
#49271=CARTESIAN_POINT('Ctrl Pts',(0.283822982975207,0.738505714910133,
-2.03481248292547));
#49272=CARTESIAN_POINT('Ctrl Pts',(0.16123034347023,0.785620595584199,-2.02952664606682));
#49273=CARTESIAN_POINT('Ctrl Pts',(0.0266529996083376,0.801551346747966,
-2.02424080920817));
#49274=CARTESIAN_POINT('Ctrl Pts',(-0.103551769049521,0.784361656218983,
-2.01895497234952));
#49275=CARTESIAN_POINT('Ctrl Pts',(-0.233756537707379,0.76717196569,-2.01366913549088));
#49276=CARTESIAN_POINT('Ctrl Pts',(-0.359588731161204,0.716861833468259,
-2.00838329863223));
#49277=CARTESIAN_POINT('Ctrl Pts',(-0.46575400411459,0.639546233098982,
-2.00309746177358));
#49278=CARTESIAN_POINT('Ctrl Pts',(-0.571919277067976,0.562230632729704,
-1.99781162491493));
#49279=CARTESIAN_POINT('Ctrl Pts',(-0.658417629520933,0.457909564212886,
-1.99252578805628));
#49280=CARTESIAN_POINT('Ctrl Pts',(-0.714735570182623,0.339262790968288,
-1.98723995119764));
#49281=CARTESIAN_POINT('Ctrl Pts',(-0.764835864461531,0.233714928511718,
-1.98253768440632));
#49282=CARTESIAN_POINT('Ctrl Pts',(-0.791051877136207,0.116829938905797,
-1.97783541761501));
#49283=CARTESIAN_POINT('Ctrl Pts',(-0.791147029519077,-1.37720429744394E-5,
-1.9731331508237));
#49284=CARTESIAN_POINT('Origin',(0.,0.,-2.94));
#49285=CARTESIAN_POINT('',(-0.79103421667841,4.57183632199265E-6,-1.74466684917629));
#49286=CARTESIAN_POINT('',(-0.791032665677869,-2.33805119084811E-7,-1.7731331508237));
#49287=CARTESIAN_POINT('',(-0.7911,-9.68818082805471E-17,-2.94));
#49288=CARTESIAN_POINT('Ctrl Pts',(-0.79103421667841,4.57183632199265E-6,
-1.74466684917629));
#49289=CARTESIAN_POINT('Ctrl Pts',(-0.791046491980383,0.0607363198089551,
-1.74710993980086));
#49290=CARTESIAN_POINT('Ctrl Pts',(-0.784141006924924,0.121465321068842,
-1.74955303042543));
#49291=CARTESIAN_POINT('Ctrl Pts',(-0.770287134004301,0.18056552798937,
-1.75199612105));
#49292=CARTESIAN_POINT('Ctrl Pts',(-0.740313087449333,0.30843391279368,
-1.75728195790865));
#49293=CARTESIAN_POINT('Ctrl Pts',(-0.677812909732563,0.42867774074456,
-1.7625677947673));
#49294=CARTESIAN_POINT('Ctrl Pts',(-0.590383220390283,0.526681907599112,
-1.76785363162595));
#49295=CARTESIAN_POINT('Ctrl Pts',(-0.502953531048003,0.624686074453665,
-1.77313946848459));
#49296=CARTESIAN_POINT('Ctrl Pts',(-0.390594330080212,0.70045058021189,
-1.77842530534324));
#49297=CARTESIAN_POINT('Ctrl Pts',(-0.266962380272803,0.744766585065227,
-1.78371114220189));
#49298=CARTESIAN_POINT('Ctrl Pts',(-0.143330430465394,0.789082589918563,
-1.78899697906054));
#49299=CARTESIAN_POINT('Ctrl Pts',(-0.00842573181836657,0.801950093867011,
-1.79428281591919));
#49300=CARTESIAN_POINT('Ctrl Pts',(0.12135464758435,0.781805108847671,-1.79956865277783));
#49301=CARTESIAN_POINT('Ctrl Pts',(0.251135026987067,0.761660123828331,
-1.80485448963648));
#49302=CARTESIAN_POINT('Ctrl Pts',(0.375791087145474,0.708502649841203,
-1.81014032649513));
#49303=CARTESIAN_POINT('Ctrl Pts',(0.480171436551409,0.628793742200729,
-1.81542616335378));
#49304=CARTESIAN_POINT('Ctrl Pts',(0.584551785957344,0.549084834560255,
-1.82071200021242));
#49305=CARTESIAN_POINT('Ctrl Pts',(0.668656424610807,0.442824493266436,
-1.82599783707107));
#49306=CARTESIAN_POINT('Ctrl Pts',(0.722262806521882,0.322928191748221,
-1.83128367392972));
#49307=CARTESIAN_POINT('Ctrl Pts',(0.775869188432956,0.203031890230006,
-1.83656951078837));
#49308=CARTESIAN_POINT('Ctrl Pts',(0.798977313601642,0.0694996284873965,
-1.84185534764702));
#49309=CARTESIAN_POINT('Ctrl Pts',(0.788778491852706,-0.0614383390173576,
-1.84714118450566));
#49310=CARTESIAN_POINT('Ctrl Pts',(0.778579670103769,-0.192376306522112,
-1.85242702136431));
#49311=CARTESIAN_POINT('Ctrl Pts',(0.73507390143721,-0.32071997978901,-1.85771285822296));
#49312=CARTESIAN_POINT('Ctrl Pts',(0.663549119172057,-0.430869754283854,
-1.86299869508161));
#49313=CARTESIAN_POINT('Ctrl Pts',(0.592024336906903,-0.541019528778699,
-1.86828453194025));
#49314=CARTESIAN_POINT('Ctrl Pts',(0.492480541043156,-0.632975404501489,
-1.8735703687989));
#49315=CARTESIAN_POINT('Ctrl Pts',(0.37701683868739,-0.695560552401304,
-1.87885620565755));
#49316=CARTESIAN_POINT('Ctrl Pts',(0.261553136331624,-0.758145700301119,
-1.8841420425162));
#49317=CARTESIAN_POINT('Ctrl Pts',(0.130169527483839,-0.791360120377959,
-1.88942787937485));
#49318=CARTESIAN_POINT('Ctrl Pts',(-0.00116489262803629,-0.791166747112014,
-1.89471371623349));
#49319=CARTESIAN_POINT('Ctrl Pts',(-0.132499312739904,-0.79097337384607,
-1.89999955309214));
#49320=CARTESIAN_POINT('Ctrl Pts',(-0.263784544115863,-0.757372207237345,
-1.90528538995079));
#49321=CARTESIAN_POINT('Ctrl Pts',(-0.379063448873576,-0.69444732013214,
-1.91057122680944));
#49322=CARTESIAN_POINT('Ctrl Pts',(-0.494342353631296,-0.631522433026931,
-1.91585706366809));
#49323=CARTESIAN_POINT('Ctrl Pts',(-0.593614931770767,-0.539273825425238,
-1.92114290052673));
#49324=CARTESIAN_POINT('Ctrl Pts',(-0.664815041497486,-0.428913906640175,
-1.92642873738538));
#49325=CARTESIAN_POINT('Ctrl Pts',(-0.736015151224201,-0.318553987855117,
-1.93171457424403));
#49326=CARTESIAN_POINT('Ctrl Pts',(-0.779142792538166,-0.190082757886691,
-1.93700041110267));
#49327=CARTESIAN_POINT('Ctrl Pts',(-0.78895599182381,-0.0591153252206997,
-1.94228624796132));
#49328=CARTESIAN_POINT('Ctrl Pts',(-0.790429193688017,-0.0394539018318772,
-1.94307978169965));
#49329=CARTESIAN_POINT('Ctrl Pts',(-0.791151575563343,-0.0197362205930797,
-1.94387331543797));
#49330=CARTESIAN_POINT('Ctrl Pts',(-0.791132802071856,-1.71669250316198E-5,
-1.94466684917629));
#49331=CARTESIAN_POINT('Ctrl Pts',(-0.791147029519077,-1.37720429744394E-5,
-1.9731331508237));
#49332=CARTESIAN_POINT('Ctrl Pts',(-0.791158838309378,-0.0145145426908869,
-1.97254958075636));
#49333=CARTESIAN_POINT('Ctrl Pts',(-0.790768338829755,-0.0290146775731718,
-1.97196601068903));
#49334=CARTESIAN_POINT('Ctrl Pts',(-0.789971256028148,-0.043492427722329,
-1.97138244062169));
#49335=CARTESIAN_POINT('Ctrl Pts',(-0.78275147234156,-0.174628395195968,
-1.96609660376304));
#49336=CARTESIAN_POINT('Ctrl Pts',(-0.742174376097962,-0.303927852170872,
-1.9608107669044));
#49337=CARTESIAN_POINT('Ctrl Pts',(-0.673171933466268,-0.415675022840148,
-1.95552493004575));
#49338=CARTESIAN_POINT('Ctrl Pts',(-0.604169490834576,-0.52742219350942,
-1.9502390931871));
#49339=CARTESIAN_POINT('Ctrl Pts',(-0.506741701814794,-0.621617077873063,
-1.94495325632845));
#49340=CARTESIAN_POINT('Ctrl Pts',(-0.392730482261924,-0.686810705305464,
-1.93966741946981));
#49341=CARTESIAN_POINT('Ctrl Pts',(-0.27871926270905,-0.752004332737866,
-1.93438158261116));
#49342=CARTESIAN_POINT('Ctrl Pts',(-0.14812461262309,-0.788196703239019,
-1.92909574575251));
#49343=CARTESIAN_POINT('Ctrl Pts',(-0.0168197327919539,-0.790988794616383,
-1.92380990889386));
#49344=CARTESIAN_POINT('Ctrl Pts',(0.114485147039182,-0.793780885993746,
-1.91852407203521));
#49345=CARTESIAN_POINT('Ctrl Pts',(0.246500256615497,-0.763172698247319,
-1.91323823517657));
#49346=CARTESIAN_POINT('Ctrl Pts',(0.363179744594969,-0.702884520910657,
-1.90795239831792));
#49347=CARTESIAN_POINT('Ctrl Pts',(0.479859232574441,-0.642596343573996,
-1.90266656145927));
#49348=CARTESIAN_POINT('Ctrl Pts',(0.581203098957073,-0.552628176647096,
-1.89738072460062));
#49349=CARTESIAN_POINT('Ctrl Pts',(0.654893446044485,-0.443915251988317,
-1.89209488774197));
#49350=CARTESIAN_POINT('Ctrl Pts',(0.728583793131896,-0.335202327329538,
-1.88680905088333));
#49351=CARTESIAN_POINT('Ctrl Pts',(0.774620620924088,-0.207744644938874,
-1.88152321402468));
#49352=CARTESIAN_POINT('Ctrl Pts',(0.787408357085573,-0.0770341210871483,
-1.87623737716603));
#49353=CARTESIAN_POINT('Ctrl Pts',(0.800196093247058,0.0536764027645815,
-1.87095154030738));
#49354=CARTESIAN_POINT('Ctrl Pts',(0.779734737777836,0.18763976807737,-1.86566570344874));
#49355=CARTESIAN_POINT('Ctrl Pts',(0.72851127772938,0.308573321661119,-1.86037986659009));
#49356=CARTESIAN_POINT('Ctrl Pts',(0.677287817680926,0.429506875244866,
-1.85509402973144));
#49357=CARTESIAN_POINT('Ctrl Pts',(0.595302253053237,0.537410617099569,
-1.84980819287279));
#49358=CARTESIAN_POINT('Ctrl Pts',(0.492519565782321,0.619169325743342,
-1.84452235601415));
#49359=CARTESIAN_POINT('Ctrl Pts',(0.389736878511398,0.700928034387121,
-1.8392365191555));
#49360=CARTESIAN_POINT('Ctrl Pts',(0.266157068597242,0.75654170981997,-1.83395068229685));
#49361=CARTESIAN_POINT('Ctrl Pts',(0.13680071410188,0.779250756330134,-1.8286648454382));
#49362=CARTESIAN_POINT('Ctrl Pts',(0.00744435960653334,0.801959802840296,
-1.82337900857955));
#49363=CARTESIAN_POINT('Ctrl Pts',(-0.127688539470023,0.79176422042778,
-1.81809317172091));
#49364=CARTESIAN_POINT('Ctrl Pts',(-0.252173178293266,0.749903236937503,
-1.81280733486226));
#49365=CARTESIAN_POINT('Ctrl Pts',(-0.376657817116519,0.708042253447222,
-1.80752149800361));
#49366=CARTESIAN_POINT('Ctrl Pts',(-0.490494195686453,0.634515868879179,
-1.80223566114496));
#49367=CARTESIAN_POINT('Ctrl Pts',(-0.579846006828024,0.53826088933292,
-1.79694982428631));
#49368=CARTESIAN_POINT('Ctrl Pts',(-0.669197817969591,0.442005909786664,
-1.79166398742767));
#49369=CARTESIAN_POINT('Ctrl Pts',(-0.73406506168279,0.323022335262195,
-1.78637815056902));
#49370=CARTESIAN_POINT('Ctrl Pts',(-0.766563412052733,0.195772091785175,
-1.78109231371037));
#49371=CARTESIAN_POINT('Ctrl Pts',(-0.782874904509492,0.131902961107212,
-1.77843925941482));
#49372=CARTESIAN_POINT('Ctrl Pts',(-0.791031985578626,0.0659512810282034,
-1.77578620511926));
#49373=CARTESIAN_POINT('Ctrl Pts',(-0.791032665677869,-2.33805119084811E-7,
-1.7731331508237));
#49374=CARTESIAN_POINT('Origin',(0.,0.,-2.94));
#49375=CARTESIAN_POINT('',(-0.791157484722713,9.84224722326565E-6,-1.54466684917629));
#49376=CARTESIAN_POINT('',(-0.791145759608552,1.41466495050277E-5,-1.5731331508237));
#49377=CARTESIAN_POINT('',(-0.7911,-9.68818082805471E-17,-2.94));
#49378=CARTESIAN_POINT('Ctrl Pts',(-0.791157484722713,9.84224722326565E-6,
-1.54466684917629));
#49379=CARTESIAN_POINT('Ctrl Pts',(-0.791163583645489,0.0097967005803917,
-1.54506072730511));
#49380=CARTESIAN_POINT('Ctrl Pts',(-0.790985743924691,0.0195833369757562,
-1.54545460543392));
#49381=CARTESIAN_POINT('Ctrl Pts',(-0.7906225317606,0.0293630887867682,
-1.54584848356274));
#49382=CARTESIAN_POINT('Ctrl Pts',(-0.785748231554505,0.160607168641227,
-1.55113432042139));
#49383=CARTESIAN_POINT('Ctrl Pts',(-0.747489118033617,0.290611363217802,
-1.55642015728003));
#49384=CARTESIAN_POINT('Ctrl Pts',(-0.680495416842589,0.403574238978249,
-1.56170599413868));
#49385=CARTESIAN_POINT('Ctrl Pts',(-0.61350171565156,0.516537114738695,
-1.56699183099733));
#49386=CARTESIAN_POINT('Ctrl Pts',(-0.517773426790394,0.612458671683009,
-1.57227766785598));
#49387=CARTESIAN_POINT('Ctrl Pts',(-0.404945899403756,0.679680069787782,
-1.57756350471462));
#49388=CARTESIAN_POINT('Ctrl Pts',(-0.292118372017125,0.74690146789255,
-1.58284934157327));
#49389=CARTESIAN_POINT('Ctrl Pts',(-0.162191606105027,0.785422707157778,
-1.58813517843192));
#49390=CARTESIAN_POINT('Ctrl Pts',(-0.0309576240947823,0.7905617017166,
-1.59342101529057));
#49391=CARTESIAN_POINT('Ctrl Pts',(0.100276357915478,0.795700696275423,
-1.59870685214922));
#49392=CARTESIAN_POINT('Ctrl Pts',(0.232817556023881,0.767457446127832,
-1.60399268900786));
#49393=CARTESIAN_POINT('Ctrl Pts',(0.350556175159501,0.709264793126081,
-1.60927852586651));
#49394=CARTESIAN_POINT('Ctrl Pts',(0.468294794295108,0.651072140124337,
-1.61456436272516));
#49395=CARTESIAN_POINT('Ctrl Pts',(0.571230834457931,0.562930084268443,
-1.61985019958381));
#49396=CARTESIAN_POINT('Ctrl Pts',(0.646852876284771,0.455551901711275,
-1.62513603644245));
#49397=CARTESIAN_POINT('Ctrl Pts',(0.72247491811162,0.348173719154094,-1.6304218733011));
#49398=CARTESIAN_POINT('Ctrl Pts',(0.770782961602475,0.221559409895639,
-1.63570771015975));
#49399=CARTESIAN_POINT('Ctrl Pts',(0.785905378222046,0.0910983819411992,
-1.6409935470184));
#49400=CARTESIAN_POINT('Ctrl Pts',(0.801027794841615,-0.0393626460132327,
-1.64627938387705));
#49401=CARTESIAN_POINT('Ctrl Pts',(0.782964584589898,-0.173670392663664,
-1.6515652207357));
#49402=CARTESIAN_POINT('Ctrl Pts',(0.733911250598238,-0.295500346795009,
-1.65685105759434));
#49403=CARTESIAN_POINT('Ctrl Pts',(0.684857916606581,-0.417330300926347,
-1.66213689445299));
#49404=CARTESIAN_POINT('Ctrl Pts',(0.604814458874985,-0.526682462538616,
-1.66742273131164));
#49405=CARTESIAN_POINT('Ctrl Pts',(0.503509804855647,-0.610265561149299,
-1.67270856817029));
#49406=CARTESIAN_POINT('Ctrl Pts',(0.402205150836304,-0.693848659759987,
-1.67799440502893));
#49407=CARTESIAN_POINT('Ctrl Pts',(0.279639300529219,-0.751662695369081,
-1.68328024188758));
#49408=CARTESIAN_POINT('Ctrl Pts',(0.150709589701088,-0.776680628239671,
-1.68856607874623));
#49409=CARTESIAN_POINT('Ctrl Pts',(0.021779878872957,-0.801698561110261,
-1.69385191560488));
#49410=CARTESIAN_POINT('Ctrl Pts',(-0.113513692476217,-0.793920391242345,
-1.69913775246353));
#49411=CARTESIAN_POINT('Ctrl Pts',(-0.238726790509447,-0.754291520702506,
-1.70442358932217));
#49412=CARTESIAN_POINT('Ctrl Pts',(-0.363939888542678,-0.714662650162667,
-1.70970942618082));
#49413=CARTESIAN_POINT('Ctrl Pts',(-0.479072513259962,-0.643183078950906,
-1.71499526303947));
#49414=CARTESIAN_POINT('Ctrl Pts',(-0.570130804513331,-0.548540832076904,
-1.72028109989812));
#49415=CARTESIAN_POINT('Ctrl Pts',(-0.6611890957667,-0.453898585202903,
-1.72556693675676));
#49416=CARTESIAN_POINT('Ctrl Pts',(-0.728173053556152,-0.336093662666664,
-1.73085277361541));
#49417=CARTESIAN_POINT('Ctrl Pts',(-0.762941074754295,-0.209444730569673,
-1.73613861047406));
#49418=CARTESIAN_POINT('Ctrl Pts',(-0.781639468967064,-0.141332379697595,
-1.73898135670814));
#49419=CARTESIAN_POINT('Ctrl Pts',(-0.79101993330795,-0.070662044498731,
-1.74182410294222));
#49420=CARTESIAN_POINT('Ctrl Pts',(-0.79103421667841,4.57183632199265E-6,
-1.74466684917629));
#49421=CARTESIAN_POINT('Ctrl Pts',(-0.791032665677869,-2.33805119084811E-7,
-1.7731331508237));
#49422=CARTESIAN_POINT('Ctrl Pts',(-0.791033340580539,-0.0654478194626728,
-1.77050036826061));
#49423=CARTESIAN_POINT('Ctrl Pts',(-0.783001782864027,-0.130895242390146,
-1.76786758569752));
#49424=CARTESIAN_POINT('Ctrl Pts',(-0.766936048205097,-0.194307165548313,
-1.76523480313443));
#49425=CARTESIAN_POINT('Ctrl Pts',(-0.734680876960827,-0.321619266975207,
-1.75994896627578));
#49426=CARTESIAN_POINT('Ctrl Pts',(-0.670041077445598,-0.440726557399418,
-1.75466312941713));
#49427=CARTESIAN_POINT('Ctrl Pts',(-0.580873330740293,-0.537152073676115,
-1.74937729255848));
#49428=CARTESIAN_POINT('Ctrl Pts',(-0.491705584034995,-0.633577589952803,
-1.74409145569984));
#49429=CARTESIAN_POINT('Ctrl Pts',(-0.378009890139618,-0.707321332081983,
-1.73880561884119));
#49430=CARTESIAN_POINT('Ctrl Pts',(-0.253605456630702,-0.749420075116088,
-1.73351978198254));
#49431=CARTESIAN_POINT('Ctrl Pts',(-0.129201023121776,-0.791518818150198,
-1.72823394512389));
#49432=CARTESIAN_POINT('Ctrl Pts',(0.005912150000697,-0.801972562089233,
-1.72294810826524));
#49433=CARTESIAN_POINT('Ctrl Pts',(0.135311655504476,-0.779510700699169,
-1.7176622714066));
#49434=CARTESIAN_POINT('Ctrl Pts',(0.264711161008255,-0.757048839309105,
-1.71237643454795));
#49435=CARTESIAN_POINT('Ctrl Pts',(0.388396998893335,-0.701671372589941,
-1.7070905976893));
#49436=CARTESIAN_POINT('Ctrl Pts',(0.491335703867856,-0.620109186131402,
-1.70180476083066));
#49437=CARTESIAN_POINT('Ctrl Pts',(0.594274408842377,-0.538546999672864,
-1.69651892397201));
#49438=CARTESIAN_POINT('Ctrl Pts',(0.676465980906336,-0.430800093474953,
-1.69123308711336));
#49439=CARTESIAN_POINT('Ctrl Pts',(0.727920398833092,-0.309964626340722,
-1.68594725025471));
#49440=CARTESIAN_POINT('Ctrl Pts',(0.779374816759847,-0.189129159206491,
-1.68066141339606));
#49441=CARTESIAN_POINT('Ctrl Pts',(0.800092080549398,-0.0552051311359448,
-1.67537557653742));
#49442=CARTESIAN_POINT('Ctrl Pts',(0.787554098628381,0.0755295859482219,
-1.67008973967877));
#49443=CARTESIAN_POINT('Ctrl Pts',(0.775016116707365,0.206264303032389,
-1.66480390282012));
#49444=CARTESIAN_POINT('Ctrl Pts',(0.729222889075781,0.333809709130172,
-1.65951806596147));
#49445=CARTESIAN_POINT('Ctrl Pts',(0.655740379549484,0.44266322554304,-1.65423222910282));
#49446=CARTESIAN_POINT('Ctrl Pts',(0.582257870023187,0.551516741955908,
-1.64894639224418));
#49447=CARTESIAN_POINT('Ctrl Pts',(0.481086078602161,0.641678368683872,
-1.64366055538553));
#49448=CARTESIAN_POINT('Ctrl Pts',(0.364521988036041,0.702189359687345,
-1.63837471852688));
#49449=CARTESIAN_POINT('Ctrl Pts',(0.247957897469928,0.762700350690814,
-1.63308888166823));
#49450=CARTESIAN_POINT('Ctrl Pts',(0.116001507758712,0.79356070596981,-1.62780304480958));
#49451=CARTESIAN_POINT('Ctrl Pts',(-0.015308466894889,0.791019486145062,
-1.62251720795094));
#49452=CARTESIAN_POINT('Ctrl Pts',(-0.146618441548498,0.788478266320315,
-1.61723137109229));
#49453=CARTESIAN_POINT('Ctrl Pts',(-0.277282001144486,0.752535471391821,
-1.61194553423364));
#49454=CARTESIAN_POINT('Ctrl Pts',(-0.391417569249487,0.687559788747637,
-1.60665969737499));
#49455=CARTESIAN_POINT('Ctrl Pts',(-0.505553137354487,0.622584106103453,
-1.60137386051635));
#49456=CARTESIAN_POINT('Ctrl Pts',(-0.603160713968495,0.528575535743582,
-1.5960880236577));
#49457=CARTESIAN_POINT('Ctrl Pts',(-0.672376530851428,0.416960402652422,
-1.59080218679905));
#49458=CARTESIAN_POINT('Ctrl Pts',(-0.74159234773436,0.305345269561261,
-1.5855163499404));
#49459=CARTESIAN_POINT('Ctrl Pts',(-0.782416404886214,0.176123573738817,
-1.58023051308176));
#49460=CARTESIAN_POINT('Ctrl Pts',(-0.789886719134465,0.0450016394686068,
-1.57494467622311));
#49461=CARTESIAN_POINT('Ctrl Pts',(-0.790740110588152,0.0300225724068191,
-1.5743408344233));
#49462=CARTESIAN_POINT('Ctrl Pts',(-0.791158227354029,0.0150187067579734,
-1.5737369926235));
#49463=CARTESIAN_POINT('Ctrl Pts',(-0.791145759608552,1.41466495050277E-5,
-1.5731331508237));
#49464=CARTESIAN_POINT('Origin',(0.,0.,-2.94));
#49465=CARTESIAN_POINT('',(-0.791067994997204,-1.8415035504149E-5,-1.3446668491763));
#49466=CARTESIAN_POINT('',(-0.791082733992286,-2.00018711214563E-5,-1.3731331508237));
#49467=CARTESIAN_POINT('',(-0.7911,-9.68818082805471E-17,-2.94));
#49468=CARTESIAN_POINT('Ctrl Pts',(-0.791067994997204,-1.8415035504149E-5,
-1.3446668491763));
#49469=CARTESIAN_POINT('Ctrl Pts',(-0.790990174960068,0.0902196588333193,
-1.348297351668));
#49470=CARTESIAN_POINT('Ctrl Pts',(-0.775570000219954,0.180483650617083,
-1.35192785415971));
#49471=CARTESIAN_POINT('Ctrl Pts',(-0.745303502796337,0.265459728452642,
-1.35555835665142));
#49472=CARTESIAN_POINT('Ctrl Pts',(-0.701236939550792,0.389180807105671,
-1.36084419351007));
#49473=CARTESIAN_POINT('Ctrl Pts',(-0.625699203521556,0.50169258786878,
-1.36613003036871));
#49474=CARTESIAN_POINT('Ctrl Pts',(-0.527871571661909,0.589319762558348,
-1.37141586722736));
#49475=CARTESIAN_POINT('Ctrl Pts',(-0.430043939802261,0.676946937247915,
-1.37670170408601));
#49476=CARTESIAN_POINT('Ctrl Pts',(-0.309926412112203,0.73968950586394,
-1.38198754094466));
#49477=CARTESIAN_POINT('Ctrl Pts',(-0.18211874159782,0.769921387330854,
-1.3872733778033));
#49478=CARTESIAN_POINT('Ctrl Pts',(-0.0543110710834368,0.800153268797768,
-1.39255921466195));
#49479=CARTESIAN_POINT('Ctrl Pts',(0.0811867422552711,0.79787446311557,
-1.3978450515206));
#49480=CARTESIAN_POINT('Ctrl Pts',(0.207905539872897,0.763361949012918,
-1.40313088837925));
#49481=CARTESIAN_POINT('Ctrl Pts',(0.334624337490523,0.728849434910265,
-1.4084167252379));
#49482=CARTESIAN_POINT('Ctrl Pts',(0.452564119387066,0.662103212387157,
-1.41370256209654));
#49483=CARTESIAN_POINT('Ctrl Pts',(0.547389827903631,0.57123598890325,-1.41898839895519));
#49484=CARTESIAN_POINT('Ctrl Pts',(0.642215536420195,0.480368765419343,
-1.42427423581384));
#49485=CARTESIAN_POINT('Ctrl Pts',(0.71392717155678,0.365380540974639,-1.42956007267249));
#49486=CARTESIAN_POINT('Ctrl Pts',(0.753808501962385,0.240247624504105,
-1.43484590953113));
#49487=CARTESIAN_POINT('Ctrl Pts',(0.793689832367991,0.115114708033571,
-1.44013174638978));
#49488=CARTESIAN_POINT('Ctrl Pts',(0.801740858042617,-0.0201629004627912,
-1.44541758324843));
#49489=CARTESIAN_POINT('Ctrl Pts',(0.776983012505953,-0.149142807361987,
-1.45070342010708));
#49490=CARTESIAN_POINT('Ctrl Pts',(0.75222516696929,-0.278122714261184,
-1.45598925696573));
#49491=CARTESIAN_POINT('Ctrl Pts',(0.694658450221336,-0.400804919563214,
-1.46127509382437));
#49492=CARTESIAN_POINT('Ctrl Pts',(0.611279841487808,-0.502277945067551,
-1.46656093068302));
#49493=CARTESIAN_POINT('Ctrl Pts',(0.527901232754279,-0.603750970571887,
-1.47184676754167));
#49494=CARTESIAN_POINT('Ctrl Pts',(0.418710732035175,-0.68401481627853,
-1.47713260440032));
#49495=CARTESIAN_POINT('Ctrl Pts',(0.296979960648103,-0.733313767553898,
-1.48241844125897));
#49496=CARTESIAN_POINT('Ctrl Pts',(0.175249189261031,-0.782612718829265,
-1.48770427811761));
#49497=CARTESIAN_POINT('Ctrl Pts',(0.0409781472059913,-0.800946775673357,
-1.49299011497626));
#49498=CARTESIAN_POINT('Ctrl Pts',(-0.0895131155828244,-0.786087514752204,
-1.49827595183491));
#49499=CARTESIAN_POINT('Ctrl Pts',(-0.22000437837164,-0.771228253831051,
-1.50356178869356));
#49500=CARTESIAN_POINT('Ctrl Pts',(-0.346715861894232,-0.723175675144652,
-1.5088476255522));
#49501=CARTESIAN_POINT('Ctrl Pts',(-0.454246347044275,-0.647770356613803,
-1.51413346241085));
#49502=CARTESIAN_POINT('Ctrl Pts',(-0.561776832194319,-0.572365038082953,
-1.5194192992695));
#49503=CARTESIAN_POINT('Ctrl Pts',(-0.650126318971814,-0.469606979707652,
-1.52470513612815));
#49504=CARTESIAN_POINT('Ctrl Pts',(-0.708556318914909,-0.351985967953831,
-1.5299909729868));
#49505=CARTESIAN_POINT('Ctrl Pts',(-0.762632363248006,-0.243129574794532,
-1.53488293171663));
#49506=CARTESIAN_POINT('Ctrl Pts',(-0.791081736219983,-0.121542748663734,
-1.53977489044646));
#49507=CARTESIAN_POINT('Ctrl Pts',(-0.791157484722713,9.84224722326565E-6,
-1.54466684917629));
#49508=CARTESIAN_POINT('Ctrl Pts',(-0.791145759608552,1.41466495050277E-5,
-1.5731331508237));
#49509=CARTESIAN_POINT('Ctrl Pts',(-0.791049088721019,-0.116326385441727,
-1.56845115576485));
#49510=CARTESIAN_POINT('Ctrl Pts',(-0.765065880610099,-0.232708668117082,
-1.56376916070601));
#49511=CARTESIAN_POINT('Ctrl Pts',(-0.715382449179442,-0.337896623282764,
-1.55908716564716));
#49512=CARTESIAN_POINT('Ctrl Pts',(-0.659291293631521,-0.456650779045952,
-1.55380132878851));
#49513=CARTESIAN_POINT('Ctrl Pts',(-0.572992411191032,-0.561136917854358,
-1.54851549192987));
#49514=CARTESIAN_POINT('Ctrl Pts',(-0.466975048453054,-0.638655212726037,
-1.54322965507122));
#49515=CARTESIAN_POINT('Ctrl Pts',(-0.360957685715075,-0.716173507597717,
-1.53794381821257));
#49516=CARTESIAN_POINT('Ctrl Pts',(-0.235221842679609,-0.766723958532671,
-1.53265798135392));
#49517=CARTESIAN_POINT('Ctrl Pts',(-0.105050153676812,-0.784162382311437,
-1.52737214449528));
#49518=CARTESIAN_POINT('Ctrl Pts',(0.0251215353259854,-0.801600806090204,
-1.52208630763663));
#49519=CARTESIAN_POINT('Ctrl Pts',(0.159729070296112,-0.785927202712783,
-1.51680047077798));
#49520=CARTESIAN_POINT('Ctrl Pts',(0.282411502077233,-0.73904662918814,
-1.51151463391933));
#49521=CARTESIAN_POINT('Ctrl Pts',(0.405093933858354,-0.692166055663498,
-1.50622879706069));
#49522=CARTESIAN_POINT('Ctrl Pts',(0.515851262450468,-0.614078511991633,
-1.50094296020204));
#49523=CARTESIAN_POINT('Ctrl Pts',(0.601221425553798,-0.514275192941416,
-1.49565712334339));
#49524=CARTESIAN_POINT('Ctrl Pts',(0.686591588657128,-0.414471873891198,
-1.49037128648474));
#49525=CARTESIAN_POINT('Ctrl Pts',(0.746574586271674,-0.292952779462627,
-1.48508544962609));
#49526=CARTESIAN_POINT('Ctrl Pts',(0.773879750943835,-0.164488016885666,
-1.47979961276745));
#49527=CARTESIAN_POINT('Ctrl Pts',(0.801184915615994,-0.0360232543087124,
-1.4745137759088));
#49528=CARTESIAN_POINT('Ctrl Pts',(0.795812247345771,0.0993871764166298,
-1.46922793905015));
#49529=CARTESIAN_POINT('Ctrl Pts',(0.758414770144211,0.22528473771424,-1.4639421021915));
#49530=CARTESIAN_POINT('Ctrl Pts',(0.721017292942649,0.351182299011858,
-1.45865626533285));
#49531=CARTESIAN_POINT('Ctrl Pts',(0.651595006809745,0.467566990881743,
-1.45337042847421));
#49532=CARTESIAN_POINT('Ctrl Pts',(0.558585882873856,0.560292769963976,
-1.44808459161556));
#49533=CARTESIAN_POINT('Ctrl Pts',(0.465576758937968,0.65301854904621,-1.44279875475691));
#49534=CARTESIAN_POINT('Ctrl Pts',(0.348980797199094,0.722085415340792,
-1.43751291789827));
#49535=CARTESIAN_POINT('Ctrl Pts',(0.222969719933163,0.759098597425129,
-1.43222708103962));
#49536=CARTESIAN_POINT('Ctrl Pts',(0.0969586426672318,0.796111779509465,
-1.42694124418097));
#49537=CARTESIAN_POINT('Ctrl Pts',(-0.0384675501257566,0.801071277383556,
-1.42165540732232));
#49538=CARTESIAN_POINT('Ctrl Pts',(-0.166848405060231,0.77337428606641,
-1.41636957046367));
#49539=CARTESIAN_POINT('Ctrl Pts',(-0.295229259994706,0.745677294749263,
-1.41108373360502));
#49540=CARTESIAN_POINT('Ctrl Pts',(-0.416564777070667,0.685323814240878,
-1.40579789674638));
#49541=CARTESIAN_POINT('Ctrl Pts',(-0.516107162071556,0.599649542548242,
-1.40051205988773));
#49542=CARTESIAN_POINT('Ctrl Pts',(-0.615649547072444,0.513975270855606,
-1.39522622302908));
#49543=CARTESIAN_POINT('Ctrl Pts',(-0.693398799998261,0.402980207978719,
-1.38994038617043));
#49544=CARTESIAN_POINT('Ctrl Pts',(-0.739904843820666,0.280155311765788,
-1.38465454931178));
#49545=CARTESIAN_POINT('Ctrl Pts',(-0.773694174145641,0.190915921588506,
-1.38081408314909));
#49546=CARTESIAN_POINT('Ctrl Pts',(-0.790990642988861,0.0954317246784125,
-1.37697361698639));
#49547=CARTESIAN_POINT('Ctrl Pts',(-0.791082733992286,-2.00018711214563E-5,
-1.3731331508237));
#49548=CARTESIAN_POINT('Origin',(0.,0.,-2.94));
#49549=CARTESIAN_POINT('',(-0.791073002592696,1.9102929482484E-5,-1.1446668491763));
#49550=CARTESIAN_POINT('',(-0.791059456711661,1.68138715613493E-5,-1.1731331508237));
#49551=CARTESIAN_POINT('',(-0.7911,-9.68818082805471E-17,-2.94));
#49552=CARTESIAN_POINT('Ctrl Pts',(-0.791073002592696,1.9102929482484E-5,
-1.1446668491763));
#49553=CARTESIAN_POINT('Ctrl Pts',(-0.791108504901705,0.0393221944095275,
-1.14624813917225));
#49554=CARTESIAN_POINT('Ctrl Pts',(-0.788231387404301,0.0786201345074876,
-1.1478294291682));
#49555=CARTESIAN_POINT('Ctrl Pts',(-0.782397600201548,0.117474141450363,
-1.14941071916415));
#49556=CARTESIAN_POINT('Ctrl Pts',(-0.762896782830441,0.247352874972065,
-1.1546965560228));
#49557=CARTESIAN_POINT('Ctrl Pts',(-0.710358457961914,0.372271147434174,
-1.15998239288145));
#49558=CARTESIAN_POINT('Ctrl Pts',(-0.631168426079748,0.477045696585406,
-1.1652682297401));
#49559=CARTESIAN_POINT('Ctrl Pts',(-0.551978394197586,0.581820245736633,
-1.17055406659874));
#49560=CARTESIAN_POINT('Ctrl Pts',(-0.446136655301788,0.666451071576987,
-1.17583990345739));
#49561=CARTESIAN_POINT('Ctrl Pts',(-0.326507803555503,0.72065167239659,
-1.18112574031604));
#49562=CARTESIAN_POINT('Ctrl Pts',(-0.206878951809204,0.774852273216199,
-1.18641157717469));
#49563=CARTESIAN_POINT('Ctrl Pts',(-0.0734629872124128,0.798622649015049,
-1.19169741403333));
#49564=CARTESIAN_POINT('Ctrl Pts',(0.0575239711751428,0.789073615989587,
-1.19698325089198));
#49565=CARTESIAN_POINT('Ctrl Pts',(0.188510929562691,0.779524582964126,
-1.20226908775063));
#49566=CARTESIAN_POINT('Ctrl Pts',(0.317068881741004,0.736656141114355,
-1.20755492460928));
#49567=CARTESIAN_POINT('Ctrl Pts',(0.427572178524106,0.665678759510014,
-1.21284076146793));
#49568=CARTESIAN_POINT('Ctrl Pts',(0.538075475307208,0.594701377905672,
-1.21812659832657));
#49569=CARTESIAN_POINT('Ctrl Pts',(0.6305241166951,0.49561505654676,-1.22341243518522));
#49570=CARTESIAN_POINT('Ctrl Pts',(0.693681380154711,0.380463298541787,
-1.22869827204387));
#49571=CARTESIAN_POINT('Ctrl Pts',(0.756838643614322,0.265311540536814,
-1.23398410890252));
#49572=CARTESIAN_POINT('Ctrl Pts',(0.790704529145653,0.13409434588578,-1.23926994576117));
#49573=CARTESIAN_POINT('Ctrl Pts',(0.791162788490867,0.00276058290871739,
-1.24455578261981));
#49574=CARTESIAN_POINT('Ctrl Pts',(0.791621047836082,-0.128573180068345,
-1.24984161947846));
#49575=CARTESIAN_POINT('Ctrl Pts',(0.75867168099518,-0.260023511371435,
-1.25512745633711));
#49576=CARTESIAN_POINT('Ctrl Pts',(0.696319537442132,-0.375613205953966,
-1.26041329319576));
#49577=CARTESIAN_POINT('Ctrl Pts',(0.633967393889087,-0.49120290053649,
-1.26569913005441));
#49578=CARTESIAN_POINT('Ctrl Pts',(0.542212473623899,-0.590931958398456,
-1.27098496691305));
#49579=CARTESIAN_POINT('Ctrl Pts',(0.432207180452458,-0.662678754658679,
-1.2762708037717));
#49580=CARTESIAN_POINT('Ctrl Pts',(0.322201887281011,-0.734425550918906,
-1.28155664063035));
#49581=CARTESIAN_POINT('Ctrl Pts',(0.193946221203308,-0.778190085577387,
-1.286842477489));
#49582=CARTESIAN_POINT('Ctrl Pts',(0.0630290898698403,-0.788652973455892,
-1.29212831434764));
#49583=CARTESIAN_POINT('Ctrl Pts',(-0.0678880414636275,-0.799115861334397,
-1.29741415120629));
#49584=CARTESIAN_POINT('Ctrl Pts',(-0.20146663805286,-0.776277102432927,
-1.30269998806494));
#49585=CARTESIAN_POINT('Ctrl Pts',(-0.321470813640404,-0.722912646651044,
-1.30798582492359));
#49586=CARTESIAN_POINT('Ctrl Pts',(-0.441474989227948,-0.669548190869161,
-1.31327166178223));
#49587=CARTESIAN_POINT('Ctrl Pts',(-0.547904743813803,-0.585658038206865,
-1.31855749864088));
#49588=CARTESIAN_POINT('Ctrl Pts',(-0.627824012534386,-0.48143866483267,
-1.32384333549953));
#49589=CARTESIAN_POINT('Ctrl Pts',(-0.707743281254969,-0.377219291458475,
-1.32912917235818));
#49590=CARTESIAN_POINT('Ctrl Pts',(-0.761152064110279,-0.25267069737238,
-1.33441500921682));
#49591=CARTESIAN_POINT('Ctrl Pts',(-0.781558760307008,-0.122931212057858,
-1.33970084607547));
#49592=CARTESIAN_POINT('Ctrl Pts',(-0.787949405049457,-0.0823014623070763,
-1.34135618044241));
#49593=CARTESIAN_POINT('Ctrl Pts',(-0.791103477187948,-0.041162632736165,
-1.34301151480935));
#49594=CARTESIAN_POINT('Ctrl Pts',(-0.791067994997204,-1.8415035504149E-5,
-1.3446668491763));
#49595=CARTESIAN_POINT('Ctrl Pts',(-0.791082733992286,-2.00018711214563E-5,
-1.3731331508237));
#49596=CARTESIAN_POINT('Ctrl Pts',(-0.791117392711325,-0.0359435389075563,
-1.37168778012775));
#49597=CARTESIAN_POINT('Ctrl Pts',(-0.788715197055925,-0.0718624767924898,
-1.3702424094318));
#49598=CARTESIAN_POINT('Ctrl Pts',(-0.783838218078167,-0.107442191432954,
-1.36879703873584));
#49599=CARTESIAN_POINT('Ctrl Pts',(-0.766002713794266,-0.23756006886979,
-1.36351120187719));
#49600=CARTESIAN_POINT('Ctrl Pts',(-0.715068870507469,-0.363141094194489,
-1.35822536501854));
#49601=CARTESIAN_POINT('Ctrl Pts',(-0.637227471078016,-0.468921450483326,
-1.3529395281599));
#49602=CARTESIAN_POINT('Ctrl Pts',(-0.559386071648563,-0.574701806772162,
-1.34765369130125));
#49603=CARTESIAN_POINT('Ctrl Pts',(-0.454637116076454,-0.660681494025135,
-1.3423678544426));
#49604=CARTESIAN_POINT('Ctrl Pts',(-0.335712375556184,-0.716410062407205,
-1.33708201758396));
#49605=CARTESIAN_POINT('Ctrl Pts',(-0.216787635035913,-0.772138630789275,
-1.33179618072531));
#49606=CARTESIAN_POINT('Ctrl Pts',(-0.0836871095674816,-0.797616080300441,
-1.32651034386666));
#49607=CARTESIAN_POINT('Ctrl Pts',(0.0474114220170869,-0.789745739894928,
-1.32122450700801));
#49608=CARTESIAN_POINT('Ctrl Pts',(0.178509953601655,-0.781875399489416,
-1.31593867014936));
#49609=CARTESIAN_POINT('Ctrl Pts',(0.307606491302361,-0.740657269167225,
-1.31065283329072));
#49610=CARTESIAN_POINT('Ctrl Pts',(0.419009923250545,-0.671101229947795,
-1.30536699643207));
#49611=CARTESIAN_POINT('Ctrl Pts',(0.53041335519873,-0.601545190728366,
-1.30008115957342));
#49612=CARTESIAN_POINT('Ctrl Pts',(0.624123681394395,-0.503651242611697,
-1.29479532271477));
#49613=CARTESIAN_POINT('Ctrl Pts',(0.688750827109173,-0.389317961024534,
-1.28950948585612));
#49614=CARTESIAN_POINT('Ctrl Pts',(0.753377972823951,-0.27498467943737,
-1.28422364899748));
#49615=CARTESIAN_POINT('Ctrl Pts',(0.788921938057842,-0.144212064379711,
-1.27893781213883));
#49616=CARTESIAN_POINT('Ctrl Pts',(0.791062511404142,-0.0128949474928493,
-1.27365197528018));
#49617=CARTESIAN_POINT('Ctrl Pts',(0.793203084750441,0.118422169394013,
-1.26836613842153));
#49618=CARTESIAN_POINT('Ctrl Pts',(0.761940266209149,0.250283788110078,
-1.26308030156288));
#49619=CARTESIAN_POINT('Ctrl Pts',(0.701073912784938,0.366662713446961,
-1.25779446470424));
#49620=CARTESIAN_POINT('Ctrl Pts',(0.640207559360726,0.483041638783844,
-1.25250862784559));
#49621=CARTESIAN_POINT('Ctrl Pts',(0.549737671053596,0.583937870741544,
-1.24722279098694));
#49622=CARTESIAN_POINT('Ctrl Pts',(0.440660461731521,0.657087919601657,
-1.24193695412829));
#49623=CARTESIAN_POINT('Ctrl Pts',(0.331583252409446,0.73023796846177,-1.23665111726965));
#49624=CARTESIAN_POINT('Ctrl Pts',(0.203898722072426,0.775641834224296,
-1.231365280411));
#49625=CARTESIAN_POINT('Ctrl Pts',(0.0731263593535346,0.787780878282514,
-1.22607944355235));
#49626=CARTESIAN_POINT('Ctrl Pts',(-0.0576460033653572,0.799919922340731,
-1.2207936066937));
#49627=CARTESIAN_POINT('Ctrl Pts',(-0.191506198466121,0.778794144694639,
-1.21550776983506));
#49628=CARTESIAN_POINT('Ctrl Pts',(-0.312184112640562,0.726971289965908,
-1.21022193297641));
#49629=CARTESIAN_POINT('Ctrl Pts',(-0.432862026814995,0.67514843523718,
-1.20493609611776));
#49630=CARTESIAN_POINT('Ctrl Pts',(-0.540357660063106,0.592628503425816,
-1.19965025925911));
#49631=CARTESIAN_POINT('Ctrl Pts',(-0.621605394694988,0.489441426430128,
-1.19436442240046));
#49632=CARTESIAN_POINT('Ctrl Pts',(-0.70285312932687,0.386254349434441,
-1.18907858554182));
#49633=CARTESIAN_POINT('Ctrl Pts',(-0.757852965342524,0.262400127254429,
-1.18379274868317));
#49634=CARTESIAN_POINT('Ctrl Pts',(-0.779919916490187,0.132932691546551,
-1.17850691182452));
#49635=CARTESIAN_POINT('Ctrl Pts',(-0.787397920109764,0.0890590296907594,
-1.17671565815758));
#49636=CARTESIAN_POINT('Ctrl Pts',(-0.791093967912682,0.0445407560544645,
-1.17492440449064));
#49637=CARTESIAN_POINT('Ctrl Pts',(-0.791059456711661,1.68138715613493E-5,
-1.1731331508237));
#49638=CARTESIAN_POINT('Origin',(0.,0.,-2.94));
#49639=CARTESIAN_POINT('',(-0.791153738188075,-1.14622333243219E-5,-0.944666849176297));
#49640=CARTESIAN_POINT('',(-0.791163026494784,-6.63049684663537E-6,-0.973133150823701));
#49641=CARTESIAN_POINT('',(-0.7911,-9.68818082805471E-17,-2.94));
#49642=CARTESIAN_POINT('Ctrl Pts',(-0.791153738188075,-1.14622333243219E-5,
-0.944666849176297));
#49643=CARTESIAN_POINT('Ctrl Pts',(-0.791069254281359,0.119702961705676,
-0.949484763535142));
#49644=CARTESIAN_POINT('Ctrl Pts',(-0.763503490006759,0.239454969527334,
-0.954302677893988));
#49645=CARTESIAN_POINT('Ctrl Pts',(-0.71099538606271,0.347032764603257,
-0.959120592252833));
#49646=CARTESIAN_POINT('Ctrl Pts',(-0.653387622509252,0.465058663785214,
-0.96440642911148));
#49647=CARTESIAN_POINT('Ctrl Pts',(-0.565757380114313,0.568430763467434,
-0.969692265970127));
#49648=CARTESIAN_POINT('Ctrl Pts',(-0.458755726373478,0.644584643185194,
-0.974978102828774));
#49649=CARTESIAN_POINT('Ctrl Pts',(-0.351754072632631,0.720738522902962,
-0.980263939687422));
#49650=CARTESIAN_POINT('Ctrl Pts',(-0.225381007545903,0.769674182656259,
-0.98554977654607));
#49651=CARTESIAN_POINT('Ctrl Pts',(-0.0949966169589208,0.785443709935347,
-0.990835613404718));
#49652=CARTESIAN_POINT('Ctrl Pts',(0.0353877736280465,0.801213237214434,
-0.996121450263366));
#49653=CARTESIAN_POINT('Ctrl Pts',(0.16978348971527,0.783816632019305,-1.00140728712201));
#49654=CARTESIAN_POINT('Ctrl Pts',(0.291855327792586,0.735368374591758,
-1.00669312398066));
#49655=CARTESIAN_POINT('Ctrl Pts',(0.413927165869916,0.686920117164204,
-1.01197896083931));
#49656=CARTESIAN_POINT('Ctrl Pts',(0.523675125937363,0.607420207504222,
-1.01726479769796));
#49657=CARTESIAN_POINT('Ctrl Pts',(0.607759829964756,0.506531507205476,
-1.02255063455661));
#49658=CARTESIAN_POINT('Ctrl Pts',(0.691844533992139,0.405642806906743,
-1.02783647141525));
#49659=CARTESIAN_POINT('Ctrl Pts',(0.750265981979478,0.283365315969246,
-1.0331223082739));
#49660=CARTESIAN_POINT('Ctrl Pts',(0.775923305907959,0.15456132135662,-1.03840814513255));
#49661=CARTESIAN_POINT('Ctrl Pts',(0.801580629836442,0.0257573267439869,
-1.0436939819912));
#49662=CARTESIAN_POINT('Ctrl Pts',(0.794473829706067,-0.10957317154376,
-1.04897981884984));
#49663=CARTESIAN_POINT('Ctrl Pts',(0.75546670556802,-0.234981351363983,
-1.05426565570849));
#49664=CARTESIAN_POINT('Ctrl Pts',(0.716459581429971,-0.360389531184213,
-1.05955149256714));
#49665=CARTESIAN_POINT('Ctrl Pts',(0.645552133284242,-0.4758753925369,-1.06483732942579));
#49666=CARTESIAN_POINT('Ctrl Pts',(0.551362847118086,-0.567402140926943,
-1.07012316628444));
#49667=CARTESIAN_POINT('Ctrl Pts',(0.457173560951941,-0.658928889316976,
-1.07540900314308));
#49668=CARTESIAN_POINT('Ctrl Pts',(0.339702436765368,-0.726496524744374,
-1.08069484000173));
#49669=CARTESIAN_POINT('Ctrl Pts',(0.213227568950196,-0.76189250065231,
-1.08598067686038));
#49670=CARTESIAN_POINT('Ctrl Pts',(0.0867527011350093,-0.797288476560251,
-1.09126651371903));
#49671=CARTESIAN_POINT('Ctrl Pts',(-0.0487259103087836,-0.800512792948724,
-1.09655235057767));
#49672=CARTESIAN_POINT('Ctrl Pts',(-0.176741440740974,-0.771173548454202,
-1.10183818743632));
#49673=CARTESIAN_POINT('Ctrl Pts',(-0.304756971173165,-0.741834303959681,
-1.10712402429497));
#49674=CARTESIAN_POINT('Ctrl Pts',(-0.425309420593757,-0.679931498582165,
-1.11240986115362));
#49675=CARTESIAN_POINT('Ctrl Pts',(-0.523746173188335,-0.592989143898281,
-1.11769569801227));
#49676=CARTESIAN_POINT('Ctrl Pts',(-0.622182925782902,-0.506046789214406,
-1.12298153487091));
#49677=CARTESIAN_POINT('Ctrl Pts',(-0.698503981551462,-0.394064885224168,
-1.12826737172956));
#49678=CARTESIAN_POINT('Ctrl Pts',(-0.7434328544989,-0.270654335938406,
-1.13355320858821));
#49679=CARTESIAN_POINT('Ctrl Pts',(-0.774920983961236,-0.184162797246254,
-1.1372577554509));
#49680=CARTESIAN_POINT('Ctrl Pts',(-0.790989830013477,-0.0920577106906312,
-1.1409623023136));
#49681=CARTESIAN_POINT('Ctrl Pts',(-0.791073002592696,1.9102929482484E-5,
-1.1446668491763));
#49682=CARTESIAN_POINT('Ctrl Pts',(-0.791059456711661,1.68138715613493E-5,
-1.1731331508237));
#49683=CARTESIAN_POINT('Ctrl Pts',(-0.790992128300705,-0.0868456014593881,
-1.16963856763199));
#49684=CARTESIAN_POINT('Ctrl Pts',(-0.776726037359125,-0.173729591666139,
-1.16614398444028));
#49685=CARTESIAN_POINT('Ctrl Pts',(-0.748642821403881,-0.255890802062731,
-1.16264940124858));
#49686=CARTESIAN_POINT('Ctrl Pts',(-0.706164708890245,-0.380166210728354,
-1.15736356438993));
#49687=CARTESIAN_POINT('Ctrl Pts',(-0.632074417583308,-0.493636378823848,
-1.15207772753128));
#49688=CARTESIAN_POINT('Ctrl Pts',(-0.53537729394692,-0.582509510433902,
-1.14679189067263));
#49689=CARTESIAN_POINT('Ctrl Pts',(-0.438680170310532,-0.671382642043956,
-1.14150605381399));
#49690=CARTESIAN_POINT('Ctrl Pts',(-0.319376214344695,-0.735658737168568,
-1.13622021695534));
#49691=CARTESIAN_POINT('Ctrl Pts',(-0.191966293019002,-0.76752532138322,
-1.13093438009669));
#49692=CARTESIAN_POINT('Ctrl Pts',(-0.0645563716933151,-0.79939190559787,
-1.12564854323804));
#49693=CARTESIAN_POINT('Ctrl Pts',(0.0709595149922231,-0.798848978902562,
-1.1203627063794));
#49694=CARTESIAN_POINT('Ctrl Pts',(0.198110011757025,-0.765962531630302,
-1.11507686952075));
#49695=CARTESIAN_POINT('Ctrl Pts',(0.325260508521841,-0.733076084358039,
-1.1097910326621));
#49696=CARTESIAN_POINT('Ctrl Pts',(0.444045615365914,-0.667846116508817,
-1.10450519580345));
#49697=CARTESIAN_POINT('Ctrl Pts',(0.540027529130329,-0.578201041508283,
-1.0992193589448));
#49698=CARTESIAN_POINT('Ctrl Pts',(0.636009442894732,-0.488555966507759,
-1.09393352208616));
#49699=CARTESIAN_POINT('Ctrl Pts',(0.709188163579479,-0.374495784355932,
-1.08864768522751));
#49700=CARTESIAN_POINT('Ctrl Pts',(0.750669142088827,-0.249884004561106,
-1.08336184836886));
#49701=CARTESIAN_POINT('Ctrl Pts',(0.792150120598178,-0.125272224766274,
-1.07807601151021));
#49702=CARTESIAN_POINT('Ctrl Pts',(0.801933356932126,0.00989115267157506,
-1.07279017465157));
#49703=CARTESIAN_POINT('Ctrl Pts',(0.778829742083658,0.139177618408181,
-1.06750433779292));
#49704=CARTESIAN_POINT('Ctrl Pts',(0.75572612723519,0.268464084144795,-1.06221850093427));
#49705=CARTESIAN_POINT('Ctrl Pts',(0.699735661204308,0.391873638180182,
-1.05693266407562));
#49706=CARTESIAN_POINT('Ctrl Pts',(0.617663736929631,0.494406396299637,
-1.05164682721697));
#49707=CARTESIAN_POINT('Ctrl Pts',(0.535591812654964,0.596939154419081,
-1.04636099035832));
#49708=CARTESIAN_POINT('Ctrl Pts',(0.427438430136513,0.678595116622594,
-1.04107515349968));
#49709=CARTESIAN_POINT('Ctrl Pts',(0.306349153572166,0.729449362687698,
-1.03578931664103));
#49710=CARTESIAN_POINT('Ctrl Pts',(0.185259877007812,0.780303608752805,
-1.03050347978238));
#49711=CARTESIAN_POINT('Ctrl Pts',(0.0512347063975671,0.800356138679497,
-1.02521764292373));
#49712=CARTESIAN_POINT('Ctrl Pts',(-0.0794361929085426,0.78716965634866,
-1.01993180606509));
#49713=CARTESIAN_POINT('Ctrl Pts',(-0.210107092214652,0.773983174017823,
-1.01464596920644));
#49714=CARTESIAN_POINT('Ctrl Pts',(-0.337423720216622,0.727557679429456,
-1.00936013234779));
#49715=CARTESIAN_POINT('Ctrl Pts',(-0.445911305179286,0.653535985645149,
-1.00407429548914));
#49716=CARTESIAN_POINT('Ctrl Pts',(-0.55439889014195,0.579514291860843,
-0.998788458630495));
#49717=CARTESIAN_POINT('Ctrl Pts',(-0.644057432065305,0.477896398880599,
-0.993502621771847));
#49718=CARTESIAN_POINT('Ctrl Pts',(-0.703989332637604,0.361033511120964,
-0.988216784913199));
#49719=CARTESIAN_POINT('Ctrl Pts',(-0.760996443192033,0.249873753152225,
-0.983188906883366));
#49720=CARTESIAN_POINT('Ctrl Pts',(-0.791107547260317,0.124920661667419,
-0.978161028853534));
#49721=CARTESIAN_POINT('Ctrl Pts',(-0.791163026494784,-6.63049684663537E-6,
-0.973133150823701));
#49722=CARTESIAN_POINT('Origin',(0.,0.,-2.94));
#49723=CARTESIAN_POINT('',(-0.79103327968755,-2.89210560314168E-6,-0.744666849176298));
#49724=CARTESIAN_POINT('',(-0.791037024154788,-7.56658461008487E-6,-0.7731331508237));
#49725=CARTESIAN_POINT('',(-0.7911,-9.68818082805471E-17,-2.94));
#49726=CARTESIAN_POINT('Ctrl Pts',(-0.79103327968755,-2.89210560314168E-6,
-0.744666849176298));
#49727=CARTESIAN_POINT('Ctrl Pts',(-0.791024492119856,0.0688233200155534,
-0.747435551039388));
#49728=CARTESIAN_POINT('Ctrl Pts',(-0.782132078258211,0.137651760409329,
-0.750204252902477));
#49729=CARTESIAN_POINT('Ctrl Pts',(-0.764384099192582,0.204115476170194,
-0.752972954765567));
#49730=CARTESIAN_POINT('Ctrl Pts',(-0.730500739209966,0.331003951673808,
-0.758258791624215));
#49731=CARTESIAN_POINT('Ctrl Pts',(-0.664340509511136,0.449273450620519,
-0.763544628482863));
#49732=CARTESIAN_POINT('Ctrl Pts',(-0.573944892725679,0.544548839705632,
-0.76883046534151));
#49733=CARTESIAN_POINT('Ctrl Pts',(-0.483549275940222,0.639824228790745,
-0.774116302200158));
#49734=CARTESIAN_POINT('Ctrl Pts',(-0.368918272068141,0.712105508014256,
-0.779402139058806));
#49735=CARTESIAN_POINT('Ctrl Pts',(-0.24398477146737,0.752607208311651,
-0.784687975917454));
#49736=CARTESIAN_POINT('Ctrl Pts',(-0.119051270866599,0.793108908609046,
-0.789973812776101));
#49737=CARTESIAN_POINT('Ctrl Pts',(0.0161847264628582,0.801831029980324,
-0.79525964963475));
#49738=CARTESIAN_POINT('Ctrl Pts',(0.145285884550884,0.777713437238234,
-0.800545486493398));
#49739=CARTESIAN_POINT('Ctrl Pts',(0.274387042638903,0.753595844496146,
-0.805831323352045));
#49740=CARTESIAN_POINT('Ctrl Pts',(0.397353361485488,0.696638537640694,
-0.811117160210692));
#49741=CARTESIAN_POINT('Ctrl Pts',(0.49923883014826,0.61376442482669,-0.816402997069339));
#49742=CARTESIAN_POINT('Ctrl Pts',(0.601124298811043,0.530890312012677,
-0.821688833927988));
#49743=CARTESIAN_POINT('Ctrl Pts',(0.681928917290005,0.422099393240108,
-0.826974670786636));
#49744=CARTESIAN_POINT('Ctrl Pts',(0.731831242418353,0.300614722412347,
-0.832260507645284));
#49745=CARTESIAN_POINT('Ctrl Pts',(0.781733567546697,0.179130051584592,
-0.837546344503932));
#49746=CARTESIAN_POINT('Ctrl Pts',(0.800733599324429,0.0449516287016287,
-0.84283218136258));
#49747=CARTESIAN_POINT('Ctrl Pts',(0.786521968116677,-0.0856117537520969,
-0.848118018221228));
#49748=CARTESIAN_POINT('Ctrl Pts',(0.772310336908926,-0.216175136205815,
-0.853403855079876));
#49749=CARTESIAN_POINT('Ctrl Pts',(0.724887042715701,-0.343123478230312,
-0.858689691938524));
#49750=CARTESIAN_POINT('Ctrl Pts',(0.650016176717285,-0.451026771618364,
-0.863975528797172));
#49751=CARTESIAN_POINT('Ctrl Pts',(0.575145310718861,-0.558930065006429,
-0.86926136565582));
#49752=CARTESIAN_POINT('Ctrl Pts',(0.472826872915242,-0.647788309758041,
-0.874547202514467));
#49753=CARTESIAN_POINT('Ctrl Pts',(0.355497215840721,-0.706801180134935,
-0.879833039373115));
#49754=CARTESIAN_POINT('Ctrl Pts',(0.238167558766213,-0.765814050511822,
-0.885118876231763));
#49755=CARTESIAN_POINT('Ctrl Pts',(0.105826682420811,-0.794981546513998,
-0.89040471309041));
#49756=CARTESIAN_POINT('Ctrl Pts',(-0.0254399663468239,-0.79075848830279,
-0.895690549949058));
#49757=CARTESIAN_POINT('Ctrl Pts',(-0.156706615114466,-0.786535430091583,
-0.900976386807706));
#49758=CARTESIAN_POINT('Ctrl Pts',(-0.286899036304337,-0.748921817666989,
-0.906262223666354));
#49759=CARTESIAN_POINT('Ctrl Pts',(-0.40019291826776,-0.682489418876934,
-0.911548060525002));
#49760=CARTESIAN_POINT('Ctrl Pts',(-0.513486800231182,-0.616057020086879,
-0.916833897383649));
#49761=CARTESIAN_POINT('Ctrl Pts',(-0.609882142968154,-0.520805834931365,
-0.922119734242297));
#49762=CARTESIAN_POINT('Ctrl Pts',(-0.677662519892473,-0.408313222714652,
-0.927405571100945));
#49763=CARTESIAN_POINT('Ctrl Pts',(-0.745442896816793,-0.295820610497938,
-0.932691407959593));
#49764=CARTESIAN_POINT('Ctrl Pts',(-0.784608307928459,-0.166086571220027,
-0.93797724481824));
#49765=CARTESIAN_POINT('Ctrl Pts',(-0.790398371128303,-0.0348797022402185,
-0.943263081676888));
#49766=CARTESIAN_POINT('Ctrl Pts',(-0.790910929672757,-0.0232647682636074,
-0.943731004176691));
#49767=CARTESIAN_POINT('Ctrl Pts',(-0.791161943381833,-0.0116382925046326,
-0.944198926676494));
#49768=CARTESIAN_POINT('Ctrl Pts',(-0.791153738188075,-1.14622333243219E-5,
-0.944666849176297));
#49769=CARTESIAN_POINT('Ctrl Pts',(-0.791163026494784,-6.63049684663537E-6,
-0.973133150823701));
#49770=CARTESIAN_POINT('Ctrl Pts',(-0.791165872896041,-0.0064161133407936,
-0.972875191994886));
#49771=CARTESIAN_POINT('Ctrl Pts',(-0.791089604615324,-0.0128255282738238,
-0.972617233166071));
#49772=CARTESIAN_POINT('Ctrl Pts',(-0.790933794943816,-0.0192330090117345,
-0.972359274337257));
#49773=CARTESIAN_POINT('Ctrl Pts',(-0.787741097456487,-0.150528758845775,
-0.967073437478609));
#49774=CARTESIAN_POINT('Ctrl Pts',(-0.751150443260588,-0.281012375974835,
-0.96178760061996));
#49775=CARTESIAN_POINT('Ctrl Pts',(-0.685609264166152,-0.394824155174704,
-0.956501763761312));
#49776=CARTESIAN_POINT('Ctrl Pts',(-0.620068085071716,-0.508635934374572,
-0.951215926902664));
#49777=CARTESIAN_POINT('Ctrl Pts',(-0.525576381078742,-0.605775875645253,
-0.945930090044017));
#49778=CARTESIAN_POINT('Ctrl Pts',(-0.41361919992299,-0.674437049749595,
-0.94064425318537));
#49779=CARTESIAN_POINT('Ctrl Pts',(-0.301662018767232,-0.74309822385394,
-0.935358416326722));
#49780=CARTESIAN_POINT('Ctrl Pts',(-0.17223936044869,-0.783280630791945,
-0.930072579468073));
#49781=CARTESIAN_POINT('Ctrl Pts',(-0.0410819753514236,-0.790100277130122,
-0.924786742609425));
#49782=CARTESIAN_POINT('Ctrl Pts',(0.090075409745828,-0.796919923468298,
-0.919500905750777));
#49783=CARTESIAN_POINT('Ctrl Pts',(0.222967521621809,-0.770376809206654,
-0.914215068892129));
#49784=CARTESIAN_POINT('Ctrl Pts',(0.341441913192751,-0.713697132217263,
-0.908929232033482));
#49785=CARTESIAN_POINT('Ctrl Pts',(0.459916304763692,-0.657017455227872,
-0.903643395174834));
#49786=CARTESIAN_POINT('Ctrl Pts',(0.563972976029599,-0.570201215510731,
-0.898357558316188));
#49787=CARTESIAN_POINT('Ctrl Pts',(0.640964299884474,-0.46380054214444,
-0.89307172145754));
#49788=CARTESIAN_POINT('Ctrl Pts',(0.717955623739359,-0.357399868778137,
-0.887785884598892));
#49789=CARTESIAN_POINT('Ctrl Pts',(0.767881600183203,-0.231414761762697,
-0.882500047740244));
#49790=CARTESIAN_POINT('Ctrl Pts',(0.784673948102637,-0.101158152360013,
-0.877214210881596));
#49791=CARTESIAN_POINT('Ctrl Pts',(0.80146629602207,0.0290984570426636,
-0.871928374022948));
#49792=CARTESIAN_POINT('Ctrl Pts',(0.785125015417087,0.163626568832565,
-0.8666425371643));
#49793=CARTESIAN_POINT('Ctrl Pts',(0.737636316503833,0.286074887388823,
-0.861356700305653));
#49794=CARTESIAN_POINT('Ctrl Pts',(0.690147617590579,0.408523205945081,
-0.856070863447005));
#49795=CARTESIAN_POINT('Ctrl Pts',(0.611511500369052,0.518891731267699,
-0.850785026588357));
#49796=CARTESIAN_POINT('Ctrl Pts',(0.511285836291241,0.603765658370727,
-0.845499189729709));
#49797=CARTESIAN_POINT('Ctrl Pts',(0.411060172213435,0.68863958547375,-0.840213352871062));
#49798=CARTESIAN_POINT('Ctrl Pts',(0.289244961279322,0.748018914357198,
-0.834927516012414));
#49799=CARTESIAN_POINT('Ctrl Pts',(0.160646302367462,0.774686350825631,
-0.829641679153766));
#49800=CARTESIAN_POINT('Ctrl Pts',(0.0320476434555805,0.801353787294069,
-0.824355842295117));
#49801=CARTESIAN_POINT('Ctrl Pts',(-0.103334463434049,0.795309331347496,
-0.819070005436469));
#49802=CARTESIAN_POINT('Ctrl Pts',(-0.229044923362013,0.75728765981096,
-0.813784168577821));
#49803=CARTESIAN_POINT('Ctrl Pts',(-0.354755383289956,0.719265988274431,
-0.808498331719173));
#49804=CARTESIAN_POINT('Ctrl Pts',(-0.470794196256217,0.649267101147948,
-0.803212494860526));
#49805=CARTESIAN_POINT('Ctrl Pts',(-0.56305735894832,0.555799052854549,
-0.797926658001879));
#49806=CARTESIAN_POINT('Ctrl Pts',(-0.655320521640422,0.46233100456115,
-0.792640821143232));
#49807=CARTESIAN_POINT('Ctrl Pts',(-0.723808034058369,0.345393795100832,
-0.787354984284584));
#49808=CARTESIAN_POINT('Ctrl Pts',(-0.760195542674977,0.219200623897304,
-0.782069147425936));
#49809=CARTESIAN_POINT('Ctrl Pts',(-0.78070056783669,0.148088468953461,
-0.779090481891858));
#49810=CARTESIAN_POINT('Ctrl Pts',(-0.791012146346498,0.074037057278515,
-0.776111816357779));
#49811=CARTESIAN_POINT('Ctrl Pts',(-0.791037024154788,-7.56658461008487E-6,
-0.7731331508237));
#49812=CARTESIAN_POINT('Origin',(0.,0.,-2.94));
#49813=CARTESIAN_POINT('',(-0.791138066768001,1.60959521169762E-5,-0.544666849176297));
#49814=CARTESIAN_POINT('',(-0.791122640286116,1.87499586476574E-5,-0.573133150823702));
#49815=CARTESIAN_POINT('',(-0.7911,-9.68818082805471E-17,-2.94));
#49816=CARTESIAN_POINT('Ctrl Pts',(-0.791138066768001,1.60959521169762E-5,
-0.544666849176297));
#49817=CARTESIAN_POINT('Ctrl Pts',(-0.791154370742701,0.0178948272985896,
-0.545386338543632));
#49818=CARTESIAN_POINT('Ctrl Pts',(-0.790560616501651,0.03577247744017,
-0.546105827910967));
#49819=CARTESIAN_POINT('Ctrl Pts',(-0.789349314925486,0.0536081872233632,
-0.546825317278302));
#49820=CARTESIAN_POINT('Ctrl Pts',(-0.780450305699053,0.184640911892175,
-0.55211115413695));
#49821=CARTESIAN_POINT('Ctrl Pts',(-0.738220245989705,0.313409978176958,
-0.557396990995598));
#49822=CARTESIAN_POINT('Ctrl Pts',(-0.667792012348153,0.424264076908017,
-0.562682827854246));
#49823=CARTESIAN_POINT('Ctrl Pts',(-0.597363778706602,0.535118175639075,
-0.567968664712894));
#49824=CARTESIAN_POINT('Ctrl Pts',(-0.498737371132847,0.628057306816409,
-0.573254501571542));
#49825=CARTESIAN_POINT('Ctrl Pts',(-0.383900392253534,0.691785131047376,
-0.578540338430189));
#49826=CARTESIAN_POINT('Ctrl Pts',(-0.269063413374222,0.755512955278343,
-0.583826175288837));
#49827=CARTESIAN_POINT('Ctrl Pts',(-0.138015863189353,0.790029472562943,
-0.589112012147485));
#49828=CARTESIAN_POINT('Ctrl Pts',(-0.00668599048618175,0.791139353238011,
-0.594397849006133));
#49829=CARTESIAN_POINT('Ctrl Pts',(0.124643882216989,0.792249233913078,
-0.599683685864781));
#49830=CARTESIAN_POINT('Ctrl Pts',(0.256256077438462,0.759952477978614,
-0.604969522723429));
#49831=CARTESIAN_POINT('Ctrl Pts',(0.372153716289941,0.698174612945949,
-0.610255359582077));
#49832=CARTESIAN_POINT('Ctrl Pts',(0.488051355141419,0.636396747913284,
-0.615541196440724));
#49833=CARTESIAN_POINT('Ctrl Pts',(0.588234437622903,0.545137773782418,
-0.620827033299372));
#49834=CARTESIAN_POINT('Ctrl Pts',(0.660526154173397,0.435489814305162,
-0.62611287015802));
#49835=CARTESIAN_POINT('Ctrl Pts',(0.732817870723891,0.325841854827906,
-0.631398707016668));
#49836=CARTESIAN_POINT('Ctrl Pts',(0.777218221343395,0.19780491000426,-0.636684543875315));
#49837=CARTESIAN_POINT('Ctrl Pts',(0.788330540242214,0.066941302885881,
-0.641970380733963));
#49838=CARTESIAN_POINT('Ctrl Pts',(0.799442859141033,-0.0639223042324982,
-0.647256217592611));
#49839=CARTESIAN_POINT('Ctrl Pts',(0.777267146319167,-0.197612573645611,
-0.652542054451259));
#49840=CARTESIAN_POINT('Ctrl Pts',(0.724498761364504,-0.31788004575931,
-0.657827891309907));
#49841=CARTESIAN_POINT('Ctrl Pts',(0.671730376409841,-0.438147517873008,
-0.663113728168555));
#49842=CARTESIAN_POINT('Ctrl Pts',(0.588369319322382,-0.544992192687291,
-0.668399565027202));
#49843=CARTESIAN_POINT('Ctrl Pts',(0.484547757049015,-0.625427573624165,
-0.67368540188585));
#49844=CARTESIAN_POINT('Ctrl Pts',(0.380726194775648,-0.705862954561039,
-0.678971238744498));
#49845=CARTESIAN_POINT('Ctrl Pts',(0.256444127316373,-0.759889041620504,
-0.684257075603146));
#49846=CARTESIAN_POINT('Ctrl Pts',(0.126807489024694,-0.780939203419763,
-0.689542912461794));
#49847=CARTESIAN_POINT('Ctrl Pts',(-0.00282914926697755,-0.801989365219021,
-0.694828749320442));
#49848=CARTESIAN_POINT('Ctrl Pts',(-0.137820358391053,-0.790063601758076,
-0.700114586179089));
#49849=CARTESIAN_POINT('Ctrl Pts',(-0.261758555298625,-0.746611436718336,
-0.705400423037737));
#49850=CARTESIAN_POINT('Ctrl Pts',(-0.38569675220621,-0.703159271678591,
-0.710686259896385));
#49851=CARTESIAN_POINT('Ctrl Pts',(-0.498581936897288,-0.628180705060044,
-0.715972096755033));
#49852=CARTESIAN_POINT('Ctrl Pts',(-0.586693415596102,-0.530789049252922,
-0.721257933613681));
#49853=CARTESIAN_POINT('Ctrl Pts',(-0.674804894294906,-0.43339739344581,
-0.726543770472328));
#49854=CARTESIAN_POINT('Ctrl Pts',(-0.738142667001452,-0.313592648450128,
-0.731829607330976));
#49855=CARTESIAN_POINT('Ctrl Pts',(-0.769008308221525,-0.185936549922035,
-0.737115444189623));
#49856=CARTESIAN_POINT('Ctrl Pts',(-0.78370664034055,-0.125146245265584,
-0.739632579185181));
#49857=CARTESIAN_POINT('Ctrl Pts',(-0.791041268808539,-0.0625754895569357,
-0.742149714180739));
#49858=CARTESIAN_POINT('Ctrl Pts',(-0.79103327968755,-2.89210560314168E-6,
-0.744666849176298));
#49859=CARTESIAN_POINT('Ctrl Pts',(-0.791037024154788,-7.56658461008487E-6,
-0.7731331508237));
#49860=CARTESIAN_POINT('Ctrl Pts',(-0.79105629364485,-0.0573599718684727,
-0.770825979499131));
#49861=CARTESIAN_POINT('Ctrl Pts',(-0.784904040672549,-0.114708304793828,
-0.768518808174561));
#49862=CARTESIAN_POINT('Ctrl Pts',(-0.772536929917119,-0.170683533283396,
-0.766211636849992));
#49863=CARTESIAN_POINT('Ctrl Pts',(-0.744203303727385,-0.298925386313782,
-0.760925799991344));
#49864=CARTESIAN_POINT('Ctrl Pts',(-0.683248546532655,-0.419959959427814,
-0.755639963132697));
#49865=CARTESIAN_POINT('Ctrl Pts',(-0.597081438855663,-0.519076036813415,
-0.750354126274049));
#49866=CARTESIAN_POINT('Ctrl Pts',(-0.510914331178661,-0.618192114199027,
-0.745068289415401));
#49867=CARTESIAN_POINT('Ctrl Pts',(-0.39953487301939,-0.695389695856203,
-0.739782452556753));
#49868=CARTESIAN_POINT('Ctrl Pts',(-0.276480743768598,-0.741285757953729,
-0.734496615698105));
#49869=CARTESIAN_POINT('Ctrl Pts',(-0.15342661451782,-0.78718182005125,
-0.729210778839458));
#49870=CARTESIAN_POINT('Ctrl Pts',(-0.0186978141755228,-0.801776362589129,
-0.72392494198081));
#49871=CARTESIAN_POINT('Ctrl Pts',(0.111329968833544,-0.783295483619938,
-0.718639105122162));
#49872=CARTESIAN_POINT('Ctrl Pts',(0.241357751842625,-0.764814604650745,
-0.713353268263514));
#49873=CARTESIAN_POINT('Ctrl Pts',(0.366684517518475,-0.713258304174474,
-0.708067431404866));
#49874=CARTESIAN_POINT('Ctrl Pts',(0.472077353070542,-0.634893021963372,
-0.702781594546217));
#49875=CARTESIAN_POINT('Ctrl Pts',(0.577470188622603,-0.556527739752275,
-0.69749575768757));
#49876=CARTESIAN_POINT('Ctrl Pts',(0.662929094050884,-0.451353475806351,
-0.692209920828922));
#49877=CARTESIAN_POINT('Ctrl Pts',(0.718066918242495,-0.332153695667528,
-0.686924083970274));
#49878=CARTESIAN_POINT('Ctrl Pts',(0.773204742434107,-0.212953915528704,
-0.681638247111627));
#49879=CARTESIAN_POINT('Ctrl Pts',(0.798021485389048,-0.0797286191969827,
-0.676352410252979));
#49880=CARTESIAN_POINT('Ctrl Pts',(0.78950078201452,0.0513292491502936,
-0.671066573394331));
#49881=CARTESIAN_POINT('Ctrl Pts',(0.780980078639991,0.182387117497577,
-0.665780736535683));
#49882=CARTESIAN_POINT('Ctrl Pts',(0.739121928935989,0.311277557860415,
-0.660494899677034));
#49883=CARTESIAN_POINT('Ctrl Pts',(0.66901400544059,0.422334508587931,-0.655209062818386));
#49884=CARTESIAN_POINT('Ctrl Pts',(0.598906081945198,0.533391459315435,
-0.649923225959738));
#49885=CARTESIAN_POINT('Ctrl Pts',(0.500548384658416,0.62661492040762,-0.644637389101092));
#49886=CARTESIAN_POINT('Ctrl Pts',(0.385895855662796,0.690673993431162,
-0.639351552242444));
#49887=CARTESIAN_POINT('Ctrl Pts',(0.271243326667177,0.754733066454704,
-0.634065715383797));
#49888=CARTESIAN_POINT('Ctrl Pts',(0.140295965962721,0.789627751409603,
-0.628779878525149));
#49889=CARTESIAN_POINT('Ctrl Pts',(0.00896984474943487,0.791116754028786,
-0.623494041666501));
#49890=CARTESIAN_POINT('Ctrl Pts',(-0.122356276463859,0.792605756647969,
-0.618208204807853));
#49891=CARTESIAN_POINT('Ctrl Pts',(-0.254061158185983,0.760689076931433,
-0.612922367949206));
#49892=CARTESIAN_POINT('Ctrl Pts',(-0.370136655895347,0.699246045811115,
-0.607636531090558));
#49893=CARTESIAN_POINT('Ctrl Pts',(-0.486212153604717,0.637803014690794,
-0.60235069423191));
#49894=CARTESIAN_POINT('Ctrl Pts',(-0.586658267301324,0.546833632166687,
-0.597064857373262));
#49895=CARTESIAN_POINT('Ctrl Pts',(-0.659266217146009,0.43739482341457,
-0.591779020514613));
#49896=CARTESIAN_POINT('Ctrl Pts',(-0.731874166990686,0.327956014662466,
-0.586493183655966));
#49897=CARTESIAN_POINT('Ctrl Pts',(-0.776643952983447,0.200047779682357,
-0.581207346797319));
#49898=CARTESIAN_POINT('Ctrl Pts',(-0.788134006102694,0.0692167974149916,
-0.575921509938671));
#49899=CARTESIAN_POINT('Ctrl Pts',(-0.790154398533972,0.046211688247417,
-0.574992056900348));
#49900=CARTESIAN_POINT('Ctrl Pts',(-0.791145810275827,0.0231162102499581,
-0.574062603862025));
#49901=CARTESIAN_POINT('Ctrl Pts',(-0.791122640286116,1.87499586476574E-5,
-0.573133150823702));
#49902=CARTESIAN_POINT('Origin',(0.,0.,-2.94));
#49903=CARTESIAN_POINT('',(-0.791091445179114,-2.03764682111252E-5,-0.3446668491763));
#49904=CARTESIAN_POINT('',(-0.791107814146002,-2.00951009365201E-5,-0.373133150823702));
#49905=CARTESIAN_POINT('',(-0.7911,-9.68818082805471E-17,-2.94));
#49906=CARTESIAN_POINT('Ctrl Pts',(-0.791091445179114,-2.03764682111252E-5,
-0.3446668491763));
#49907=CARTESIAN_POINT('Ctrl Pts',(-0.790992936328914,0.0983025670368676,
-0.348622962906527));
#49908=CARTESIAN_POINT('Ctrl Pts',(-0.772614090163263,0.196661307733409,
-0.352579076636755));
#49909=CARTESIAN_POINT('Ctrl Pts',(-0.736807395616188,0.288203124009163,
-0.356535190366982));
#49910=CARTESIAN_POINT('Ctrl Pts',(-0.688965407561815,0.410513840933409,
-0.36182102722563));
#49911=CARTESIAN_POINT('Ctrl Pts',(-0.610011002822924,0.52065489764232,
-0.367106864084277));
#49912=CARTESIAN_POINT('Ctrl Pts',(-0.509540739832612,0.605239137095278,
-0.372392700942925));
#49913=CARTESIAN_POINT('Ctrl Pts',(-0.409070476842299,0.689823376548237,
-0.377678537801572));
#49914=CARTESIAN_POINT('Ctrl Pts',(-0.287084355600562,0.748850798745245,
-0.38296437466022));
#49915=CARTESIAN_POINT('Ctrl Pts',(-0.158409248097563,0.775146882115055,
-0.388250211518869));
#49916=CARTESIAN_POINT('Ctrl Pts',(-0.0297341405945646,0.801442965484864,
-0.393536048377516));
#49917=CARTESIAN_POINT('Ctrl Pts',(0.1056299531697,0.795007710027475,-0.398821885236164));
#49918=CARTESIAN_POINT('Ctrl Pts',(0.231230127528721,0.756623292553696,
-0.404107722094812));
#49919=CARTESIAN_POINT('Ctrl Pts',(0.356830301887734,0.718238875079919,
-0.40939355895346));
#49920=CARTESIAN_POINT('Ctrl Pts',(0.47266655684151,0.647905295589755,-0.414679395812107));
#49921=CARTESIAN_POINT('Ctrl Pts',(0.564659509179019,0.554171288860078,
-0.419965232670754));
#49922=CARTESIAN_POINT('Ctrl Pts',(0.656652461516538,0.460437282130389,
-0.425251069529402));
#49923=CARTESIAN_POINT('Ctrl Pts',(0.72480211123779,0.343302848161179,-0.430536906388051));
#49924=CARTESIAN_POINT('Ctrl Pts',(0.760825170491265,0.217005158150775,
-0.435822743246699));
#49925=CARTESIAN_POINT('Ctrl Pts',(0.796848229744735,0.0907074681403859,
-0.441108580105346));
#49926=CARTESIAN_POINT('Ctrl Pts',(0.80074469853044,-0.0447534779111776,
-0.446394416963993));
#49927=CARTESIAN_POINT('Ctrl Pts',(0.772040978359756,-0.172913002518913,
-0.451680253822641));
#49928=CARTESIAN_POINT('Ctrl Pts',(0.743337258189069,-0.301072527126663,
-0.456966090681289));
#49929=CARTESIAN_POINT('Ctrl Pts',(0.682033349061983,-0.421930630290567,
-0.462251927539937));
#49930=CARTESIAN_POINT('Ctrl Pts',(0.595580469361028,-0.520797545336097,
-0.467537764398585));
#49931=CARTESIAN_POINT('Ctrl Pts',(0.509127589660082,-0.619664460381615,
-0.472823601257233));
#49932=CARTESIAN_POINT('Ctrl Pts',(0.397525739385269,-0.696540187308768,
-0.47810943811588));
#49933=CARTESIAN_POINT('Ctrl Pts',(0.274339628708118,-0.742080822303308,
-0.483395274974527));
#49934=CARTESIAN_POINT('Ctrl Pts',(0.151153518030953,-0.787621457297853,
-0.488681111833175));
#49935=CARTESIAN_POINT('Ctrl Pts',(0.0163831469514432,-0.80182700035978,
-0.493966948691824));
#49936=CARTESIAN_POINT('Ctrl Pts',(-0.113590743369394,-0.782970830702836,
-0.499252785550472));
#49937=CARTESIAN_POINT('Ctrl Pts',(-0.243564633690224,-0.764114661045893,
-0.50453862240912));
#49938=CARTESIAN_POINT('Ctrl Pts',(-0.368742043252385,-0.712196778670083,
-0.509824459267768));
#49939=CARTESIAN_POINT('Ctrl Pts',(-0.473908212837532,-0.633527572024988,
-0.515110296126416));
#49940=CARTESIAN_POINT('Ctrl Pts',(-0.57907438242268,-0.554858365379893,
-0.520396132985063));
#49941=CARTESIAN_POINT('Ctrl Pts',(-0.664229312030816,-0.44943783446551,
-0.525681969843711));
#49942=CARTESIAN_POINT('Ctrl Pts',(-0.719022797463125,-0.330079377481899,
-0.530967806702359));
#49943=CARTESIAN_POINT('Ctrl Pts',(-0.766357987979791,-0.226967570366176,
-0.535534154193671));
#49944=CARTESIAN_POINT('Ctrl Pts',(-0.791034591140219,-0.113453961755914,
-0.540100501684984));
#49945=CARTESIAN_POINT('Ctrl Pts',(-0.791138066768001,1.60959521169762E-5,
-0.544666849176297));
#49946=CARTESIAN_POINT('Ctrl Pts',(-0.791122640286116,1.87499586476574E-5,
-0.573133150823702));
#49947=CARTESIAN_POINT('Ctrl Pts',(-0.791014041611268,-0.108239976577143,
-0.568776767003377));
#49948=CARTESIAN_POINT('Ctrl Pts',(-0.768616759905835,-0.216542250831125,
-0.564420383183053));
#49949=CARTESIAN_POINT('Ctrl Pts',(-0.7254134058197,-0.315787218355868,
-0.560063999362727));
#49950=CARTESIAN_POINT('Ctrl Pts',(-0.672992432171727,-0.436206522304726,
-0.554778162504079));
#49951=CARTESIAN_POINT('Ctrl Pts',(-0.589940164630051,-0.543291400647814,
-0.549492325645431));
#49952=CARTESIAN_POINT('Ctrl Pts',(-0.486351238141156,-0.624026161133036,
-0.544206488786784));
#49953=CARTESIAN_POINT('Ctrl Pts',(-0.38276231165226,-0.704760921618259,
-0.538920651928136));
#49954=CARTESIAN_POINT('Ctrl Pts',(-0.258636726216144,-0.759145564245615,
-0.533634815069489));
#49955=CARTESIAN_POINT('Ctrl Pts',(-0.129061396490065,-0.780569876792528,
-0.528348978210841));
#49956=CARTESIAN_POINT('Ctrl Pts',(0.000513933236015063,-0.801994189339442,
-0.523063141352193));
#49957=CARTESIAN_POINT('Ctrl Pts',(0.135539007252059,-0.790458171805913,
-0.517777304493544));
#49958=CARTESIAN_POINT('Ctrl Pts',(0.259602126381619,-0.747363975983607,
-0.512491467634897));
#49959=CARTESIAN_POINT('Ctrl Pts',(0.383665245511179,-0.704269780161301,
-0.507205630776248));
#49960=CARTESIAN_POINT('Ctrl Pts',(0.496766409754256,-0.629617406050217,
-0.501919793917601));
#49961=CARTESIAN_POINT('Ctrl Pts',(0.585158673978075,-0.532480518787361,
-0.496633957058954));
#49962=CARTESIAN_POINT('Ctrl Pts',(0.67355093820189,-0.435343631524511,
-0.491348120200306));
#49963=CARTESIAN_POINT('Ctrl Pts',(0.737234302406452,-0.31572223110989,
-0.486062283341658));
#49964=CARTESIAN_POINT('Ctrl Pts',(0.768468335982814,-0.188155768478525,
-0.480776446483011));
#49965=CARTESIAN_POINT('Ctrl Pts',(0.799702369559179,-0.0605893058471451,
-0.475490609624363));
#49966=CARTESIAN_POINT('Ctrl Pts',(0.798487072507338,0.0749222190009814,
-0.470204772765715));
#49967=CARTESIAN_POINT('Ctrl Pts',(0.764970158796818,0.201907980947109,
-0.464918935907067));
#49968=CARTESIAN_POINT('Ctrl Pts',(0.731453245086298,0.32889374289323,-0.459633099048419));
#49969=CARTESIAN_POINT('Ctrl Pts',(0.665634714717104,0.447353741937353,
-0.45434726218977));
#49970=CARTESIAN_POINT('Ctrl Pts',(0.575514518279434,0.542889690332724,
-0.449061425331122));
#49971=CARTESIAN_POINT('Ctrl Pts',(0.485394321841764,0.638425638728095,
-0.443775588472475));
#49972=CARTESIAN_POINT('Ctrl Pts',(0.370972459335619,0.711037536474715,
-0.438489751613827));
#49973=CARTESIAN_POINT('Ctrl Pts',(0.246156400914278,0.751899729291653,
-0.43320391475518));
#49974=CARTESIAN_POINT('Ctrl Pts',(0.121340342492937,0.79276192210859,-0.427918077896532));
#49975=CARTESIAN_POINT('Ctrl Pts',(-0.0138699118435993,0.801874409995844,
-0.422632241037884));
#49976=CARTESIAN_POINT('Ctrl Pts',(-0.143040155074307,0.778129610447774,
-0.417346404179236));
#49977=CARTESIAN_POINT('Ctrl Pts',(-0.272210398305008,0.754384810899704,
-0.412060567320588));
#49978=CARTESIAN_POINT('Ctrl Pts',(-0.395340630429881,0.697782723916312,
-0.406774730461941));
#49979=CARTESIAN_POINT('Ctrl Pts',(-0.497464917569459,0.615203082249481,
-0.401488893603293));
#49980=CARTESIAN_POINT('Ctrl Pts',(-0.599589204709056,0.532623440582635,
-0.396203056744645));
#49981=CARTESIAN_POINT('Ctrl Pts',(-0.68070754686335,0.424066244232339,
-0.390917219885996));
#49982=CARTESIAN_POINT('Ctrl Pts',(-0.730960369152815,0.302726139181895,
-0.385631383027348));
#49983=CARTESIAN_POINT('Ctrl Pts',(-0.770567559629172,0.207090900518661,
-0.381465305626133));
#49984=CARTESIAN_POINT('Ctrl Pts',(-0.791001278485662,0.103514997377555,
-0.377299228224918));
#49985=CARTESIAN_POINT('Ctrl Pts',(-0.791107814146002,-2.00951009365201E-5,
-0.373133150823702));
#49986=CARTESIAN_POINT('Origin',(0.,0.,-2.94));
#49987=CARTESIAN_POINT('',(-0.791053554504038,1.52922707510328E-5,-0.144666849176299));
#49988=CARTESIAN_POINT('',(-0.79104322765544,1.14479096649424E-5,-0.173133150823705));
#49989=CARTESIAN_POINT('',(-0.7911,-9.68818082805471E-17,-2.94));
#49990=CARTESIAN_POINT('Ctrl Pts',(-0.791053554504038,1.52922707510328E-5,
-0.144666849176299));
#49991=CARTESIAN_POINT('Ctrl Pts',(-0.791085703591015,0.0474147764528999,
-0.146573750410772));
#49992=CARTESIAN_POINT('Ctrl Pts',(-0.786893588218416,0.094808539727534,
-0.148480651645245));
#49993=CARTESIAN_POINT('Ctrl Pts',(-0.778423925444021,0.141425176396593,
-0.150387552879717));
#49994=CARTESIAN_POINT('Ctrl Pts',(-0.754946434914425,0.270644210857813,
-0.155673389738365));
#49995=CARTESIAN_POINT('Ctrl Pts',(-0.698601499670502,0.393892027855944,
-0.160959226597013));
#49996=CARTESIAN_POINT('Ctrl Pts',(-0.616234303656779,0.496187532009763,
-0.16624506345566));
#49997=CARTESIAN_POINT('Ctrl Pts',(-0.533867107643055,0.598483036163582,
-0.171530900314307));
#49998=CARTESIAN_POINT('Ctrl Pts',(-0.425477650859533,0.679826227473085,
-0.176816737172955));
#49999=CARTESIAN_POINT('Ctrl Pts',(-0.304241876441027,0.730330646536183,
-0.182102574031602));
#50000=CARTESIAN_POINT('Ctrl Pts',(-0.183006102022508,0.780835065599286,
-0.18738841089025));
#50001=CARTESIAN_POINT('Ctrl Pts',(-0.0489240099689825,0.800500712415977,
-0.1926742477489));
#50002=CARTESIAN_POINT('Ctrl Pts',(0.0817081782642248,0.786937087104024,
-0.197960084607548));
#50003=CARTESIAN_POINT('Ctrl Pts',(0.212340366497417,0.773373461792073,
-0.203245921466195));
#50004=CARTESIAN_POINT('Ctrl Pts',(0.339522650910292,0.726580564351502,
-0.208531758324842));
#50005=CARTESIAN_POINT('Ctrl Pts',(0.44779614723485,0.652245980563451,-0.213817595183489));
#50006=CARTESIAN_POINT('Ctrl Pts',(0.55606964355942,0.577911396775392,-0.219103432042137));
#50007=CARTESIAN_POINT('Ctrl Pts',(0.645434351795641,0.476035126639855,
-0.224389268900785));
#50008=CARTESIAN_POINT('Ctrl Pts',(0.705028613724712,0.358999719529879,
-0.229675105759433));
#50009=CARTESIAN_POINT('Ctrl Pts',(0.764622875653779,0.24196431241991,-0.234960942618081));
#50010=CARTESIAN_POINT('Ctrl Pts',(0.7944466912757,0.109769768335487,-0.24024677947673));
#50011=CARTESIAN_POINT('Ctrl Pts',(0.790874992389185,-0.0215162213875797,
-0.245532616335378));
#50012=CARTESIAN_POINT('Ctrl Pts',(0.78730329350267,-0.152802211110639,
-0.250818453194026));
#50013=CARTESIAN_POINT('Ctrl Pts',(0.750336080107733,-0.283179646472356,
-0.256104290052673));
#50014=CARTESIAN_POINT('Ctrl Pts',(0.68446661229184,-0.396801743794359,
-0.261390126911321));
#50015=CARTESIAN_POINT('Ctrl Pts',(0.618597144475944,-0.510423841116369,
-0.266675963769968));
#50016=CARTESIAN_POINT('Ctrl Pts',(0.523825422239093,-0.607290600398658,
-0.271961800628616));
#50017=CARTESIAN_POINT('Ctrl Pts',(0.411670498006626,-0.675628288467962,
-0.277247637487264));
#50018=CARTESIAN_POINT('Ctrl Pts',(0.299515573774159,-0.743965976537265,
-0.282533474345911));
#50019=CARTESIAN_POINT('Ctrl Pts',(0.16997744754608,-0.783774593393581,
-0.28781931120456));
#50020=CARTESIAN_POINT('Ctrl Pts',(0.0388009198198214,-0.790215582223114,
-0.293105148063208));
#50021=CARTESIAN_POINT('Ctrl Pts',(-0.0923756079064444,-0.796656571052647,
-0.298390984921856));
#50022=CARTESIAN_POINT('Ctrl Pts',(-0.225190537130885,-0.769729931855394,
-0.303676821780504));
#50023=CARTESIAN_POINT('Ctrl Pts',(-0.343500809912295,-0.71270847616472,
-0.308962658639152));
#50024=CARTESIAN_POINT('Ctrl Pts',(-0.461811082693692,-0.655687020474052,
-0.3142484954978));
#50025=CARTESIAN_POINT('Ctrl Pts',(-0.565616699032059,-0.568570748289972,
-0.319534332356447));
#50026=CARTESIAN_POINT('Ctrl Pts',(-0.642300542374549,-0.461948257379328,
-0.324820169215095));
#50027=CARTESIAN_POINT('Ctrl Pts',(-0.71898438571704,-0.355325766468685,
-0.330106006073742));
#50028=CARTESIAN_POINT('Ctrl Pts',(-0.768546456063654,-0.229197056831479,
-0.335391842932389));
#50029=CARTESIAN_POINT('Ctrl Pts',(-0.784962705552036,-0.0988925134430879,
-0.340677679791037));
#50030=CARTESIAN_POINT('Ctrl Pts',(-0.789092433201673,-0.0661126585751875,
-0.342007402919458));
#50031=CARTESIAN_POINT('Ctrl Pts',(-0.791124555828957,-0.033068539627467,
-0.343337126047879));
#50032=CARTESIAN_POINT('Ctrl Pts',(-0.791091445179114,-2.03764682111252E-5,
-0.3446668491763));
#50033=CARTESIAN_POINT('Ctrl Pts',(-0.791107814146002,-2.00951009365201E-5,
-0.373133150823702));
#50034=CARTESIAN_POINT('Ctrl Pts',(-0.791136448830798,-0.0278482864218827,
-0.37201339136627));
#50035=CARTESIAN_POINT('Ctrl Pts',(-0.789696590075878,-0.055673529464667,
-0.370893631908838));
#50036=CARTESIAN_POINT('Ctrl Pts',(-0.786765835743427,-0.0833408443281345,
-0.369773872451406));
#50037=CARTESIAN_POINT('Ctrl Pts',(-0.772931177619944,-0.21394470903718,
-0.364488035592758));
#50038=CARTESIAN_POINT('Ctrl Pts',(-0.725874558948336,-0.341029424704697,
-0.35920219873411));
#50039=CARTESIAN_POINT('Ctrl Pts',(-0.651315503160049,-0.449148407495439,
-0.353916361875462));
#50040=CARTESIAN_POINT('Ctrl Pts',(-0.576756447371763,-0.557267390286181,
-0.348630525016814));
#50041=CARTESIAN_POINT('Ctrl Pts',(-0.474694954466797,-0.646420640200151,
-0.343344688158166));
#50042=CARTESIAN_POINT('Ctrl Pts',(-0.357536146397053,-0.70577197496111,
-0.338058851299519));
#50043=CARTESIAN_POINT('Ctrl Pts',(-0.240377338327316,-0.765123309722065,
-0.332773014440872));
#50044=CARTESIAN_POINT('Ctrl Pts',(-0.1081212150928,-0.794672729330014,
-0.327487177582224));
#50045=CARTESIAN_POINT('Ctrl Pts',(0.0231570776879453,-0.79082863276307,
-0.322201340723576));
#50046=CARTESIAN_POINT('Ctrl Pts',(0.154435370468698,-0.786984536196125,
-0.316915503864928));
#50047=CARTESIAN_POINT('Ctrl Pts',(0.284735832795685,-0.749746923454283,
-0.31162966700628));
#50048=CARTESIAN_POINT('Ctrl Pts',(0.398221021362254,-0.683641861411983,
-0.306343830147633));
#50049=CARTESIAN_POINT('Ctrl Pts',(0.511706209928824,-0.617536799369684,
-0.301057993288985));
#50050=CARTESIAN_POINT('Ctrl Pts',(0.608376124734981,-0.522564288026924,
-0.295772156430336));
#50051=CARTESIAN_POINT('Ctrl Pts',(0.676480965662377,-0.410267814884783,
-0.290486319571689));
#50052=CARTESIAN_POINT('Ctrl Pts',(0.744585806589778,-0.297971341742634,
-0.285200482713041));
#50053=CARTESIAN_POINT('Ctrl Pts',(0.784125573638418,-0.168350906801097,
-0.279914645854393));
#50054=CARTESIAN_POINT('Ctrl Pts',(0.79029438440916,-0.0371612997782024,
-0.274628808995745));
#50055=CARTESIAN_POINT('Ctrl Pts',(0.796463195179903,0.0940283072446845,
-0.269342972137097));
#50056=CARTESIAN_POINT('Ctrl Pts',(0.769261049672759,0.226787086348913,
-0.26405713527845));
#50057=CARTESIAN_POINT('Ctrl Pts',(0.71199424612376,0.344978797360926,-0.258771298419802));
#50058=CARTESIAN_POINT('Ctrl Pts',(0.65472744257476,0.463170508372939,-0.253485461561154));
#50059=CARTESIAN_POINT('Ctrl Pts',(0.567395980983906,0.566795151292719,
-0.248199624702506));
#50060=CARTESIAN_POINT('Ctrl Pts',(0.460614617197846,0.643257608380992,
-0.242913787843858));
#50061=CARTESIAN_POINT('Ctrl Pts',(0.353833253411787,0.719720065469265,
-0.237627950985211));
#50062=CARTESIAN_POINT('Ctrl Pts',(0.227601987430519,0.769020336726032,
-0.232342114126563));
#50063=CARTESIAN_POINT('Ctrl Pts',(0.0972636625592692,0.785166196174475,
-0.227056277267915));
#50064=CARTESIAN_POINT('Ctrl Pts',(-0.0330746623119731,0.801312055622916,
-0.221770440409268));
#50065=CARTESIAN_POINT('Ctrl Pts',(-0.167520046073201,0.784303503263036,
-0.21648460355062));
#50066=CARTESIAN_POINT('Ctrl Pts',(-0.289731233702443,0.736207846505756,
-0.211198766691972));
#50067=CARTESIAN_POINT('Ctrl Pts',(-0.411942421331698,0.688112189748469,
-0.205912929833324));
#50068=CARTESIAN_POINT('Ctrl Pts',(-0.521919412828967,0.608929428593772,
-0.200627092974676));
#50069=CARTESIAN_POINT('Ctrl Pts',(-0.606295020979308,0.508283889784541,
-0.195341256116028));
#50070=CARTESIAN_POINT('Ctrl Pts',(-0.690670629129644,0.407638350975315,
-0.190055419257381));
#50071=CARTESIAN_POINT('Ctrl Pts',(-0.749444853933058,0.285530034511553,
-0.184769582398733));
#50072=CARTESIAN_POINT('Ctrl Pts',(-0.775473893104923,0.156800639274513,
-0.179483745540085));
#50073=CARTESIAN_POINT('Ctrl Pts',(-0.78589796804693,0.105247262512122,
-0.177366880634625));
#50074=CARTESIAN_POINT('Ctrl Pts',(-0.791070266522022,0.0526319761890897,
-0.175250015729165));
#50075=CARTESIAN_POINT('Ctrl Pts',(-0.79104322765544,1.14479096649424E-5,
-0.173133150823705));
#50076=CARTESIAN_POINT('Origin',(0.,0.,-6.17861797838101));
#50077=CARTESIAN_POINT('',(-0.676660270930202,1.30808743349972E-5,-0.0786179783810092));
#50078=CARTESIAN_POINT('',(-0.6767,7.27977111083166E-14,-0.0710999999999995));
#50079=CARTESIAN_POINT('',(-0.6767,7.27977111083166E-14,-6.17861797838101));
#50080=CARTESIAN_POINT('',(-0.657933807534675,-0.158364149874814,-0.0711000000000017));
#50081=CARTESIAN_POINT('Ctrl Pts',(-0.676660270930202,1.30808743350301E-5,
-0.0786179783810092));
#50082=CARTESIAN_POINT('Ctrl Pts',(-0.676624131187738,-0.053270085543402,
-0.0761119855873401));
#50083=CARTESIAN_POINT('Ctrl Pts',(-0.670347495187715,-0.106561703444771,
-0.0736059927936709));
#50084=CARTESIAN_POINT('Ctrl Pts',(-0.657933807534675,-0.158364149874814,
-0.0711000000000017));
#50085=CARTESIAN_POINT('Origin',(0.,0.,-0.0711000000000004));
#50086=CARTESIAN_POINT('Origin',(0.,0.,-6.17861797838101));
#50087=CARTESIAN_POINT('',(-0.676692682281262,-1.74298521427489E-5,-0.278617978381007));
#50088=CARTESIAN_POINT('',(-0.676651437434504,9.79244154855619E-6,-0.239182021618999));
#50089=CARTESIAN_POINT('',(-0.6767,7.27977111083166E-14,-6.17861797838101));
#50090=CARTESIAN_POINT('Ctrl Pts',(-0.676692682281262,-1.7429852142755E-5,
-0.278617978381007));
#50091=CARTESIAN_POINT('Ctrl Pts',(-0.676721004840672,-0.0282865387004088,
-0.277288255252586));
#50092=CARTESIAN_POINT('Ctrl Pts',(-0.668072916989408,-0.168912128805448,
-0.270672695265517));
#50093=CARTESIAN_POINT('Ctrl Pts',(-0.572617975996934,-0.411831935255785,
-0.258771298419802));
#50094=CARTESIAN_POINT('Ctrl Pts',(-0.306234735283331,-0.635387420227233,
-0.242913787843858));
#50095=CARTESIAN_POINT('Ctrl Pts',(0.0345914406976117,-0.704485853085711,
-0.227056277267915));
#50096=CARTESIAN_POINT('Ctrl Pts',(0.367008771067512,-0.602330028183672,
-0.21119876669197));
#50097=CARTESIAN_POINT('Ctrl Pts',(0.610209470489882,-0.353753099832041,
-0.195341256116028));
#50098=CARTESIAN_POINT('Ctrl Pts',(0.705073760608792,-0.0191819564521373,
-0.179483745540084));
#50099=CARTESIAN_POINT('Ctrl Pts',(0.62854066985661,0.320052203509621,-0.16362623496414));
#50100=CARTESIAN_POINT('Ctrl Pts',(0.399215307462047,0.58148440677362,-0.147768724388197));
#50101=CARTESIAN_POINT('Ctrl Pts',(0.0728434763577143,0.701563108700217,
-0.131911213812254));
#50102=CARTESIAN_POINT('Ctrl Pts',(-0.271234459526246,0.651097643395513,
-0.11605370323631));
#50103=CARTESIAN_POINT('Ctrl Pts',(-0.549380630953683,0.442356886629713,
-0.100196192660368));
#50104=CARTESIAN_POINT('Ctrl Pts',(-0.663161936596271,0.193473868574276,
-0.0877176177086003));
#50105=CARTESIAN_POINT('Ctrl Pts',(-0.676687770977166,0.0405581838272357,
-0.0805248796154809));
#50106=CARTESIAN_POINT('Ctrl Pts',(-0.676660270930202,1.30808743350301E-5,
-0.0786179783810092));
#50107=CARTESIAN_POINT('',(-0.364065050236216,0.570420484551968,-0.0711000000000004));
#50108=CARTESIAN_POINT('Origin',(0.,0.,-0.0711000000000004));
#50109=CARTESIAN_POINT('Ctrl Pts',(-0.676651437434504,9.79244154853884E-6,
-0.239182021618999));
#50110=CARTESIAN_POINT('Ctrl Pts',(-0.676616813331805,-0.0673724171628328,
-0.236013049665811));
#50111=CARTESIAN_POINT('Ctrl Pts',(-0.649932577953111,-0.247174784475467,
-0.227558240853975));
#50112=CARTESIAN_POINT('Ctrl Pts',(-0.493004432164587,-0.504424033259022,
-0.21381759518349));
#50113=CARTESIAN_POINT('Ctrl Pts',(-0.192054423564975,-0.67868406853937,
-0.197960084607548));
#50114=CARTESIAN_POINT('Ctrl Pts',(0.155580900692857,-0.687961374427907,
-0.182102574031604));
#50115=CARTESIAN_POINT('Ctrl Pts',(0.465398645427725,-0.530002638582951,
-0.16624506345566));
#50116=CARTESIAN_POINT('Ctrl Pts',(0.662076718045427,-0.243202481582967,
-0.150387552879718));
#50117=CARTESIAN_POINT('Ctrl Pts',(0.697820336995596,0.102713198692547,
-0.134530042303775));
#50118=CARTESIAN_POINT('Ctrl Pts',(0.563909430812559,0.423669692494884,
-0.11867253172783));
#50119=CARTESIAN_POINT('Ctrl Pts',(0.292957635797326,0.641617108208754,
-0.102815021151888));
#50120=CARTESIAN_POINT('Ctrl Pts',(-0.0492916150247689,0.703631926771629,
-0.0869575105759442));
#50121=CARTESIAN_POINT('Ctrl Pts',(-0.269341331211303,0.630876931084481,
-0.0763858368586482));
#50122=CARTESIAN_POINT('Ctrl Pts',(-0.364065050236216,0.570420484551968,
-0.0711000000000004));
#50123=CARTESIAN_POINT('Origin',(0.,0.,-6.17861797838101));
#50124=CARTESIAN_POINT('',(-0.676732561979404,1.37683363057702E-5,-0.478617978381007));
#50125=CARTESIAN_POINT('',(-0.67670668415194,-1.71891729481843E-5,-0.439182021619));
#50126=CARTESIAN_POINT('',(-0.6767,7.27977111083166E-14,-6.17861797838101));
#50127=CARTESIAN_POINT('Ctrl Pts',(-0.676732561979403,1.3768336305774E-5,
-0.478617978381007));
#50128=CARTESIAN_POINT('Ctrl Pts',(-0.676644049835158,-0.0970475236002888,
-0.474051630889693));
#50129=CARTESIAN_POINT('Ctrl Pts',(-0.631101877637816,-0.306543793263608,
-0.464199446539731));
#50130=CARTESIAN_POINT('Ctrl Pts',(-0.422494366982188,-0.564796775530692,
-0.449061425331123));
#50131=CARTESIAN_POINT('Ctrl Pts',(-0.101267392955972,-0.698027078919814,
-0.433203914755179));
#50132=CARTESIAN_POINT('Ctrl Pts',(0.244576786450544,-0.661573188172743,
-0.417346404179235));
#50133=CARTESIAN_POINT('Ctrl Pts',(0.530966517512247,-0.464296720931165,
-0.401488893603292));
#50134=CARTESIAN_POINT('Ctrl Pts',(0.68828299573105,-0.1541538373096,-0.385631383027349));
#50135=CARTESIAN_POINT('Ctrl Pts',(0.678283980079609,0.193462477415893,
-0.369773872451405));
#50136=CARTESIAN_POINT('Ctrl Pts',(0.503400142512799,0.494049779148767,
-0.353916361875461));
#50137=CARTESIAN_POINT('Ctrl Pts',(0.206144193604109,0.674537959812384,
-0.338058851299519));
#50138=CARTESIAN_POINT('Ctrl Pts',(-0.141223581330571,0.691051943005463,
-0.322201340723575));
#50139=CARTESIAN_POINT('Ctrl Pts',(-0.454261155256553,0.539577325634538,
-0.306343830147631));
#50140=CARTESIAN_POINT('Ctrl Pts',(-0.639882056834951,0.280636962336042,
-0.29181604270011));
#50141=CARTESIAN_POINT('Ctrl Pts',(-0.676608418674978,0.0840871534747274,
-0.282574092111234));
#50142=CARTESIAN_POINT('Ctrl Pts',(-0.676692682281262,-1.7429852142755E-5,
-0.278617978381007));
#50143=CARTESIAN_POINT('Ctrl Pts',(-0.67670668415194,-1.71891729482017E-5,
-0.439182021619));
#50144=CARTESIAN_POINT('Ctrl Pts',(-0.676731178010118,-0.0238211799034624,
-0.438062262161566));
#50145=CARTESIAN_POINT('Ctrl Pts',(-0.669685553243432,-0.159977744463465,
-0.431656665845485));
#50146=CARTESIAN_POINT('Ctrl Pts',(-0.580654911117769,-0.400420729098558,
-0.419965232670754));
#50147=CARTESIAN_POINT('Ctrl Pts',(-0.318747394057519,-0.629203452711689,
-0.404107722094813));
#50148=CARTESIAN_POINT('Ctrl Pts',(0.0206447886986398,-0.705032395634334,
-0.388250211518869));
#50149=CARTESIAN_POINT('Ctrl Pts',(0.355018405902544,-0.609474213827725,
-0.372392700942925));
#50150=CARTESIAN_POINT('Ctrl Pts',(0.603090197140036,-0.365758254686112,
-0.356535190366982));
#50151=CARTESIAN_POINT('Ctrl Pts',(0.704556106741155,-0.0331297058619517,
-0.340677679791039));
#50152=CARTESIAN_POINT('Ctrl Pts',(0.634750676840949,0.307552379158318,
-0.324820169215095));
#50153=CARTESIAN_POINT('Ctrl Pts',(0.410642978477166,0.573471210647949,
-0.308962658639151));
#50154=CARTESIAN_POINT('Ctrl Pts',(0.0867116258434061,0.699984269273112,
-0.293105148063209));
#50155=CARTESIAN_POINT('Ctrl Pts',(-0.258298579659923,0.656337369834618,
-0.277247637487264));
#50156=CARTESIAN_POINT('Ctrl Pts',(-0.540518640889337,0.453140652074363,
-0.261390126911321));
#50157=CARTESIAN_POINT('Ctrl Pts',(-0.661202601018511,0.2024097365269,-0.248701588288566));
#50158=CARTESIAN_POINT('Ctrl Pts',(-0.676674566243774,0.0450209307131661,
-0.241298886524459));
#50159=CARTESIAN_POINT('Ctrl Pts',(-0.676651437434504,9.79244154853884E-6,
-0.239182021618999));
#50160=CARTESIAN_POINT('Origin',(0.,0.,-6.17861797838101));
#50161=CARTESIAN_POINT('',(-0.676642928030041,-2.47388173200321E-6,-0.678617978381005));
#50162=CARTESIAN_POINT('',(-0.676719366302129,1.60385502095753E-5,-0.639182021618998));
#50163=CARTESIAN_POINT('',(-0.6767,7.27977111083166E-14,-6.17861797838101));
#50164=CARTESIAN_POINT('Ctrl Pts',(-0.676642928030041,-2.47388173194724E-6,
-0.678617978381005));
#50165=CARTESIAN_POINT('Ctrl Pts',(-0.676649761854052,-0.0535265248175451,
-0.676100843385447));
#50166=CARTESIAN_POINT('Ctrl Pts',(-0.657200799107262,-0.219443081072225,
-0.66829787153124));
#50167=CARTESIAN_POINT('Ctrl Pts',(-0.523043611653193,-0.47320425620448,
-0.655209062818387));
#50168=CARTESIAN_POINT('Ctrl Pts',(-0.233360621587032,-0.66561228059116,
-0.639351552242444));
#50169=CARTESIAN_POINT('Ctrl Pts',(0.113050266597516,-0.696215860924957,
-0.6234940416665));
#50170=CARTESIAN_POINT('Ctrl Pts',(0.431979637282727,-0.55757553815993,
-0.607636531090557));
#50171=CARTESIAN_POINT('Ctrl Pts',(0.645898588102162,-0.283393545566738,
-0.591779020514614));
#50172=CARTESIAN_POINT('Ctrl Pts',(0.702805318729989,0.0596789053693757,
-0.57592150993867));
#50173=CARTESIAN_POINT('Ctrl Pts',(0.588866307489121,0.388243943526985,
-0.560063999362727));
#50174=CARTESIAN_POINT('Ctrl Pts',(0.331779117822002,0.622430321207524,
-0.544206488786783));
#50175=CARTESIAN_POINT('Ctrl Pts',(-0.00596063381383579,0.705309406307461,
-0.52834897821084));
#50176=CARTESIAN_POINT('Ctrl Pts',(-0.34225140821695,0.616734028050019,
-0.512491467634896));
#50177=CARTESIAN_POINT('Ctrl Pts',(-0.595343899704099,0.378236075574855,
-0.496633957058954));
#50178=CARTESIAN_POINT('Ctrl Pts',(-0.672507309873267,0.142947270699369,
-0.485342793974323));
#50179=CARTESIAN_POINT('Ctrl Pts',(-0.676746508256332,0.0153070782871879,
-0.479337467748341));
#50180=CARTESIAN_POINT('Ctrl Pts',(-0.676732561979403,1.3768336305774E-5,
-0.478617978381007));
#50181=CARTESIAN_POINT('Ctrl Pts',(-0.676719366302129,1.60385502095822E-5,
-0.639182021618998));
#50182=CARTESIAN_POINT('Ctrl Pts',(-0.676626471948366,-0.0925875264185486,
-0.634825637798672));
#50183=CARTESIAN_POINT('Ctrl Pts',(-0.634222060982391,-0.297634469454627,
-0.625183417119698));
#50184=CARTESIAN_POINT('Ctrl Pts',(-0.433587460447112,-0.556326163561039,
-0.610255359582076));
#50185=CARTESIAN_POINT('Ctrl Pts',(-0.11505964981147,-0.695886602188015,
-0.594397849006135));
#50186=CARTESIAN_POINT('Ctrl Pts',(0.231438141567586,-0.66628317759591,
-0.578540338430189));
#50187=CARTESIAN_POINT('Ctrl Pts',(0.521675372676006,-0.474712219837212,
-0.562682827854247));
#50188=CARTESIAN_POINT('Ctrl Pts',(0.685097945892652,-0.167742930263535,
-0.546825317278303));
#50189=CARTESIAN_POINT('Ctrl Pts',(0.681979282582143,0.180003178438481,
-0.53096780670236));
#50190=CARTESIAN_POINT('Ctrl Pts',(0.513077502146677,0.483992110380683,
-0.515110296126415));
#50191=CARTESIAN_POINT('Ctrl Pts',(0.219451129913428,0.670326851393724,
-0.499252785550473));
#50192=CARTESIAN_POINT('Ctrl Pts',(-0.127521866330539,0.693711077989502,
-0.483395274974529));
#50193=CARTESIAN_POINT('Ctrl Pts',(-0.443495427494386,0.54846029201429,
-0.467537764398586));
#50194=CARTESIAN_POINT('Ctrl Pts',(-0.636959943577643,0.28955503210012,
-0.452800013280076));
#50195=CARTESIAN_POINT('Ctrl Pts',(-0.676615554482665,0.088545820661681,
-0.443348099020214));
#50196=CARTESIAN_POINT('Ctrl Pts',(-0.67670668415194,-1.71891729482017E-5,
-0.439182021619));
#50197=CARTESIAN_POINT('Origin',(0.,0.,-6.17861797838101));
#50198=CARTESIAN_POINT('',(-0.676745967174656,-9.80469378314186E-6,-0.878617978381005));
#50199=CARTESIAN_POINT('',(-0.676646131014468,-6.47238999015864E-6,-0.839182021618998));
#50200=CARTESIAN_POINT('',(-0.6767,7.27977111083166E-14,-6.17861797838101));
#50201=CARTESIAN_POINT('Ctrl Pts',(-0.676745967174656,-9.80469378311123E-6,
-0.878617978381005));
#50202=CARTESIAN_POINT('Ctrl Pts',(-0.676752985825416,-0.00995529331039852,
-0.878150055881202));
#50203=CARTESIAN_POINT('Ctrl Pts',(-0.674112766541405,-0.132245209733512,
-0.87239629652275));
#50204=CARTESIAN_POINT('Ctrl Pts',(-0.604143565385745,-0.364015714199608,
-0.861356700305653));
#50205=CARTESIAN_POINT('Ctrl Pts',(-0.356776373766072,-0.608446798745448,
-0.845499189729708));
#50206=CARTESIAN_POINT('Ctrl Pts',(-0.0226800088848199,-0.704969861042468,
-0.829641679153765));
#50207=CARTESIAN_POINT('Ctrl Pts',(0.316929665073997,-0.630121000425581,
-0.813784168577821));
#50208=CARTESIAN_POINT('Ctrl Pts',(0.579496547370947,-0.40209531129622,
-0.797926658001879));
#50209=CARTESIAN_POINT('Ctrl Pts',(0.701192956853533,-0.0763238169921492,
-0.782069147425935));
#50210=CARTESIAN_POINT('Ctrl Pts',(0.652435575344282,0.268001320531126,
-0.76621163684999));
#50211=CARTESIAN_POINT('Ctrl Pts',(0.445076890002194,0.547177713149235,
-0.750354126274048));
#50212=CARTESIAN_POINT('Ctrl Pts',(0.129523958779256,0.693340055011537,
-0.734496615698105));
#50213=CARTESIAN_POINT('Ctrl Pts',(-0.217515098455649,0.670957576695487,
-0.718639105122159));
#50214=CARTESIAN_POINT('Ctrl Pts',(-0.511678163758033,0.485471260235309,
-0.702781594546218));
#50215=CARTESIAN_POINT('Ctrl Pts',(-0.654507065922775,0.230147136195413,
-0.689441218965832));
#50216=CARTESIAN_POINT('Ctrl Pts',(-0.676635411221723,0.0588708641822061,
-0.681386680244095));
#50217=CARTESIAN_POINT('Ctrl Pts',(-0.676642928030041,-2.47388173194724E-6,
-0.678617978381005));
#50218=CARTESIAN_POINT('Ctrl Pts',(-0.676646131014468,-6.47238999016905E-6,
-0.839182021618998));
#50219=CARTESIAN_POINT('Ctrl Pts',(-0.676662613967231,-0.0490652167404076,
-0.836874850294427));
#50220=CARTESIAN_POINT('Ctrl Pts',(-0.659343207714862,-0.210508362902118,
-0.829281842111208));
#50221=CARTESIAN_POINT('Ctrl Pts',(-0.532304648268198,-0.462761977210308,
-0.816402997069341));
#50222=CARTESIAN_POINT('Ctrl Pts',(-0.246485614000569,-0.660864379589555,
-0.800545486493398));
#50223=CARTESIAN_POINT('Ctrl Pts',(0.0992518876742048,-0.698316510554226,
-0.784687975917454));
#50224=CARTESIAN_POINT('Ctrl Pts',(0.420862135428632,-0.566014089119677,
-0.76883046534151));
#50225=CARTESIAN_POINT('Ctrl Pts',(0.64016452944956,-0.296118660935354,
-0.752972954765568));
#50226=CARTESIAN_POINT('Ctrl Pts',(0.703848602098822,0.0457605883163558,
-0.737115444189624));
#50227=CARTESIAN_POINT('Ctrl Pts',(0.596433319942227,0.37651584426451,-0.721257933613681));
#50228=CARTESIAN_POINT('Ctrl Pts',(0.34403038572165,0.615743436684253,-0.705400423037737));
#50229=CARTESIAN_POINT('Ctrl Pts',(0.0079967149263957,0.705289258864694,
-0.689542912461795));
#50230=CARTESIAN_POINT('Ctrl Pts',(-0.329980886368106,0.623385515352452,
-0.67368540188585));
#50231=CARTESIAN_POINT('Ctrl Pts',(-0.58774305981707,0.389942280031795,
-0.657827891309908));
#50232=CARTESIAN_POINT('Ctrl Pts',(-0.671068275265414,0.151880359453098,
-0.64632676455429));
#50233=CARTESIAN_POINT('Ctrl Pts',(-0.676739185708065,0.0197734034587098,
-0.64011147465732));
#50234=CARTESIAN_POINT('Ctrl Pts',(-0.676719366302129,1.60385502095822E-5,
-0.639182021618998));
#50235=CARTESIAN_POINT('Origin',(0.,0.,-6.17861797838101));
#50236=CARTESIAN_POINT('',(-0.676676906654629,1.63404783267962E-5,-1.078617978381));
#50237=CARTESIAN_POINT('',(-0.676753912310732,-5.67166874843039E-6,-1.039182021619));
#50238=CARTESIAN_POINT('',(-0.6767,7.27977111083166E-14,-6.17861797838101));
#50239=CARTESIAN_POINT('Ctrl Pts',(-0.676676906654629,1.63404783268123E-5,
-1.078617978381));
#50240=CARTESIAN_POINT('Ctrl Pts',(-0.676605761560008,-0.0787453581397193,
-1.07491343151831));
#50241=CARTESIAN_POINT('Ctrl Pts',(-0.643248328946388,-0.269946967027055,
-1.06592304779696));
#50242=CARTESIAN_POINT('Ctrl Pts',(-0.466925454985086,-0.528656322451762,
-1.05164682721697));
#50243=CARTESIAN_POINT('Ctrl Pts',(-0.157566931955473,-0.687509672466789,
-1.03578931664103));
#50244=CARTESIAN_POINT('Ctrl Pts',(0.190094715234546,-0.679235516607566,
-1.01993180606508));
#50245=CARTESIAN_POINT('Ctrl Pts',(0.491546022542315,-0.505845228804307,
-1.00407429548914));
#50246=CARTESIAN_POINT('Ctrl Pts',(0.673506849846877,-0.209488450733178,
-0.988216784913199));
#50247=CARTESIAN_POINT('Ctrl Pts',(0.691744133306218,0.137793112373883,
-0.972359274337254));
#50248=CARTESIAN_POINT('Ctrl Pts',(0.541824551004231,0.45157839154494,-0.956501763761313));
#50249=CARTESIAN_POINT('Ctrl Pts',(0.260192224202427,0.655588967452813,
-0.940644253185368));
#50250=CARTESIAN_POINT('Ctrl Pts',(-0.0846905254229573,0.700231677864431,
-0.924786742609425));
#50251=CARTESIAN_POINT('Ctrl Pts',(-0.408985759189344,0.574654275683705,
-0.908929232033481));
#50252=CARTESIAN_POINT('Ctrl Pts',(-0.627224599629542,0.317211108211441,
-0.893539643957343));
#50253=CARTESIAN_POINT('Ctrl Pts',(-0.676673700381987,0.102392863337454,
-0.88343589273985));
#50254=CARTESIAN_POINT('Ctrl Pts',(-0.676745967174656,-9.80469378311123E-6,
-0.878617978381005));
#50255=CARTESIAN_POINT('Ctrl Pts',(-0.676753912310732,-5.67166874834366E-6,
-1.039182021619));
#50256=CARTESIAN_POINT('Ctrl Pts',(-0.676756347097398,-0.00548828706568831,
-1.03892406279018));
#50257=CARTESIAN_POINT('Ctrl Pts',(-0.675354290426282,-0.123313979218898,
-1.03338026710272));
#50258=CARTESIAN_POINT('Ctrl Pts',(-0.61122817502222,-0.35199006261332,
-1.0225506345566));
#50259=CARTESIAN_POINT('Ctrl Pts',(-0.368746051047842,-0.601268023394017,
-1.00669312398066));
#50260=CARTESIAN_POINT('Ctrl Pts',(-0.0366250313885693,-0.704383058566367,
-0.990835613404718));
#50261=CARTESIAN_POINT('Ctrl Pts',(0.304399208681507,-0.636268817304129,
-0.974978102828775));
#50262=CARTESIAN_POINT('Ctrl Pts',(0.571426699942949,-0.413483267753163,
-0.959120592252834));
#50263=CARTESIAN_POINT('Ctrl Pts',(0.699545426752022,-0.0901836017791227,
-0.943263081676888));
#50264=CARTESIAN_POINT('Ctrl Pts',(0.657610862529838,0.25503889821415,-0.927405571100947));
#50265=CARTESIAN_POINT('Ctrl Pts',(0.455816928044417,0.538263703241892,
-0.911548060525));
#50266=CARTESIAN_POINT('Ctrl Pts',(0.14321793965191,0.690641374290149,-0.89569054994906));
#50267=CARTESIAN_POINT('Ctrl Pts',(-0.204196060091041,0.675130250516757,
-0.879833039373114));
#50268=CARTESIAN_POINT('Ctrl Pts',(-0.501971808040508,0.495500948588465,
-0.863975528797173));
#50269=CARTESIAN_POINT('Ctrl Pts',(-0.652151980137971,0.239079746805326,
-0.850425189545799));
#50270=CARTESIAN_POINT('Ctrl Pts',(-0.676624850755489,0.0633306492989827,
-0.842160687153075));
#50271=CARTESIAN_POINT('Ctrl Pts',(-0.676646131014468,-6.47238999016905E-6,
-0.839182021618998));
#50272=CARTESIAN_POINT('Origin',(0.,0.,-6.17861797838101));
#50273=CARTESIAN_POINT('',(-0.676672623201375,-1.57520597928919E-5,-1.278617978381));
#50274=CARTESIAN_POINT('',(-0.676665319626825,1.43824383198043E-5,-1.239182021619));
#50275=CARTESIAN_POINT('',(-0.6767,7.27977111083166E-14,-6.17861797838101));
#50276=CARTESIAN_POINT('Ctrl Pts',(-0.676672623201375,-1.57520597928451E-5,
-1.278617978381));
#50277=CARTESIAN_POINT('Ctrl Pts',(-0.676702974356069,-0.0352101549393811,
-1.27696264401406));
#50278=CARTESIAN_POINT('Ctrl Pts',(-0.665389827098819,-0.182768491112835,
-1.27002147278847));
#50279=CARTESIAN_POINT('Ctrl Pts',(-0.559711989719446,-0.429207847488311,
-1.25779446470423));
#50280=CARTESIAN_POINT('Ctrl Pts',(-0.286594754496667,-0.644484549447267,
-1.2419369541283));
#50281=CARTESIAN_POINT('Ctrl Pts',(0.0561911245777891,-0.703092771474672,
-1.22607944355235));
#50282=CARTESIAN_POINT('Ctrl Pts',(0.385317439461293,-0.590785374419714,
-1.21022193297641));
#50283=CARTESIAN_POINT('Ctrl Pts',(0.620776501059534,-0.33486329078227,
-1.19436442240046));
#50284=CARTESIAN_POINT('Ctrl Pts',(0.705330299092296,0.00246108992610756,
-1.17850691182452));
#50285=CARTESIAN_POINT('Ctrl Pts',(0.618424554916906,0.339187201493628,
-1.16264940124858));
#50286=CARTESIAN_POINT('Ctrl Pts',(0.381185284430804,0.593459911632335,
-1.14679189067263));
#50287=CARTESIAN_POINT('Ctrl Pts',(0.0512832509114107,0.703467778904769,
-1.13093438009669));
#50288=CARTESIAN_POINT('Ctrl Pts',(-0.291085286224135,0.642468866113421,
-1.11507686952075));
#50289=CARTESIAN_POINT('Ctrl Pts',(-0.562693571058386,0.425291468137809,
-1.0992193589448));
#50290=CARTESIAN_POINT('Ctrl Pts',(-0.66601953362321,0.179617462040716,
-1.08706639523156));
#50291=CARTESIAN_POINT('Ctrl Pts',(-0.676707275018306,0.0336358601402424,
-1.08019926837696));
#50292=CARTESIAN_POINT('Ctrl Pts',(-0.676676906654629,1.63404783268123E-5,
-1.078617978381));
#50293=CARTESIAN_POINT('Ctrl Pts',(-0.676665319626825,1.43824383197974E-5,
-1.239182021619));
#50294=CARTESIAN_POINT('Ctrl Pts',(-0.676607727494747,-0.0742869656269988,
-1.23568743842729));
#50295=CARTESIAN_POINT('Ctrl Pts',(-0.645946489283497,-0.261021420873604,
-1.22690701837693));
#50296=CARTESIAN_POINT('Ctrl Pts',(-0.477294726647991,-0.519313614334867,
-1.21284076146793));
#50297=CARTESIAN_POINT('Ctrl Pts',(-0.171140054664367,-0.684257238039178,
-1.19698325089199));
#50298=CARTESIAN_POINT('Ctrl Pts',(0.176617247270067,-0.682863993842307,
-1.18112574031604));
#50299=CARTESIAN_POINT('Ctrl Pts',(0.481440462292368,-0.515472567055936,
-1.1652682297401));
#50300=CARTESIAN_POINT('Ctrl Pts',(0.669229769411713,-0.222774329429288,
-1.14941071916415));
#50301=CARTESIAN_POINT('Ctrl Pts',(0.694335253018772,0.124078372550911,
-1.13355320858821));
#50302=CARTESIAN_POINT('Ctrl Pts',(0.550653992635405,0.440768722250355,
-1.11769569801226));
#50303=CARTESIAN_POINT('Ctrl Pts',(0.273113628774048,0.650312103452947,
-1.10183818743633));
#50304=CARTESIAN_POINT('Ctrl Pts',(-0.0708182368002938,0.701770378012652,
-1.08598067686038));
#50305=CARTESIAN_POINT('Ctrl Pts',(-0.397534816887265,0.582634495616192,
-1.07012316628444));
#50306=CARTESIAN_POINT('Ctrl Pts',(-0.623871437853526,0.326107342335911,
-1.05452361453731));
#50307=CARTESIAN_POINT('Ctrl Pts',(-0.676706455860252,0.106856038111985,
-1.04420989964883));
#50308=CARTESIAN_POINT('Ctrl Pts',(-0.676753912310732,-5.67166874834366E-6,
-1.039182021619));
#50309=CARTESIAN_POINT('Origin',(0.,0.,-6.17861797838101));
#50310=CARTESIAN_POINT('',(-0.676749171927519,8.41897198169495E-6,-1.478617978381));
#50311=CARTESIAN_POINT('',(-0.676685230808469,-1.71094250207282E-5,-1.439182021619));
#50312=CARTESIAN_POINT('',(-0.6767,7.27977111083166E-14,-6.17861797838101));
#50313=CARTESIAN_POINT('Ctrl Pts',(-0.676749171927519,8.41897198166925E-6,
-1.478617978381));
#50314=CARTESIAN_POINT('Ctrl Pts',(-0.676684377322802,-0.103966600961598,
-1.47372601965117));
#50315=CARTESIAN_POINT('Ctrl Pts',(-0.626054318658875,-0.320349160458701,
-1.46354822406269));
#50316=CARTESIAN_POINT('Ctrl Pts',(-0.404965598083139,-0.577494374128802,
-1.44808459161556));
#50317=CARTESIAN_POINT('Ctrl Pts',(-0.0798019238330923,-0.700805636916392,
-1.43222708103962));
#50318=CARTESIAN_POINT('Ctrl Pts',(0.264760890572085,-0.65375726275486,
-1.41636957046367));
#50319=CARTESIAN_POINT('Ctrl Pts',(0.544962679865294,-0.447786294269141,
-1.40051205988773));
#50320=CARTESIAN_POINT('Ctrl Pts',(0.692688873355398,-0.13296244774702,
-1.38465454931178));
#50321=CARTESIAN_POINT('Ctrl Pts',(0.672028543154347,0.21418339096928,-1.36879703873584));
#50322=CARTESIAN_POINT('Ctrl Pts',(0.488004032358267,0.509263146303875,
-1.3529395281599));
#50323=CARTESIAN_POINT('Ctrl Pts',(0.185350067969226,0.680545545929922,
-1.33708201758396));
#50324=CARTESIAN_POINT('Ctrl Pts',(-0.162360854618199,0.686393357098464,
-1.32122450700801));
#50325=CARTESIAN_POINT('Ctrl Pts',(-0.470603292949117,0.525385028761478,
-1.30536699643207));
#50326=CARTESIAN_POINT('Ctrl Pts',(-0.644211358515505,0.266799669463018,
-1.29116482022306));
#50327=CARTESIAN_POINT('Ctrl Pts',(-0.676606056624289,0.0771731047055059,
-1.28224848087271));
#50328=CARTESIAN_POINT('Ctrl Pts',(-0.676672623201375,-1.57520597928451E-5,
-1.278617978381));
#50329=CARTESIAN_POINT('Ctrl Pts',(-0.676685230808469,-1.71094250207143E-5,
-1.439182021619));
#50330=CARTESIAN_POINT('Ctrl Pts',(-0.676714877572692,-0.0307457878633605,
-1.43773665092304));
#50331=CARTESIAN_POINT('Ctrl Pts',(-0.667145429154239,-0.173833392972892,
-1.43100544336844));
#50332=CARTESIAN_POINT('Ctrl Pts',(-0.568095276096871,-0.418048613675424,
-1.41898839895519));
#50333=CARTESIAN_POINT('Ctrl Pts',(-0.299291263068257,-0.638687424309053,
-1.40313088837925));
#50334=CARTESIAN_POINT('Ctrl Pts',(0.0422678024777705,-0.704066984734566,
-1.3872733778033));
#50335=CARTESIAN_POINT('Ctrl Pts',(0.373551939990352,-0.598294103471671,
-1.37141586722736));
#50336=CARTESIAN_POINT('Ctrl Pts',(0.614028912825419,-0.347081230166595,
-1.35555835665142));
#50337=CARTESIAN_POINT('Ctrl Pts',(0.705240900970187,-0.0114959870512474,
-1.33970084607548));
#50338=CARTESIAN_POINT('Ctrl Pts',(0.625015078797678,0.326883828592142,
-1.32384333549953));
#50339=CARTESIAN_POINT('Ctrl Pts',(0.392853632391026,0.585801083676619,
-1.30798582492359));
#50340=CARTESIAN_POINT('Ctrl Pts',(0.0651929510142312,0.702315289067225,
-1.29212831434764));
#50341=CARTESIAN_POINT('Ctrl Pts',(-0.27831555874946,0.648102874455513,
-1.2762708037717));
#50342=CARTESIAN_POINT('Ctrl Pts',(-0.554168023743774,0.43634239718304,
-1.26041329319576));
#50343=CARTESIAN_POINT('Ctrl Pts',(-0.664203759053046,0.188552741867401,
-1.24805036581152));
#50344=CARTESIAN_POINT('Ctrl Pts',(-0.676694840205421,0.0380997719910252,
-1.24097327528594));
#50345=CARTESIAN_POINT('Ctrl Pts',(-0.676665319626825,1.43824383197974E-5,
-1.239182021619));
#50346=CARTESIAN_POINT('Origin',(0.,0.,-6.17861797838101));
#50347=CARTESIAN_POINT('',(-0.676643729523802,3.91070869351799E-6,-1.678617978381));
#50348=CARTESIAN_POINT('',(-0.676739142367725,1.21009199712183E-5,-1.639182021619));
#50349=CARTESIAN_POINT('',(-0.6767,7.27977111083166E-14,-6.17861797838101));
#50350=CARTESIAN_POINT('Ctrl Pts',(-0.676643729523802,3.91070869351987E-6,
-1.678617978381));
#50351=CARTESIAN_POINT('Ctrl Pts',(-0.676631511654014,-0.060443692974697,
-1.67577523214692));
#50352=CARTESIAN_POINT('Ctrl Pts',(-0.653687683271354,-0.233297400810955,
-1.6676466490542));
#50353=CARTESIAN_POINT('Ctrl Pts',(-0.508277862304651,-0.489030165196652,
-1.65423222910282));
#50354=CARTESIAN_POINT('Ctrl Pts',(-0.212827550790863,-0.672459159656269,
-1.63837471852688));
#50355=CARTESIAN_POINT('Ctrl Pts',(0.134359251378219,-0.692419294467113,
-1.62251720795094));
#50356=CARTESIAN_POINT('Ctrl Pts',(0.448884510774523,-0.54405843782444,
-1.60665969737499));
#50357=CARTESIAN_POINT('Ctrl Pts',(0.65428992543882,-0.263441798601729,
-1.59080218679905));
#50358=CARTESIAN_POINT('Ctrl Pts',(0.700643260203079,0.0812152061701052,
-1.57494467622311));
#50359=CARTESIAN_POINT('Ctrl Pts',(0.576676430357581,0.406129514380929,
-1.55908716564716));
#50360=CARTESIAN_POINT('Ctrl Pts',(0.312524673140342,0.63231733841464,-1.54322965507122));
#50361=CARTESIAN_POINT('Ctrl Pts',(-0.0275990612546199,0.704794423643601,
-1.52737214449527));
#50362=CARTESIAN_POINT('Ctrl Pts',(-0.361013708553533,0.605942233234882,
-1.51151463391933));
#50363=CARTESIAN_POINT('Ctrl Pts',(-0.606669124072505,0.359790858247332,
-1.49565712334339));
#50364=CARTESIAN_POINT('Ctrl Pts',(-0.674560784855072,0.129095479649908,
-1.48469157149728));
#50365=CARTESIAN_POINT('Ctrl Pts',(-0.676754388892557,0.00838001173401543,
-1.47901185650982));
#50366=CARTESIAN_POINT('Ctrl Pts',(-0.676749171927519,8.41897198166925E-6,
-1.478617978381));
#50367=CARTESIAN_POINT('Ctrl Pts',(-0.676739142367725,1.210091997122E-5,
-1.63918202161899));
#50368=CARTESIAN_POINT('Ctrl Pts',(-0.676656450938597,-0.0995045696225097,
-1.63450002656015));
#50369=CARTESIAN_POINT('Ctrl Pts',(-0.629338348642414,-0.311448711915821,
-1.62453219464265));
#50370=CARTESIAN_POINT('Ctrl Pts',(-0.416313374927947,-0.569368123427741,
-1.60927852586652));
#50371=CARTESIAN_POINT('Ctrl Pts',(-0.0936533636192634,-0.699089360241109,
-1.59342101529057));
#50372=CARTESIAN_POINT('Ctrl Pts',(0.251772950048864,-0.658868171748504,
-1.57756350471463));
#50373=CARTESIAN_POINT('Ctrl Pts',(0.535995491794349,-0.458481972268986,
-1.56170599413868));
#50374=CARTESIAN_POINT('Ctrl Pts',(0.689922281653143,-0.146642870259839,
-1.54584848356274));
#50375=CARTESIAN_POINT('Ctrl Pts',(0.676135081734832,0.200843813364896,
-1.5299909729868));
#50376=CARTESIAN_POINT('Ctrl Pts',(0.49798543810141,0.49950714665405,-1.51413346241085));
#50377=CARTESIAN_POINT('Ctrl Pts',(0.198779949634609,0.676744721252252,
-1.49827595183491));
#50378=CARTESIAN_POINT('Ctrl Pts',(-0.148747182193283,0.689471654173747,
-1.48241844125896));
#50379=CARTESIAN_POINT('Ctrl Pts',(-0.460115192831522,0.534594140863082,
-1.46656093068302));
#50380=CARTESIAN_POINT('Ctrl Pts',(-0.641447726706004,0.275723280480322,
-1.45214879080303));
#50381=CARTESIAN_POINT('Ctrl Pts',(-0.676606456972008,0.0816314601060807,
-1.44302248778169));
#50382=CARTESIAN_POINT('Ctrl Pts',(-0.676685230808469,-1.71094250207143E-5,
-1.439182021619));
#50383=CARTESIAN_POINT('Origin',(0.,0.,-6.17861797838101));
#50384=CARTESIAN_POINT('',(-0.676728058604507,-1.46844370246448E-5,-1.878617978381));
#50385=CARTESIAN_POINT('',(-0.676642402811546,-1.99994779626067E-7,-1.839182021619));
#50386=CARTESIAN_POINT('',(-0.6767,7.27977111083166E-14,-6.17861797838101));
#50387=CARTESIAN_POINT('Ctrl Pts',(-0.676728058604507,-1.46844370245737E-5,
-1.878617978381));
#50388=CARTESIAN_POINT('Ctrl Pts',(-0.676744117284434,-0.0168821899574054,
-1.87782444464268));
#50389=CARTESIAN_POINT('Ctrl Pts',(-0.672010154326253,-0.14609746486122,
-1.87174507404571));
#50390=CARTESIAN_POINT('Ctrl Pts',(-0.592689897555636,-0.382381449755007,
-1.86037986659008));
#50391=CARTESIAN_POINT('Ctrl Pts',(-0.337939220168536,-0.619107398803415,
-1.84452235601415));
#50392=CARTESIAN_POINT('Ctrl Pts',(-0.00103851454807973,-0.705333828246443,
-1.8286648454382));
#50393=CARTESIAN_POINT('Ctrl Pts',(0.336114644751484,-0.620099857575242,
-1.81280733486226));
#50394=CARTESIAN_POINT('Ctrl Pts',(0.591561313924781,-0.384125109370422,
-1.79694982428632));
#50395=CARTESIAN_POINT('Ctrl Pts',(0.70320467250143,-0.0547729527541542,
-1.78109231371037));
#50396=CARTESIAN_POINT('Ctrl Pts',(0.64390520984823,0.287894023056329,-1.76523480313443));
#50397=CARTESIAN_POINT('Ctrl Pts',(0.428078099583546,0.560576514347677,
-1.74937729255848));
#50398=CARTESIAN_POINT('Ctrl Pts',(0.10818899867648,0.69698782510646,-1.73351978198254));
#50399=CARTESIAN_POINT('Ctrl Pts',(-0.237999888598618,0.663967575118165,
-1.7176622714066));
#50400=CARTESIAN_POINT('Ctrl Pts',(-0.526333113076832,0.469542694395412,
-1.70180476083065));
#50401=CARTESIAN_POINT('Ctrl Pts',(-0.657967270519695,0.216292294824611,
-1.68878999648879));
#50402=CARTESIAN_POINT('Ctrl Pts',(-0.676654229709424,0.051953315149448,
-1.68106106900557));
#50403=CARTESIAN_POINT('Ctrl Pts',(-0.676643729523802,3.91070869351987E-6,
-1.678617978381));
#50404=CARTESIAN_POINT('Ctrl Pts',(-0.676642402811546,-1.99994779622598E-7,
-1.839182021619));
#50405=CARTESIAN_POINT('Ctrl Pts',(-0.676642980117375,-0.0559834906210994,
-1.8365492390559));
#50406=CARTESIAN_POINT('Ctrl Pts',(-0.655979709932234,-0.224364000430775,
-1.82863061963417));
#50407=CARTESIAN_POINT('Ctrl Pts',(-0.51785494220135,-0.478876962232637,
-1.81542616335378));
#50408=CARTESIAN_POINT('Ctrl Pts',(-0.226092044745908,-0.668116212512566,
-1.79956865277784));
#50409=CARTESIAN_POINT('Ctrl Pts',(0.120631824241489,-0.694942335089534,
-1.78371114220189));
#50410=CARTESIAN_POINT('Ctrl Pts',(0.438031166284854,-0.552834137407103,
-1.76785363162595));
#50411=CARTESIAN_POINT('Ctrl Pts',(0.648949015415239,-0.276336862381976,
-1.75199612105));
#50412=CARTESIAN_POINT('Ctrl Pts',(0.702113112519488,0.0673354538688382,
-1.73613861047406));
#50413=CARTESIAN_POINT('Ctrl Pts',(0.584599736947659,0.394639118284352,
-1.72028109989812));
#50414=CARTESIAN_POINT('Ctrl Pts',(0.324975348420559,0.626009511939285,
-1.70442358932217));
#50415=CARTESIAN_POINT('Ctrl Pts',(-0.0136476660564434,0.705202543480052,
-1.68856607874623));
#50416=CARTESIAN_POINT('Ctrl Pts',(-0.348953053916159,0.612967089069317,
-1.67270856817029));
#50417=CARTESIAN_POINT('Ctrl Pts',(-0.599431048207782,0.371724769909193,
-1.65685105759434));
#50418=CARTESIAN_POINT('Ctrl Pts',(-0.673261370829587,0.138027284702877,
-1.64567554207725));
#50419=CARTESIAN_POINT('Ctrl Pts',(-0.67674980716783,0.0128468700077985,
-1.6397858634188));
#50420=CARTESIAN_POINT('Ctrl Pts',(-0.676739142367725,1.210091997122E-5,
-1.63918202161899));
#50421=CARTESIAN_POINT('Origin',(0.,0.,-6.17861797838101));
#50422=CARTESIAN_POINT('',(-0.6766975754333,1.74675394711349E-5,-2.078617978381));
#50423=CARTESIAN_POINT('',(-0.676740228638047,-1.17804846946346E-5,-2.03918202161899));
#50424=CARTESIAN_POINT('',(-0.6767,7.27977111083166E-14,-6.17861797838101));
#50425=CARTESIAN_POINT('Ctrl Pts',(-0.6766975754333,1.74675394711173E-5,
-2.078617978381));
#50426=CARTESIAN_POINT('Ctrl Pts',(-0.676610386945761,-0.085659472551938,
-2.07458782027978));
#50427=CARTESIAN_POINT('Ctrl Pts',(-0.638863309880312,-0.28378240291994,
-2.06527182531992));
#50428=CARTESIAN_POINT('Ctrl Pts',(-0.450484675054114,-0.542734230837378,
-2.05066999350141));
#50429=CARTESIAN_POINT('Ctrl Pts',(-0.13639766348118,-0.692020639271782,
-2.03481248292547));
#50430=CARTESIAN_POINT('Ctrl Pts',(0.210846410774077,-0.67308296579615,
-2.01895497234952));
#50431=CARTESIAN_POINT('Ctrl Pts',(0.506835591947215,-0.490524790929845,
-2.00309746177358));
#50432=CARTESIAN_POINT('Ctrl Pts',(0.679617534353063,-0.188724388411024,
-1.98723995119763));
#50433=CARTESIAN_POINT('Ctrl Pts',(0.687190479687935,0.158953239688651,
-1.97138244062169));
#50434=CARTESIAN_POINT('Ctrl Pts',(0.527713512083115,0.467990744509071,
-1.95552493004575));
#50435=CARTESIAN_POINT('Ctrl Pts',(0.239954068430876,0.663263848573645,
-1.93966741946981));
#50436=CARTESIAN_POINT('Ctrl Pts',(-0.106136081809596,0.697303391587448,
-1.92380990889386));
#50437=CARTESIAN_POINT('Ctrl Pts',(-0.426425491571088,0.561834662440479,
-1.90795239831792));
#50438=CARTESIAN_POINT('Ctrl Pts',(-0.632214195584207,0.303402487836874,
-1.8928884214803));
#50439=CARTESIAN_POINT('Ctrl Pts',(-0.67663714821915,0.0954745733244865,
-1.88311028150133));
#50440=CARTESIAN_POINT('Ctrl Pts',(-0.676728058604507,-1.46844370245737E-5,
-1.878617978381));
#50441=CARTESIAN_POINT('Ctrl Pts',(-0.676740228638047,-1.17804846946623E-5,
-2.03918202161899));
#50442=CARTESIAN_POINT('Ctrl Pts',(-0.676750329773678,-0.012415612487542,
-2.03859845155166));
#50443=CARTESIAN_POINT('Ctrl Pts',(-0.67339073835084,-0.137164892122005,
-2.03272904462567));
#50444=CARTESIAN_POINT('Ctrl Pts',(-0.600140158358559,-0.370578839715501,
-2.02157380084104));
#50445=CARTESIAN_POINT('Ctrl Pts',(-0.350123530259618,-0.612299272968753,
-2.0057162902651));
#50446=CARTESIAN_POINT('Ctrl Pts',(-0.0149949761710098,-0.705175181645777,
-1.98985877968915));
#50447=CARTESIAN_POINT('Ctrl Pts',(0.323778723678411,-0.626629255790618,
-1.97400126911321));
#50448=CARTESIAN_POINT('Ctrl Pts',(0.583844686443398,-0.395755313585723,
-1.95814375853727));
#50449=CARTESIAN_POINT('Ctrl Pts',(0.701983182336375,-0.0686767634387369,
-1.94228624796132));
#50450=CARTESIAN_POINT('Ctrl Pts',(0.649475790428822,0.275096499007858,
-1.92642873738538));
#50451=CARTESIAN_POINT('Ctrl Pts',(0.439086592159748,0.551996241567879,
-1.91057122680944));
#50452=CARTESIAN_POINT('Ctrl Pts',(0.121959336304979,0.694710591834882,
-1.89471371623349));
#50453=CARTESIAN_POINT('Ctrl Pts',(-0.224815152906662,0.668546956573044,
-1.87885620565755));
#50454=CARTESIAN_POINT('Ctrl Pts',(-0.516939071671466,0.479865483546136,
-1.86299869508161));
#50455=CARTESIAN_POINT('Ctrl Pts',(-0.655762648669376,0.225226555268029,
-1.84977396706875));
#50456=CARTESIAN_POINT('Ctrl Pts',(-0.676641821060614,0.0564141472276884,
-1.84183507591455));
#50457=CARTESIAN_POINT('Ctrl Pts',(-0.676642402811546,-1.99994779622598E-7,
-1.839182021619));
#50458=CARTESIAN_POINT('Origin',(0.,0.,-6.17861797838101));
#50459=CARTESIAN_POINT('',(-0.676656556320913,-1.19096857998774E-5,-2.278617978381));
#50460=CARTESIAN_POINT('',(-0.676683955905987,1.70211467142023E-5,-2.23918202161899));
#50461=CARTESIAN_POINT('',(-0.6767,7.27977111083166E-14,-6.17861797838101));
#50462=CARTESIAN_POINT('Ctrl Pts',(-0.676656556320913,-1.19096857998831E-5,
-2.278617978381));
#50463=CARTESIAN_POINT('Ctrl Pts',(-0.676683115505212,-0.0421320665452035,
-2.27663703277554));
#50464=CARTESIAN_POINT('Ctrl Pts',(-0.662482884559255,-0.196625443856858,
-2.26937025031143));
#50465=CARTESIAN_POINT('Ctrl Pts',(-0.546278931161056,-0.446179579486538,
-2.25681763098868));
#50466=CARTESIAN_POINT('Ctrl Pts',(-0.266684887662029,-0.652974776292271,
-2.24096012041273));
#50467=CARTESIAN_POINT('Ctrl Pts',(0.0777378875832581,-0.701037594295302,
-2.22510260983679));
#50468=CARTESIAN_POINT('Ctrl Pts',(0.403263271585882,-0.578684388566949,
-2.20924509926084));
#50469=CARTESIAN_POINT('Ctrl Pts',(0.630758929622586,-0.315658138628835,
-2.1933875886849));
#50470=CARTESIAN_POINT('Ctrl Pts',(0.704922684214943,0.0241018061657587,
-2.17753007810895));
#50471=CARTESIAN_POINT('Ctrl Pts',(0.607725984161892,0.358002815569531,
-2.16167256753301));
#50472=CARTESIAN_POINT('Ctrl Pts',(0.362796485494498,0.604876514583012,
-2.14581505695707));
#50473=CARTESIAN_POINT('Ctrl Pts',(0.0296743777790237,0.704710095773204,
-2.12995754638113));
#50474=CARTESIAN_POINT('Ctrl Pts',(-0.310661308079694,0.633234900683358,
-2.11410003580518));
#50475=CARTESIAN_POINT('Ctrl Pts',(-0.575477984286229,0.407825915536408,
-2.09824252522924));
#50476=CARTESIAN_POINT('Ctrl Pts',(-0.668652086086511,0.165761324663879,
-2.08641517275451));
#50477=CARTESIAN_POINT('Ctrl Pts',(-0.676724740802238,0.026711882739232,
-2.07987365713843));
#50478=CARTESIAN_POINT('Ctrl Pts',(-0.6766975754333,1.74675394711173E-5,
-2.078617978381));
#50479=CARTESIAN_POINT('Ctrl Pts',(-0.676683955905987,1.70211467142092E-5,
-2.23918202161899));
#50480=CARTESIAN_POINT('Ctrl Pts',(-0.676606246433108,-0.0812010095403874,
-2.23536182718876));
#50481=CARTESIAN_POINT('Ctrl Pts',(-0.641718981747392,-0.274861857426088,
-2.22625579589989));
#50482=CARTESIAN_POINT('Ctrl Pts',(-0.461135729708285,-0.533714085354632,
-2.21186392775236));
#50483=CARTESIAN_POINT('Ctrl Pts',(-0.150064190853226,-0.689186204695865,
-2.19600641717642));
#50484=CARTESIAN_POINT('Ctrl Pts',(0.197486622320041,-0.677123268042198,
-2.18014890660047));
#50485=CARTESIAN_POINT('Ctrl Pts',(0.497030188535669,-0.500457668343409,
-2.16429139602453));
#50486=CARTESIAN_POINT('Ctrl Pts',(0.675750122618055,-0.20213524655836,
-2.14843388544859));
#50487=CARTESIAN_POINT('Ctrl Pts',(0.690201193133537,0.145324461521679,
-2.13257637487265));
#50488=CARTESIAN_POINT('Ctrl Pts',(0.536870472963871,0.457457081461282,
-2.1167188642967));
#50489=CARTESIAN_POINT('Ctrl Pts',(0.253031300742842,0.65838594073986,-2.10086135372076));
#50490=CARTESIAN_POINT('Ctrl Pts',(-0.0923175372979227,0.699267015114235,
-2.08500384314482));
#50491=CARTESIAN_POINT('Ctrl Pts',(-0.415224800514443,0.57016247785808,
-2.06914633256887));
#50492=CARTESIAN_POINT('Ctrl Pts',(-0.629025916191861,0.3123083083271,-2.05387239206027));
#50493=CARTESIAN_POINT('Ctrl Pts',(-0.676658836124467,0.0999353048383027,
-2.0438842884103));
#50494=CARTESIAN_POINT('Ctrl Pts',(-0.676740228638047,-1.17804846946623E-5,
-2.03918202161899));
#50495=CARTESIAN_POINT('Origin',(0.,0.,-6.17861797838101));
#50496=CARTESIAN_POINT('',(-0.676757533991425,1.53215262135908E-6,-2.478617978381));
#50497=CARTESIAN_POINT('',(-0.676666358633788,-1.46093892624266E-5,-2.43918202161899));
#50498=CARTESIAN_POINT('',(-0.6767,7.27977111083166E-14,-6.17861797838101));
#50499=CARTESIAN_POINT('Ctrl Pts',(-0.676757533991425,1.53215262137176E-6,
-2.478617978381));
#50500=CARTESIAN_POINT('Ctrl Pts',(-0.676742969913277,-0.110890132171142,
-2.47340040841265));
#50501=CARTESIAN_POINT('Ctrl Pts',(-0.620749487720945,-0.334138543334539,
-2.46289700158564));
#50502=CARTESIAN_POINT('Ctrl Pts',(-0.387055478021894,-0.589648153320687,
-2.4471077579));
#50503=CARTESIAN_POINT('Ctrl Pts',(-0.0582613062111292,-0.70292425479551,
-2.43125024732405));
#50504=CARTESIAN_POINT('Ctrl Pts',(0.284695672591286,-0.645325702098597,
-2.41539273674811));
#50505=CARTESIAN_POINT('Ctrl Pts',(0.558445657515852,-0.430854192718303,
-2.39953522617216));
#50506=CARTESIAN_POINT('Ctrl Pts',(0.696442454311359,-0.111645849067578,
-2.38367771559622));
#50507=CARTESIAN_POINT('Ctrl Pts',(0.665140265164793,0.234702610632607,
-2.36782020502028));
#50508=CARTESIAN_POINT('Ctrl Pts',(0.472148374730573,0.523996946575577,
-2.35196269444434));
#50509=CARTESIAN_POINT('Ctrl Pts',(0.164381400495464,0.685912270594717,
-2.33610518386839));
#50510=CARTESIAN_POINT('Ctrl Pts',(-0.183345234784635,0.681088402972051,
-2.32024767329245));
#50511=CARTESIAN_POINT('Ctrl Pts',(-0.486502269038555,0.510697983157941,
-2.3043901627165));
#50512=CARTESIAN_POINT('Ctrl Pts',(-0.648297829736711,0.252955391533677,
-2.29051359774602));
#50513=CARTESIAN_POINT('Ctrl Pts',(-0.676612246565188,0.0702588426274883,
-2.28192286963419));
#50514=CARTESIAN_POINT('Ctrl Pts',(-0.676656556320913,-1.19096857998831E-5,
-2.278617978381));
#50515=CARTESIAN_POINT('Ctrl Pts',(-0.676666358633788,-1.4609389262385E-5,
-2.43918202161899));
#50516=CARTESIAN_POINT('Ctrl Pts',(-0.676696070333537,-0.0376688183928807,
-2.43741103968452));
#50517=CARTESIAN_POINT('Ctrl Pts',(-0.664383137857744,-0.187690043031484,
-2.43035422089139));
#50518=CARTESIAN_POINT('Ctrl Pts',(-0.555000672657401,-0.435282826986497,
-2.41801156523963));
#50519=CARTESIAN_POINT('Ctrl Pts',(-0.27955329320369,-0.647569951726063,
-2.40215405466368));
#50520=CARTESIAN_POINT('Ctrl Pts',(0.0638510132913964,-0.702438562595467,
-2.38629654408774));
#50521=CARTESIAN_POINT('Ctrl Pts',(0.391733704562298,-0.586550586760786,
-2.3704390335118));
#50522=CARTESIAN_POINT('Ctrl Pts',(0.624389405388874,-0.328077363677613,
-2.35458152293585));
#50523=CARTESIAN_POINT('Ctrl Pts',(0.70526157763973,0.0101485577617963,
-2.33872401235991));
#50524=CARTESIAN_POINT('Ctrl Pts',(0.614690913258262,0.345907454787038,
-2.32286650178397));
#50525=CARTESIAN_POINT('Ctrl Pts',(0.374694337750614,0.59757931639001,-2.30700899120802));
#50526=CARTESIAN_POINT('Ctrl Pts',(0.0436128907985044,0.703984944353017,
-2.29115148063208));
#50527=CARTESIAN_POINT('Ctrl Pts',(-0.298070463232192,0.639258073916999,
-2.27529397005614));
#50528=CARTESIAN_POINT('Ctrl Pts',(-0.567295530361938,0.419133233412588,
-2.25943645948019));
#50529=CARTESIAN_POINT('Ctrl Pts',(-0.666979967577887,0.174696049819589,
-2.24739914333448));
#50530=CARTESIAN_POINT('Ctrl Pts',(-0.67671376965045,0.0311768466220108,
-2.24064766404741));
#50531=CARTESIAN_POINT('Ctrl Pts',(-0.676683955905987,1.70211467142092E-5,
-2.23918202161899));
#50532=CARTESIAN_POINT('Origin',(0.,0.,-6.17861797838101));
#50533=CARTESIAN_POINT('',(-0.676651429080103,9.78749391371E-6,-2.678617978381));
#50534=CARTESIAN_POINT('',(-0.676753308202105,6.0958899819781E-6,-2.63918202161899));
#50535=CARTESIAN_POINT('',(-0.6767,7.27977111083166E-14,-6.17861797838101));
#50536=CARTESIAN_POINT('Ctrl Pts',(-0.676651429080103,9.78749391371964E-6,
-2.678617978381));
#50537=CARTESIAN_POINT('Ctrl Pts',(-0.676616861736543,-0.0673593563639852,
-2.6754496209084));
#50538=CARTESIAN_POINT('Ctrl Pts',(-0.649939928618552,-0.247148624797767,
-2.66699542657715));
#50539=CARTESIAN_POINT('Ctrl Pts',(-0.493033473894675,-0.504395560448939,
-2.65325539538726));
#50540=CARTESIAN_POINT('Ctrl Pts',(-0.19209406288682,-0.678672792135419,
-2.63739788481132));
#50541=CARTESIAN_POINT('Ctrl Pts',(0.155541711691216,-0.687970685207893,
-2.62154037423537));
#50542=CARTESIAN_POINT('Ctrl Pts',(0.465366675199364,-0.530029004296125,
-2.60568286365943));
#50543=CARTESIAN_POINT('Ctrl Pts',(0.662065125935696,-0.243241971709246,
-2.58982535308348));
#50544=CARTESIAN_POINT('Ctrl Pts',(0.697821414466598,0.102675027602084,
-2.57396784250754));
#50545=CARTESIAN_POINT('Ctrl Pts',(0.563943504067627,0.423632638026367,
-2.5581103319316));
#50546=CARTESIAN_POINT('Ctrl Pts',(0.292975927787107,0.641608910099083,
-2.54225282135566));
#50547=CARTESIAN_POINT('Ctrl Pts',(-0.0492114989961208,0.703615744670204,
-2.52639531077971));
#50548=CARTESIAN_POINT('Ctrl Pts',(-0.379436046685527,0.594579830011842,
-2.51053780020377));
#50549=CARTESIAN_POINT('Ctrl Pts',(-0.617423055528672,0.341006830258411,
-2.49468028962782));
#50550=CARTESIAN_POINT('Ctrl Pts',(-0.676399412320139,0.115245834625529,
-2.48404034902024));
#50551=CARTESIAN_POINT('Ctrl Pts',(-0.676757724548395,0.0014524430419314,
-2.47868624527129));
#50552=CARTESIAN_POINT('Ctrl Pts',(-0.676757533991425,1.53215262137176E-6,
-2.478617978381));
#50553=CARTESIAN_POINT('Ctrl Pts',(-0.676753308202105,6.0958899819755E-6,
-2.63918202161899));
#50554=CARTESIAN_POINT('Ctrl Pts',(-0.676702953103352,-0.106425038065699,
-2.63417441532163));
#50555=CARTESIAN_POINT('Ctrl Pts',(-0.624199859688166,-0.325248720721236,
-2.62388097216561));
#50556=CARTESIAN_POINT('Ctrl Pts',(-0.398647252183052,-0.581873916279484,
-2.60830169215095));
#50557=CARTESIAN_POINT('Ctrl Pts',(-0.072158885197231,-0.701633794373258,
-2.59244418157501));
#50558=CARTESIAN_POINT('Ctrl Pts',(0.271870667014987,-0.650832717782648,
-2.57658667099906));
#50559=CARTESIAN_POINT('Ctrl Pts',(0.549810870497681,-0.441819977821406,
-2.56072916042312));
#50560=CARTESIAN_POINT('Ctrl Pts',(0.694096926018893,-0.125404718454481,
-2.54487164984717));
#50561=CARTESIAN_POINT('Ctrl Pts',(0.669654172730331,0.221495316122894,
-2.52901413927123));
#50562=CARTESIAN_POINT('Ctrl Pts',(0.48242442724551,0.514551803141691,-2.51315662869529));
#50563=CARTESIAN_POINT('Ctrl Pts',(0.17792158070152,0.682525308864219,-2.49729911811934));
#50564=CARTESIAN_POINT('Ctrl Pts',(-0.169832424647492,0.684582963312612,
-2.4814416075434));
#50565=CARTESIAN_POINT('Ctrl Pts',(-0.476301673309269,0.520224568933759,
-2.46558409696745));
#50566=CARTESIAN_POINT('Ctrl Pts',(-0.645690377045496,0.261883291547497,
-2.45149756832599));
#50567=CARTESIAN_POINT('Ctrl Pts',(-0.676607390040075,0.0747174244931122,
-2.44269687654317));
#50568=CARTESIAN_POINT('Ctrl Pts',(-0.676666358633788,-1.4609389262385E-5,
-2.43918202161899));
#50569=CARTESIAN_POINT('Origin',(0.,0.,-6.17861797838101));
#50570=CARTESIAN_POINT('',(-0.676706726596661,-1.7186887101997E-5,-2.878617978381));
#50571=CARTESIAN_POINT('',(-0.676645697232346,6.098308949265E-6,-2.83918202161899));
#50572=CARTESIAN_POINT('',(-0.6767,7.27977111083166E-14,-6.17861797838101));
#50573=CARTESIAN_POINT('Ctrl Pts',(-0.676706726596661,-1.71868871020019E-5,
-2.878617978381));
#50574=CARTESIAN_POINT('Ctrl Pts',(-0.67673120694042,-0.0238081107658035,
-2.87749883340416));
#50575=CARTESIAN_POINT('Ctrl Pts',(-0.669690139537909,-0.159951598195322,
-2.87109385156866));
#50576=CARTESIAN_POINT('Ctrl Pts',(-0.580678100880426,-0.400387101364609,
-2.85940303287452));
#50577=CARTESIAN_POINT('Ctrl Pts',(-0.318783833330571,-0.629184992977676,
-2.84354552229858));
#50578=CARTESIAN_POINT('Ctrl Pts',(0.0206039577451542,-0.705033591190155,
-2.82768801172263));
#50579=CARTESIAN_POINT('Ctrl Pts',(0.35498310936897,-0.609494774254864,
-2.81183050114669));
#50580=CARTESIAN_POINT('Ctrl Pts',(0.603069014406956,-0.365793181515832,
-2.79597299057075));
#50581=CARTESIAN_POINT('Ctrl Pts',(0.704554188889049,-0.0331705094948168,
-2.78011547999481));
#50582=CARTESIAN_POINT('Ctrl Pts',(0.634768486672358,0.307515619292639,
-2.76425796941886));
#50583=CARTESIAN_POINT('Ctrl Pts',(0.410676193241495,0.573447427482177,
-2.74840045884292));
#50584=CARTESIAN_POINT('Ctrl Pts',(0.0867521583136464,0.699979250270445,
-2.73254294826698));
#50585=CARTESIAN_POINT('Ctrl Pts',(-0.258260557150356,0.656352323376431,
-2.71668543769103));
#50586=CARTESIAN_POINT('Ctrl Pts',(-0.54049242092486,0.453171965929088,
-2.70082792711509));
#50587=CARTESIAN_POINT('Ctrl Pts',(-0.661196692645007,0.202435872569431,
-2.68813877401175));
#50588=CARTESIAN_POINT('Ctrl Pts',(-0.676674531156826,0.045033991551841,
-2.68073545776705));
#50589=CARTESIAN_POINT('Ctrl Pts',(-0.676651429080103,9.78749391371964E-6,
-2.678617978381));
#50590=CARTESIAN_POINT('Ctrl Pts',(-0.676645697232345,6.09830894927194E-6,
-2.83918202161899));
#50591=CARTESIAN_POINT('Ctrl Pts',(-0.676625799079458,-0.0629000889752367,
-2.83622362781738));
#50592=CARTESIAN_POINT('Ctrl Pts',(-0.652383626261716,-0.238217374673108,
-2.82797939715712));
#50593=CARTESIAN_POINT('Ctrl Pts',(-0.502917578453797,-0.494540994662418,
-2.81444932963821));
#50594=CARTESIAN_POINT('Ctrl Pts',(-0.205485567371259,-0.674738888549961,
-2.79859181906227));
#50595=CARTESIAN_POINT('Ctrl Pts',(0.141898163291737,-0.690913740906892,
-2.78273430848633));
#50596=CARTESIAN_POINT('Ctrl Pts',(0.454787708536229,-0.539133588532463,
-2.76687679791038));
#50597=CARTESIAN_POINT('Ctrl Pts',(0.657122394010951,-0.256294840776867,
-2.75101928733444));
#50598=CARTESIAN_POINT('Ctrl Pts',(0.69971645158859,0.0888469104459926,
-2.7351617767585));
#50599=CARTESIAN_POINT('Ctrl Pts',(0.572215643513511,0.412390765461524,
-2.71930426618255));
#50600=CARTESIAN_POINT('Ctrl Pts',(0.305614285798879,0.635686081674883,
-2.70344675560661));
#50601=CARTESIAN_POINT('Ctrl Pts',(-0.0352791951986797,0.704451747464407,
-2.68758924503067));
#50602=CARTESIAN_POINT('Ctrl Pts',(-0.367596616630921,0.601971439157228,
-2.67173173445472));
#50603=CARTESIAN_POINT('Ctrl Pts',(-0.610554559694072,0.353157211106192,
-2.65587422387878));
#50604=CARTESIAN_POINT('Ctrl Pts',(-0.675238312251887,0.124176238940119,
-2.6450243196002));
#50605=CARTESIAN_POINT('Ctrl Pts',(-0.676756106011389,0.00591957877575619,
-2.63946025218027));
#50606=CARTESIAN_POINT('Ctrl Pts',(-0.676753308202105,6.0958899819755E-6,
-2.63918202161899));
#50607=CARTESIAN_POINT('Origin',(0.,0.,-6.17861797838101));
#50608=CARTESIAN_POINT('',(-0.676719327190981,1.60436807500843E-5,-3.078617978381));
#50609=CARTESIAN_POINT('',(-0.676720689883097,-1.58642249737939E-5,-3.03918202161899));
#50610=CARTESIAN_POINT('',(-0.6767,7.27977111083166E-14,-6.17861797838101));
#50611=CARTESIAN_POINT('Ctrl Pts',(-0.676719327190981,1.60436807501024E-5,
-3.078617978381));
#50612=CARTESIAN_POINT('Ctrl Pts',(-0.676626430457751,-0.0925744753283335,
-3.07426220904126));
#50613=CARTESIAN_POINT('Ctrl Pts',(-0.634231039946861,-0.297608388428762,
-3.06462060284287));
#50614=CARTESIAN_POINT('Ctrl Pts',(-0.433619679201001,-0.556301053019741,
-3.04969315978585));
#50615=CARTESIAN_POINT('Ctrl Pts',(-0.115099950991358,-0.695879938684137,
-3.0338356492099));
#50616=CARTESIAN_POINT('Ctrl Pts',(0.231399554821144,-0.666296580968136,
-3.01797813863396));
#50617=CARTESIAN_POINT('Ctrl Pts',(0.521647880459103,-0.474742431844655,
-3.00212062805801));
#50618=CARTESIAN_POINT('Ctrl Pts',(0.685088231319183,-0.167782606634913,
-2.98626311748207));
#50619=CARTESIAN_POINT('Ctrl Pts',(0.681989707179352,0.179963682677014,
-2.97040560690613));
#50620=CARTESIAN_POINT('Ctrl Pts',(0.513105531786303,0.48396239629908,-2.95454809633019));
#50621=CARTESIAN_POINT('Ctrl Pts',(0.219489950840751,0.670314142220776,
-2.93869058575424));
#50622=CARTESIAN_POINT('Ctrl Pts',(-0.127481691142976,0.693718463214421,
-2.92283307517829));
#50623=CARTESIAN_POINT('Ctrl Pts',(-0.443463664270248,0.548485976350586,
-2.90697556460236));
#50624=CARTESIAN_POINT('Ctrl Pts',(-0.636951241452163,0.289581126223947,
-2.89223719900325));
#50625=CARTESIAN_POINT('Ctrl Pts',(-0.676615583758409,0.0885588702252283,
-2.8827846702628));
#50626=CARTESIAN_POINT('Ctrl Pts',(-0.676706726596661,-1.71868871020019E-5,
-2.878617978381));
#50627=CARTESIAN_POINT('Ctrl Pts',(-0.676720689883097,-1.58642249737904E-5,
-3.03918202161899));
#50628=CARTESIAN_POINT('Ctrl Pts',(-0.676739964302642,-0.0193422042320756,
-3.03827284031314));
#50629=CARTESIAN_POINT('Ctrl Pts',(-0.671211161756148,-0.151017847550784,
-3.03207782214863));
#50630=CARTESIAN_POINT('Ctrl Pts',(-0.588486997030099,-0.388818647245757,
-3.02059696712548));
#50631=CARTESIAN_POINT('Ctrl Pts',(-0.331171302414811,-0.62275392778882,
-3.00473945654953));
#50632=CARTESIAN_POINT('Ctrl Pts',(0.00664919963267667,-0.70530324986049,
-2.98888194597359));
#50633=CARTESIAN_POINT('Ctrl Pts',(0.342853340201669,-0.61639960515244,
-2.97302443539765));
#50634=CARTESIAN_POINT('Ctrl Pts',(0.595712873526129,-0.377654681468092,
-2.9571669248217));
#50635=CARTESIAN_POINT('Ctrl Pts',(0.703759888922834,-0.0471052530281482,
-2.94130941424576));
#50636=CARTESIAN_POINT('Ctrl Pts',(0.640729114900228,0.29489504478491,-2.92545190366982));
#50637=CARTESIAN_POINT('Ctrl Pts',(0.421942773788548,0.565208971768099,
-2.90959439309387));
#50638=CARTESIAN_POINT('Ctrl Pts',(0.100585885339081,0.698125608891462,
-2.89373688251793));
#50639=CARTESIAN_POINT('Ctrl Pts',(-0.245222540035754,0.661334100117283,
-2.87787937194199));
#50640=CARTESIAN_POINT('Ctrl Pts',(-0.531419540085806,0.463778135032813,
-2.86202186136604));
#50641=CARTESIAN_POINT('Ctrl Pts',(-0.659140535672339,0.211371023644656,
-2.84912274459171));
#50642=CARTESIAN_POINT('Ctrl Pts',(-0.67666135161134,0.0494959832456144,
-2.84150946467603));
#50643=CARTESIAN_POINT('Ctrl Pts',(-0.676645697232345,6.09830894927194E-6,
-2.83918202161899));
#50644=CARTESIAN_POINT('Origin',(0.,0.,-6.17861797838101));
#50645=CARTESIAN_POINT('',(-0.676646145701304,-6.48367876880208E-6,-3.278617978381));
#50646=CARTESIAN_POINT('',(-0.676705321009977,1.72594551696437E-5,-3.239182021619));
#50647=CARTESIAN_POINT('',(-0.6767,7.27977111083166E-14,-6.17861797838101));
#50648=CARTESIAN_POINT('Ctrl Pts',(-0.676646145701304,-6.48367876878927E-6,
-3.278617978381));
#50649=CARTESIAN_POINT('Ctrl Pts',(-0.67666265341308,-0.0490521592361608,
-3.27631142153702));
#50650=CARTESIAN_POINT('Ctrl Pts',(-0.659349338354501,-0.210482214049339,
-3.26871902783439));
#50651=CARTESIAN_POINT('Ctrl Pts',(-0.532331448398351,-0.462731149618616,
-3.25584079727311));
#50652=CARTESIAN_POINT('Ctrl Pts',(-0.246523886922497,-0.660850104757407,
-3.23998328669717));
#50653=CARTESIAN_POINT('Ctrl Pts',(0.0992114457684886,-0.698322258566757,
-3.22412577612122));
#50654=CARTESIAN_POINT('Ctrl Pts',(0.420829355607847,-0.566038462686005,
-3.20826826554528));
#50655=CARTESIAN_POINT('Ctrl Pts',(0.640147380197513,-0.296155735057606,
-3.19241075496933));
#50656=CARTESIAN_POINT('Ctrl Pts',(0.703851252246643,0.0457198260286,-3.17655324439339));
#50657=CARTESIAN_POINT('Ctrl Pts',(0.596455125262476,0.376481302762003,
-3.16069573381745));
#50658=CARTESIAN_POINT('Ctrl Pts',(0.344066045534297,0.615723512700013,
-3.14483822324151));
#50659=CARTESIAN_POINT('Ctrl Pts',(0.00803756064714361,0.705288795742634,
-3.12898071266556));
#50660=CARTESIAN_POINT('Ctrl Pts',(-0.32994478397183,0.623404625673433,
-3.11312320208962));
#50661=CARTESIAN_POINT('Ctrl Pts',(-0.587720476917705,0.38997631824622,
-3.09726569151367));
#50662=CARTESIAN_POINT('Ctrl Pts',(-0.671063931972615,0.151906504437187,
-3.08576395027747));
#50663=CARTESIAN_POINT('Ctrl Pts',(-0.67673916300584,0.0197864740163767,
-3.07954804589991));
#50664=CARTESIAN_POINT('Ctrl Pts',(-0.676719327190981,1.60436807501024E-5,
-3.078617978381));
#50665=CARTESIAN_POINT('Ctrl Pts',(-0.676705321009976,1.72594551696367E-5,
-3.23918202161899));
#50666=CARTESIAN_POINT('Ctrl Pts',(-0.676614650526792,-0.0881153225781286,
-3.23503621595024));
#50667=CARTESIAN_POINT('Ctrl Pts',(-0.637246565667583,-0.28869418167919,
-3.22560457342284));
#50668=CARTESIAN_POINT('Ctrl Pts',(-0.44454248687824,-0.547611964332075,
-3.2108870940368));
#50669=CARTESIAN_POINT('Ctrl Pts',(-0.128847013424495,-0.693466173112368,
-3.19502958346085));
#50670=CARTESIAN_POINT('Ctrl Pts',(0.218170026627314,-0.670744903522167,
-3.17917207288491));
#50671=CARTESIAN_POINT('Ctrl Pts',(0.512151867514703,-0.484971494750699,
-3.16331456230897));
#50672=CARTESIAN_POINT('Ctrl Pts',(0.681634130178766,-0.181305815392006,
-3.14745705173302));
#50673=CARTESIAN_POINT('Ctrl Pts',(0.68541717920589,0.166433700220129,-3.13159954115708));
#50674=CARTESIAN_POINT('Ctrl Pts',(0.522581388918324,0.473714658920027,
-3.11574203058114));
#50675=CARTESIAN_POINT('Ctrl Pts',(0.232710696222986,0.665839784019352,
-3.0998845200052));
#50676=CARTESIAN_POINT('Ctrl Pts',(-0.113729903497026,0.696105160999459,
-3.08402700942925));
#50677=CARTESIAN_POINT('Ctrl Pts',(-0.432523772013128,0.557153545051146,
-3.0681694988533));
#50678=CARTESIAN_POINT('Ctrl Pts',(-0.633925378362749,0.298494876192099,
-3.05322116958322));
#50679=CARTESIAN_POINT('Ctrl Pts',(-0.676627905864348,0.0930180914472541,
-3.04355867717178));
#50680=CARTESIAN_POINT('Ctrl Pts',(-0.676720689883097,-1.58642249737904E-5,
-3.03918202161899));
#50681=CARTESIAN_POINT('Origin',(0.,0.,-6.17861797838101));
#50682=CARTESIAN_POINT('',(-0.676753931151198,-5.65874007816422E-6,-3.478617978381));
#50683=CARTESIAN_POINT('',(-0.676652143573121,-1.0128264255671E-5,-3.43918202161899));
#50684=CARTESIAN_POINT('',(-0.6767,7.27977111083166E-14,-6.17861797838101));
#50685=CARTESIAN_POINT('Ctrl Pts',(-0.676753931151198,-5.65874007810076E-6,
-3.478617978381));
#50686=CARTESIAN_POINT('Ctrl Pts',(-0.676756355253784,-0.00547521365838144,
-3.47836063403277));
#50687=CARTESIAN_POINT('Ctrl Pts',(-0.675357794150052,-0.12328784257846,
-3.4728174528259));
#50688=CARTESIAN_POINT('Ctrl Pts',(-0.611248559970205,-0.351954664290164,
-3.46198843476037));
#50689=CARTESIAN_POINT('Ctrl Pts',(-0.368780872539474,-0.601246668040893,
-3.44613092418443));
#50690=CARTESIAN_POINT('Ctrl Pts',(-0.0366658246279656,-0.704380937480284,
-3.43027341360848));
#50691=CARTESIAN_POINT('Ctrl Pts',(0.304362360169178,-0.636286446102303,
-3.41441590303255));
#50692=CARTESIAN_POINT('Ctrl Pts',(0.571402753704327,-0.413516361031052,
-3.3985583924566));
#50693=CARTESIAN_POINT('Ctrl Pts',(0.699540203905405,-0.0902241148542729,
-3.38270088188066));
#50694=CARTESIAN_POINT('Ctrl Pts',(0.657625632702926,0.255000813711106,
-3.36684337130472));
#50695=CARTESIAN_POINT('Ctrl Pts',(0.455848100739092,0.538237305315985,
-3.35098586072876));
#50696=CARTESIAN_POINT('Ctrl Pts',(0.143257937062477,0.690633080043126,
-3.33512835015283));
#50697=CARTESIAN_POINT('Ctrl Pts',(-0.204156960980475,0.675142076206533,
-3.31927083957688));
#50698=CARTESIAN_POINT('Ctrl Pts',(-0.501943111877064,0.495530019494702,
-3.30341332900094));
#50699=CARTESIAN_POINT('Ctrl Pts',(-0.652144945246755,0.239105887371835,
-3.28986237526898));
#50700=CARTESIAN_POINT('Ctrl Pts',(-0.67662482340183,0.0633437005471308,
-3.28159725839567));
#50701=CARTESIAN_POINT('Ctrl Pts',(-0.676646145701304,-6.48367876878927E-6,
-3.278617978381));
#50702=CARTESIAN_POINT('Ctrl Pts',(-0.676652143573121,-1.01282642557092E-5,
-3.43918202161899));
#50703=CARTESIAN_POINT('Ctrl Pts',(-0.676675846286291,-0.044590091349477,
-3.437085428446));
#50704=CARTESIAN_POINT('Ctrl Pts',(-0.661396035876845,-0.201547028199607,
-3.42970299841435));
#50705=CARTESIAN_POINT('Ctrl Pts',(-0.541383431856071,-0.452107139770282,
-3.41703473152406));
#50706=CARTESIAN_POINT('Ctrl Pts',(-0.259552071413764,-0.655842670420542,
-3.40117722094812));
#50707=CARTESIAN_POINT('Ctrl Pts',(0.0853740963848333,-0.700148662632442,
-3.38531971037218));
#50708=CARTESIAN_POINT('Ctrl Pts',(0.409546578284193,-0.574254722518878,
-3.36946219979623));
#50709=CARTESIAN_POINT('Ctrl Pts',(0.634161918067455,-0.308764550738151,
-3.35360468922029));
#50710=CARTESIAN_POINT('Ctrl Pts',(0.70461811808652,0.0317835458017981,
-3.33774717864434));
#50711=CARTESIAN_POINT('Ctrl Pts',(0.603787900785698,0.364605344152174,
-3.32188966806841));
#50712=CARTESIAN_POINT('Ctrl Pts',(0.356182198023997,0.608794815952237,
-3.30603215749246));
#50713=CARTESIAN_POINT('Ctrl Pts',(0.021991760855621,0.704991665606051,
-3.29017464691652));
#50714=CARTESIAN_POINT('Ctrl Pts',(-0.317544678396473,0.629811291849872,
-3.27431713634057));
#50715=CARTESIAN_POINT('Ctrl Pts',(-0.579888821700749,0.401529376990078,
-3.25845962576463));
#50716=CARTESIAN_POINT('Ctrl Pts',(-0.669533849297346,0.160840322501936,
-3.24674792085744));
#50717=CARTESIAN_POINT('Ctrl Pts',(-0.676730253963205,0.0242523298834378,
-3.24032205280889));
#50718=CARTESIAN_POINT('Ctrl Pts',(-0.676705321009976,1.72594551696367E-5,
-3.23918202161899));
#50719=CARTESIAN_POINT('Origin',(0.,0.,-6.17861797838101));
#50720=CARTESIAN_POINT('',(-0.676665289551903,1.43754394393928E-5,-3.678617978381));
#50721=CARTESIAN_POINT('',(-0.676757684388521,-1.06428210661091E-6,-3.639182021619));
#50722=CARTESIAN_POINT('',(-0.6767,7.27977111083166E-14,-6.17861797838101));
#50723=CARTESIAN_POINT('Ctrl Pts',(-0.676665289551903,1.43754394393916E-5,
-3.678617978381));
#50724=CARTESIAN_POINT('Ctrl Pts',(-0.676607739317337,-0.0742739175691506,
-3.67512400966988));
#50725=CARTESIAN_POINT('Ctrl Pts',(-0.645954239072405,-0.260995295744918,
-3.66634420410011));
#50726=CARTESIAN_POINT('Ctrl Pts',(-0.47732480187785,-0.519285972556088,
-3.65227856167169));
#50727=CARTESIAN_POINT('Ctrl Pts',(-0.171179682347504,-0.684247326726716,
-3.63642105109576));
#50728=CARTESIAN_POINT('Ctrl Pts',(0.176577700272081,-0.682874222348358,
-3.6205635405198));
#50729=CARTESIAN_POINT('Ctrl Pts',(0.48141060950412,-0.51550044892136,-3.60470602994387));
#50730=CARTESIAN_POINT('Ctrl Pts',(0.66921686778135,-0.222813086819806,
-3.58884851936792));
#50731=CARTESIAN_POINT('Ctrl Pts',(0.694342438818249,0.12403816121331,-3.57299100879198));
#50732=CARTESIAN_POINT('Ctrl Pts',(0.550679519060578,0.440736831985327,
-3.55713349821603));
#50733=CARTESIAN_POINT('Ctrl Pts',(0.273151290577277,0.650296286501176,
-3.54127598764009));
#50734=CARTESIAN_POINT('Ctrl Pts',(-0.0707775948694625,0.701774479334883,
-3.52541847706415));
#50735=CARTESIAN_POINT('Ctrl Pts',(-0.397501074521878,0.582657518217351,
-3.5095609664882));
#50736=CARTESIAN_POINT('Ctrl Pts',(-0.623861468045536,0.326133368546649,
-3.49396080026049));
#50737=CARTESIAN_POINT('Ctrl Pts',(-0.676706564337889,0.106869103155189,
-3.48364647089142));
#50738=CARTESIAN_POINT('Ctrl Pts',(-0.676753931151198,-5.65874007810076E-6,
-3.478617978381));
#50739=CARTESIAN_POINT('Ctrl Pts',(-0.676757684388521,-1.06428210658034E-6,
-3.639182021619));
#50740=CARTESIAN_POINT('Ctrl Pts',(-0.676757777269629,-0.00100806921878618,
-3.63913464094175));
#50741=CARTESIAN_POINT('Ctrl Pts',(-0.676510061530498,-0.114357529906071,
-3.63380142340587));
#50742=CARTESIAN_POINT('Ctrl Pts',(-0.618093122687726,-0.339790785345425,
-3.62318236901133));
#50743=CARTESIAN_POINT('Ctrl Pts',(-0.380605728184695,-0.593831765563718,
-3.60732485843538));
#50744=CARTESIAN_POINT('Ctrl Pts',(-0.0505964556334205,-0.703517508521898,
-3.59146734785944));
#50745=CARTESIAN_POINT('Ctrl Pts',(0.291712366691096,-0.642184382587279,
-3.5756098372835));
#50746=CARTESIAN_POINT('Ctrl Pts',(0.563108499012531,-0.424741926891352,
-3.55975232670755));
#50747=CARTESIAN_POINT('Ctrl Pts',(0.697617947778104,-0.104048474555806,
-3.54389481613161));
#50748=CARTESIAN_POINT('Ctrl Pts',(0.66254265856183,0.241938239444174,-3.52803730555567));
#50749=CARTESIAN_POINT('Ctrl Pts',(0.466409123192545,0.529111912474371,
-3.51217979497972));
#50750=CARTESIAN_POINT('Ctrl Pts',(0.156895665186708,0.687663170720335,
-3.49632228440378));
#50751=CARTESIAN_POINT('Ctrl Pts',(-0.19075773797954,0.679049609027539,
-3.48046477382783));
#50752=CARTESIAN_POINT('Ctrl Pts',(-0.492039626312628,0.505365107875141,
-3.4646072632519));
#50753=CARTESIAN_POINT('Ctrl Pts',(-0.649691444389947,0.248036967307317,
-3.45084634584895));
#50754=CARTESIAN_POINT('Ctrl Pts',(-0.676616088066844,0.067802916062758,
-3.44237126530465));
#50755=CARTESIAN_POINT('Ctrl Pts',(-0.676652143573121,-1.01282642557092E-5,
-3.43918202161899));
#50756=CARTESIAN_POINT('Origin',(0.,0.,-6.17861797838101));
#50757=CARTESIAN_POINT('',(-0.676685270745956,-1.71119534365975E-5,-3.878617978381));
#50758=CARTESIAN_POINT('',(-0.676655703468725,1.16019570828296E-5,-3.83918202161899));
#50759=CARTESIAN_POINT('',(-0.6767,7.27977111083166E-14,-6.17861797838101));
#50760=CARTESIAN_POINT('Ctrl Pts',(-0.676685270745956,-1.71119534366597E-5,
-3.878617978381));
#50761=CARTESIAN_POINT('Ctrl Pts',(-0.676714912134811,-0.0307327214839186,
-3.87717322216564));
#50762=CARTESIAN_POINT('Ctrl Pts',(-0.66715043232197,-0.173807244306441,
-3.87044262909162));
#50763=CARTESIAN_POINT('Ctrl Pts',(-0.568119486722484,-0.418015713325986,
-3.85842619915896));
#50764=CARTESIAN_POINT('Ctrl Pts',(-0.299328251646252,-0.638670091320746,
-3.84256868858302));
#50765=CARTESIAN_POINT('Ctrl Pts',(0.0422270275427583,-0.704069432603173,
-3.82671117800707));
#50766=CARTESIAN_POINT('Ctrl Pts',(0.373517290723508,-0.598315737142038,
-3.81085366743113));
#50767=CARTESIAN_POINT('Ctrl Pts',(0.614008812156318,-0.347116790685268,
-3.79499615685518));
#50768=CARTESIAN_POINT('Ctrl Pts',(0.705240235193272,-0.0115368299714127,
-3.77913864627925));
#50769=CARTESIAN_POINT('Ctrl Pts',(0.625034009757416,0.326847631822259,
-3.76328113570329));
#50770=CARTESIAN_POINT('Ctrl Pts',(0.392887558138946,0.585778332170854,
-3.74742362512736));
#50771=CARTESIAN_POINT('Ctrl Pts',(0.065233624501804,0.702311513514914,
-3.73156611455141));
#50772=CARTESIAN_POINT('Ctrl Pts',(-0.278278024886458,0.648118992659946,
-3.71570860397547));
#50773=CARTESIAN_POINT('Ctrl Pts',(-0.554142753654658,0.436374490951619,
-3.69985109339953));
#50774=CARTESIAN_POINT('Ctrl Pts',(-0.664198309185149,0.188578892491741,
-3.6874875515347));
#50775=CARTESIAN_POINT('Ctrl Pts',(-0.676694803963945,0.0381128350943536,
-3.68040984652853));
#50776=CARTESIAN_POINT('Ctrl Pts',(-0.676665289551903,1.43754394393916E-5,
-3.678617978381));
#50777=CARTESIAN_POINT('Ctrl Pts',(-0.676655703468725,1.16019570828574E-5,
-3.839182021619));
#50778=CARTESIAN_POINT('Ctrl Pts',(-0.676612882638414,-0.069815305702025,
-3.83589801657886));
#50779=CARTESIAN_POINT('Ctrl Pts',(-0.648551748397102,-0.252067159102267,
-3.82732817468008));
#50780=CARTESIAN_POINT('Ctrl Pts',(-0.487506623358711,-0.50973932387144,
-3.81347249592265));
#50781=CARTESIAN_POINT('Ctrl Pts',(-0.184685586744943,-0.680726171208512,
-3.79761498534671));
#50782=CARTESIAN_POINT('Ctrl Pts',(0.163030878572916,-0.686234521684292,
-3.78175747477076));
#50783=CARTESIAN_POINT('Ctrl Pts',(0.471115982751349,-0.524925344135482,
-3.76589996419482));
#50784=CARTESIAN_POINT('Ctrl Pts',(0.664676968465788,-0.236011469447257,
-3.75004245361887));
#50785=CARTESIAN_POINT('Ctrl Pts',(0.696660876212486,0.110274700971604,
-3.73418494304293));
#50786=CARTESIAN_POINT('Ctrl Pts',(0.559292701589483,0.429754069286446,
-3.71832743246699));
#50787=CARTESIAN_POINT('Ctrl Pts',(0.285965429933078,0.644764033583383,
-3.70246992189105));
#50788=CARTESIAN_POINT('Ctrl Pts',(-0.0568775023532221,0.703037577833207,
-3.6866124113151));
#50789=CARTESIAN_POINT('Ctrl Pts',(-0.385894018096841,0.590408920085563,
-3.67075490073916));
#50790=CARTESIAN_POINT('Ctrl Pts',(-0.620400337809798,0.335022444869625,
-3.65494477084045));
#50791=CARTESIAN_POINT('Ctrl Pts',(-0.67674741535816,0.111334432431026,
-3.6444204778004));
#50792=CARTESIAN_POINT('Ctrl Pts',(-0.676757684388521,-1.06428210658034E-6,
-3.639182021619));
#50793=CARTESIAN_POINT('Origin',(0.,0.,-6.17861797838101));
#50794=CARTESIAN_POINT('',(-0.676739110229135,1.21105064106007E-5,-4.078617978381));
#50795=CARTESIAN_POINT('',(-0.676698966456529,-1.74541653144567E-5,-4.039182021619));
#50796=CARTESIAN_POINT('',(-0.6767,7.27977111083166E-14,-6.17861797838101));
#50797=CARTESIAN_POINT('Ctrl Pts',(-0.676739110229135,1.21105064106054E-5,
-4.078617978381));
#50798=CARTESIAN_POINT('Ctrl Pts',(-0.676656380771256,-0.099491513469243,
-4.07393659780274));
#50799=CARTESIAN_POINT('Ctrl Pts',(-0.629347804780193,-0.31142265532354,
-4.06396938036584));
#50800=CARTESIAN_POINT('Ctrl Pts',(-0.416346348986597,-0.569344013287909,
-4.04871632607028));
#50801=CARTESIAN_POINT('Ctrl Pts',(-0.0936938502820333,-0.699083936448678,
-4.03285881549434));
#50802=CARTESIAN_POINT('Ctrl Pts',(0.251734792730736,-0.658882752779327,
-4.01700130491839));
#50803=CARTESIAN_POINT('Ctrl Pts',(0.535968939526595,-0.458513013603747,
-4.00114379434245));
#50804=CARTESIAN_POINT('Ctrl Pts',(0.689913789056643,-0.146682826025263,
-3.98528628376651));
#50805=CARTESIAN_POINT('Ctrl Pts',(0.676146713284492,0.200804656061129,
-3.96942877319056));
#50806=CARTESIAN_POINT('Ctrl Pts',(0.49801436627063,0.499478306605316,-3.95357126261462));
#50807=CARTESIAN_POINT('Ctrl Pts',(0.198819142241936,0.676733209218694,
-3.93771375203867));
#50808=CARTESIAN_POINT('Ctrl Pts',(-0.148707252523208,0.689480268628661,
-3.92185624146274));
#50809=CARTESIAN_POINT('Ctrl Pts',(-0.460084232647476,0.534620787708854,
-3.90599873088679));
#50810=CARTESIAN_POINT('Ctrl Pts',(-0.641439490611294,0.275749392064349,
-3.89158597652621));
#50811=CARTESIAN_POINT('Ctrl Pts',(-0.676606465087421,0.0816445081588362,
-3.88245905902428));
#50812=CARTESIAN_POINT('Ctrl Pts',(-0.676685270745956,-1.71119534366597E-5,
-3.878617978381));
#50813=CARTESIAN_POINT('Ctrl Pts',(-0.676698966456529,-1.74541653144393E-5,
-4.039182021619));
#50814=CARTESIAN_POINT('Ctrl Pts',(-0.676725765237266,-0.0262676949275742,
-4.03794722907462));
#50815=CARTESIAN_POINT('Ctrl Pts',(-0.668813390334722,-0.164872567242388,
-4.03142659967159));
#50816=CARTESIAN_POINT('Ctrl Pts',(-0.576279664676672,-0.406692308999895,
-4.01962013340991));
#50817=CARTESIAN_POINT('Ctrl Pts',(-0.311907214595146,-0.632622142833319,
-4.00376262283397));
#50818=CARTESIAN_POINT('Ctrl Pts',(0.0282871139661857,-0.70476714261023,
-3.98790511225803));
#50819=CARTESIAN_POINT('Ctrl Pts',(0.361605095917608,-0.6055894985268,-3.97204760168208));
#50820=CARTESIAN_POINT('Ctrl Pts',(0.607020085064156,-0.35919841654471,
-3.95619009110614));
#50821=CARTESIAN_POINT('Ctrl Pts',(0.704873873408482,-0.0254893841755349,
-3.9403325805302));
#50822=CARTESIAN_POINT('Ctrl Pts',(0.631379072581692,0.31441589149629,-3.92447506995425));
#50823=CARTESIAN_POINT('Ctrl Pts',(0.40440161705542,0.57788945157572,-3.90861755937831));
#50824=CARTESIAN_POINT('Ctrl Pts',(0.0791177138722245,0.700883209579997,
-3.89276004880237));
#50825=CARTESIAN_POINT('Ctrl Pts',(-0.265399004090862,0.653498473408395,
-3.87690253822642));
#50826=CARTESIAN_POINT('Ctrl Pts',(-0.545399577203117,0.447254052308289,
-3.86104502765048));
#50827=CARTESIAN_POINT('Ctrl Pts',(-0.662288714997138,0.197514295592761,
-3.84847152211467));
#50828=CARTESIAN_POINT('Ctrl Pts',(-0.676681805773553,0.0425760084765945,
-3.84118385343751));
#50829=CARTESIAN_POINT('Ctrl Pts',(-0.676655703468725,1.16019570828574E-5,
-3.839182021619));
#50830=CARTESIAN_POINT('Origin',(0.,0.,-6.17861797838101));
#50831=CARTESIAN_POINT('',(-0.676642404370006,-2.12118767964631E-7,-4.278617978381));
#50832=CARTESIAN_POINT('',(-0.676726753762749,1.49205000514463E-5,-4.239182021619));
#50833=CARTESIAN_POINT('',(-0.6767,7.27977111083166E-14,-6.17861797838101));
#50834=CARTESIAN_POINT('Ctrl Pts',(-0.676642404370006,-2.12118767984465E-7,
-4.27861797838101));
#50835=CARTESIAN_POINT('Ctrl Pts',(-0.676643016530589,-0.0559704364681642,
-4.2759858102985));
#50836=CARTESIAN_POINT('Ctrl Pts',(-0.655986276549325,-0.22433785474264,
-4.26806780535735));
#50837=CARTESIAN_POINT('Ctrl Pts',(-0.517882675605679,-0.478846971472886,
-4.25486396355754));
#50838=CARTESIAN_POINT('Ctrl Pts',(-0.226130737646503,-0.668103118741933,
-4.23900645298161));
#50839=CARTESIAN_POINT('Ctrl Pts',(0.120591577745708,-0.694949321287569,
-4.22314894240565));
#50840=CARTESIAN_POINT('Ctrl Pts',(0.437999149760179,-0.552859505291001,
-4.20729143182972));
#50841=CARTESIAN_POINT('Ctrl Pts',(0.648933011794961,-0.276374445244078,
-4.19143392125377));
#50842=CARTESIAN_POINT('Ctrl Pts',(0.702117012141806,0.0672947920890993,
-4.17557641067783));
#50843=CARTESIAN_POINT('Ctrl Pts',(0.584622591848963,0.394605262105121,
-4.15971890010188));
#50844=CARTESIAN_POINT('Ctrl Pts',(0.325011602776974,0.625990691497561,
-4.14386138952594));
#50845=CARTESIAN_POINT('Ctrl Pts',(-0.0136068253575281,0.705203333858357,
-4.12800387895));
#50846=CARTESIAN_POINT('Ctrl Pts',(-0.348917554886554,0.612987298133689,
-4.11214636837405));
#50847=CARTESIAN_POINT('Ctrl Pts',(-0.599409520346848,0.371759485015262,
-4.09628885779812));
#50848=CARTESIAN_POINT('Ctrl Pts',(-0.673257437461863,0.138053426064092,
-4.08511272780042));
#50849=CARTESIAN_POINT('Ctrl Pts',(-0.676749792193473,0.0128599423431918,
-4.07922243466139));
#50850=CARTESIAN_POINT('Ctrl Pts',(-0.676739110229135,1.21105064106054E-5,
-4.078617978381));
#50851=CARTESIAN_POINT('Ctrl Pts',(-0.676726753762749,1.49205000514446E-5,
-4.239182021619));
#50852=CARTESIAN_POINT('Ctrl Pts',(-0.676635341683233,-0.0950309047916752,
-4.23471060471172));
#50853=CARTESIAN_POINT('Ctrl Pts',(-0.632525590471087,-0.302516277141406,
-4.2249533509458));
#50854=CARTESIAN_POINT('Ctrl Pts',(-0.427530623812185,-0.560994163804123,
-4.20991026032124));
#50855=CARTESIAN_POINT('Ctrl Pts',(-0.107508502335302,-0.697093112894644,
-4.19405274974529));
#50856=CARTESIAN_POINT('Ctrl Pts',(0.238647982882395,-0.663734906710268,
-4.17819523916935));
#50857=CARTESIAN_POINT('Ctrl Pts',(0.526791259328862,-0.469028629418541,
-4.1623377285934));
#50858=CARTESIAN_POINT('Ctrl Pts',(0.68687625119572,-0.160305650751426,
-4.14648021801746));
#50859=CARTESIAN_POINT('Ctrl Pts',(0.679987716283376,0.187386210333744,
-4.13062270744152));
#50860=CARTESIAN_POINT('Ctrl Pts',(0.507800196354854,0.489526145064282,
-4.11476519686557));
#50861=CARTESIAN_POINT('Ctrl Pts',(0.212170950879785,0.672666614098168,
-4.09890768628963));
#50862=CARTESIAN_POINT('Ctrl Pts',(-0.135035171633647,0.692287793147759,
-4.08305017571368));
#50863=CARTESIAN_POINT('Ctrl Pts',(-0.449415441152957,0.543619947548669,
-4.06719266513775));
#50864=CARTESIAN_POINT('Ctrl Pts',(-0.63857363386037,0.28466957177687,-4.05256994710618));
#50865=CARTESIAN_POINT('Ctrl Pts',(-0.676611046385397,0.0861029950325273,
-4.04323306593326));
#50866=CARTESIAN_POINT('Ctrl Pts',(-0.676698966456529,-1.74541653144393E-5,
-4.039182021619));
#50867=CARTESIAN_POINT('Origin',(0.,0.,-6.17861797838101));
#50868=CARTESIAN_POINT('',(-0.676740262348679,-1.17706457744123E-5,-4.478617978381));
#50869=CARTESIAN_POINT('',(-0.676644019679501,-4.3116399903731E-6,-4.439182021619));
#50870=CARTESIAN_POINT('',(-0.6767,7.27977111083166E-14,-6.17861797838101));
#50871=CARTESIAN_POINT('Ctrl Pts',(-0.676740262348678,-1.17706457744317E-5,
-4.478617978381));
#50872=CARTESIAN_POINT('Ctrl Pts',(-0.676750346481431,-0.0124025401036787,
-4.47803502279425));
#50873=CARTESIAN_POINT('Ctrl Pts',(-0.673394647811649,-0.137138751468068,
-4.47216623034886));
#50874=CARTESIAN_POINT('Ctrl Pts',(-0.600161619846482,-0.370544083537301,
-4.46101160104481));
#50875=CARTESIAN_POINT('Ctrl Pts',(-0.350158990608888,-0.61227899610963,
-4.44515409046887));
#50876=CARTESIAN_POINT('Ctrl Pts',(-0.0150358152851096,-0.705174313230397,
-4.42929657989292));
#50877=CARTESIAN_POINT('Ctrl Pts',(0.32374243342603,-0.626648006923061,
-4.41343906931699));
#50878=CARTESIAN_POINT('Ctrl Pts',(0.583821766891339,-0.39578912603194,
-4.39758155874103));
#50879=CARTESIAN_POINT('Ctrl Pts',(0.701979205024536,-0.0687174176928368,
-4.3817240481651));
#50880=CARTESIAN_POINT('Ctrl Pts',(0.649491722206451,0.275058885634601,
-4.36586653758914));
#50881=CARTESIAN_POINT('Ctrl Pts',(0.439118560152959,0.551970812553023,
-4.35000902701321));
#50882=CARTESIAN_POINT('Ctrl Pts',(0.121999569378052,0.694703528746487,
-4.33415151643726));
#50883=CARTESIAN_POINT('Ctrl Pts',(-0.224776435057083,0.668559976385276,
-4.31829400586132));
#50884=CARTESIAN_POINT('Ctrl Pts',(-0.516911281011339,0.479895421258078,
-4.30243649528538));
#50885=CARTESIAN_POINT('Ctrl Pts',(-0.65575605607782,0.225252701430372,
-4.28921115279194));
#50886=CARTESIAN_POINT('Ctrl Pts',(-0.676641787209029,0.0564272013647705,
-4.28127164715715));
#50887=CARTESIAN_POINT('Ctrl Pts',(-0.676642404370006,-2.12118767984465E-7,
-4.27861797838101));
#50888=CARTESIAN_POINT('Ctrl Pts',(-0.676644019679501,-4.31163999035922E-6,
-4.439182021619));
#50889=CARTESIAN_POINT('Ctrl Pts',(-0.676655503400418,-0.0515095321842119,
-4.43675981720748));
#50890=CARTESIAN_POINT('Ctrl Pts',(-0.658181313981681,-0.215403514966007,
-4.42905177593732));
#50891=CARTESIAN_POINT('Ctrl Pts',(-0.527256376882394,-0.468505708776717,
-4.41605789780849));
#50892=CARTESIAN_POINT('Ctrl Pts',(-0.239306432604977,-0.663497790074244,
-4.40020038723256));
#50893=CARTESIAN_POINT('Ctrl Pts',(0.106816783733375,-0.697199441216343,
-4.38434287665661));
#50894=CARTESIAN_POINT('Ctrl Pts',(0.426973786990221,-0.561418089611258,
-4.36848536608067));
#50895=CARTESIAN_POINT('Ctrl Pts',(0.64333724820522,-0.289160977988487,
-4.35262785550472));
#50896=CARTESIAN_POINT('Ctrl Pts',(0.703311128248571,0.0533886036645251,
-4.33677034492878));
#50897=CARTESIAN_POINT('Ctrl Pts',(0.592316308613785,0.382959889113288,
-4.32091283435284));
#50898=CARTESIAN_POINT('Ctrl Pts',(0.337334645867288,0.619437020864201,
-4.3050553237769));
#50899=CARTESIAN_POINT('Ctrl Pts',(0.000349921539867571,0.7053345048092,
-4.28919781320095));
#50900=CARTESIAN_POINT('Ctrl Pts',(-0.336719865611468,0.619771424173557,
-4.27334030262501));
#50901=CARTESIAN_POINT('Ctrl Pts',(-0.591936038811396,0.383547405252334,
-4.25748279204906));
#50902=CARTESIAN_POINT('Ctrl Pts',(-0.671867885490126,0.146986079704804,
-4.2460966983804));
#50903=CARTESIAN_POINT('Ctrl Pts',(-0.676743403478689,0.0173264837064653,
-4.23999644157037));
#50904=CARTESIAN_POINT('Ctrl Pts',(-0.676726753762749,1.49205000514446E-5,
-4.239182021619));
#50905=CARTESIAN_POINT('Origin',(0.,0.,-6.17861797838101));
#50906=CARTESIAN_POINT('',(-0.676683918556463,1.70183238131909E-5,-4.678617978381));
#50907=CARTESIAN_POINT('',(-0.67675000022537,-8.01283250001505E-6,-4.639182021619));
#50908=CARTESIAN_POINT('',(-0.6767,7.27977111083166E-14,-6.17861797838101));
#50909=CARTESIAN_POINT('Ctrl Pts',(-0.676683918556463,1.7018323813206E-5,
-4.678617978381));
#50910=CARTESIAN_POINT('Ctrl Pts',(-0.676606241781625,-0.0811879617933027,
-4.67479839843136));
#50911=CARTESIAN_POINT('Ctrl Pts',(-0.64172719032616,-0.274835745774313,
-4.66569298162307));
#50912=CARTESIAN_POINT('Ctrl Pts',(-0.461166638918949,-0.533687379398699,
-4.65130172795613));
#50913=CARTESIAN_POINT('Ctrl Pts',(-0.15010410398989,-0.689177513958953,
-4.63544421738019));
#50914=CARTESIAN_POINT('Ctrl Pts',(0.197447407787028,-0.677134705165401,
-4.61958670680424));
#50915=CARTESIAN_POINT('Ctrl Pts',(0.497001205311606,-0.500486453063479,
-4.6037291962283));
#50916=CARTESIAN_POINT('Ctrl Pts',(0.675738416267745,-0.202174381565054,
-4.58787168565236));
#50917=CARTESIAN_POINT('Ctrl Pts',(0.690209609366951,0.145284489601514,
-4.57201417507641));
#50918=CARTESIAN_POINT('Ctrl Pts',(0.536896965869284,0.457425989447045,
-4.55615666450047));
#50919=CARTESIAN_POINT('Ctrl Pts',(0.253069430129838,0.658371286824547,
-4.54029915392453));
#50920=CARTESIAN_POINT('Ctrl Pts',(-0.0922770403452622,0.699272361534738,
-4.52444164334858));
#50921=CARTESIAN_POINT('Ctrl Pts',(-0.415191780446262,0.570186524946981,
-4.50858413277264));
#50922=CARTESIAN_POINT('Ctrl Pts',(-0.629016431300928,0.312334364230696,
-4.49330957778344));
#50923=CARTESIAN_POINT('Ctrl Pts',(-0.67665891056109,0.0999483617424532,
-4.4833208596529));
#50924=CARTESIAN_POINT('Ctrl Pts',(-0.676740262348678,-1.17706457744317E-5,
-4.478617978381));
#50925=CARTESIAN_POINT('Ctrl Pts',(-0.67675000022537,-8.01283250002199E-6,
-4.639182021619));
#50926=CARTESIAN_POINT('Ctrl Pts',(-0.676754741008023,-0.00793565612024164,
-4.63880902970323));
#50927=CARTESIAN_POINT('Ctrl Pts',(-0.674685149586979,-0.128207033147944,
-4.63315020092882));
#50928=CARTESIAN_POINT('Ctrl Pts',(-0.607376188029295,-0.358595945786518,
-4.62220553529577));
#50929=CARTESIAN_POINT('Ctrl Pts',(-0.362205792415875,-0.605230410719679,
-4.60634802471981));
#50930=CARTESIAN_POINT('Ctrl Pts',(-0.0289863800046666,-0.704738728816396,
-4.59049051414388));
#50931=CARTESIAN_POINT('Ctrl Pts',(0.311279364390673,-0.632931310194133,
-4.57463300356793));
#50932=CARTESIAN_POINT('Ctrl Pts',(0.575875855124356,-0.407263901671038,
-4.55877549299199));
#50933=CARTESIAN_POINT('Ctrl Pts',(0.700482031227543,-0.0825942494781502,
-4.54291798241604));
#50934=CARTESIAN_POINT('Ctrl Pts',(0.654807236055464,0.262153332477254,
-4.5270604718401));
#50935=CARTESIAN_POINT('Ctrl Pts',(0.449954607358944,0.543173763574772,
-4.51120296126416));
#50936=CARTESIAN_POINT('Ctrl Pts',(0.13572200293829,0.692153468558775,-4.49534545068821));
#50937=CARTESIAN_POINT('Ctrl Pts',(-0.211503417077158,0.672876802010746,
-4.47948794011228));
#50938=CARTESIAN_POINT('Ctrl Pts',(-0.507314231603265,0.49002975066042,
-4.46363042953633));
#50939=CARTESIAN_POINT('Ctrl Pts',(-0.653454360935392,0.234185989462344,
-4.4501951233719));
#50940=CARTESIAN_POINT('Ctrl Pts',(-0.676630443139192,0.0608873373247691,
-4.44204565406613));
#50941=CARTESIAN_POINT('Ctrl Pts',(-0.676644019679501,-4.31163999035922E-6,
-4.439182021619));
#50942=CARTESIAN_POINT('Origin',(0.,0.,-6.17861797838101));
#50943=CARTESIAN_POINT('',(-0.676666391545702,-1.46161483497048E-5,-4.878617978381));
#50944=CARTESIAN_POINT('',(-0.676671450604501,1.55654194976124E-5,-4.839182021619));
#50945=CARTESIAN_POINT('',(-0.6767,7.27977111083166E-14,-6.17861797838101));
#50946=CARTESIAN_POINT('Ctrl Pts',(-0.676666391545702,-1.46161483497304E-5,
-4.87861797838101));
#50947=CARTESIAN_POINT('Ctrl Pts',(-0.676696108666216,-0.0376557552017236,
-4.87684761092712));
#50948=CARTESIAN_POINT('Ctrl Pts',(-0.664388562722288,-0.187663893074887,
-4.86979140661458));
#50949=CARTESIAN_POINT('Ctrl Pts',(-0.555025881375534,-0.435250684990344,
-4.85744936544339));
#50950=CARTESIAN_POINT('Ctrl Pts',(-0.279590796199469,-0.647553761831247,
-4.84159185486746));
#50951=CARTESIAN_POINT('Ctrl Pts',(0.0638103326637412,-0.702442260421875,
-4.8257343442915));
#50952=CARTESIAN_POINT('Ctrl Pts',(0.391699735402671,-0.586573273399606,
-4.80987683371557));
#50953=CARTESIAN_POINT('Ctrl Pts',(0.624370405298808,-0.32811352420809,
-4.79401932313962));
#50954=CARTESIAN_POINT('Ctrl Pts',(0.705262165372666,0.0101077136440157,
-4.77816181256367));
#50955=CARTESIAN_POINT('Ctrl Pts',(0.614710945941539,0.345871855924866,
-4.76230430198774));
#50956=CARTESIAN_POINT('Ctrl Pts',(0.374728945616527,0.597557616551221,
-4.74644679141179));
#50957=CARTESIAN_POINT('Ctrl Pts',(0.0436536609816854,0.703982418576024,
-4.73058928083585));
#50958=CARTESIAN_POINT('Ctrl Pts',(-0.298033441601801,0.639275336195787,
-4.71473177025991));
#50959=CARTESIAN_POINT('Ctrl Pts',(-0.567271256914447,0.419166087440235,
-4.69887425968396));
#50960=CARTESIAN_POINT('Ctrl Pts',(-0.666974939736738,0.17472219918873,
-4.68683632905766));
#50961=CARTESIAN_POINT('Ctrl Pts',(-0.676713737046788,0.0311899129122367,
-4.68008423529001));
#50962=CARTESIAN_POINT('Ctrl Pts',(-0.676683918556463,1.7018323813206E-5,
-4.678617978381));
#50963=CARTESIAN_POINT('Ctrl Pts',(-0.676671450604501,1.55654194976401E-5,
-4.839182021619));
#50964=CARTESIAN_POINT('Ctrl Pts',(-0.67660621972088,-0.076729606307988,
-4.83557240534034));
#50965=CARTESIAN_POINT('Ctrl Pts',(-0.64448073360313,-0.265911822706924,
-4.82667695220303));
#50966=CARTESIAN_POINT('Ctrl Pts',(-0.471636589224496,-0.524457637778504,
-4.81249566220709));
#50967=CARTESIAN_POINT('Ctrl Pts',(-0.163711689954952,-0.686072422337189,
-4.79663815163114));
#50968=CARTESIAN_POINT('Ctrl Pts',(0.184010069664874,-0.680909083785385,
-4.7807806410552));
#50969=CARTESIAN_POINT('Ctrl Pts',(0.487000612793599,-0.510222783946564,
-4.76492313047925));
#50970=CARTESIAN_POINT('Ctrl Pts',(0.671605624729155,-0.215505848996464,
-4.74906561990332));
#50971=CARTESIAN_POINT('Ctrl Pts',(0.692949263789228,0.131598647156757,
-4.73320810932736));
#50972=CARTESIAN_POINT('Ctrl Pts',(0.545843080552321,0.446712678947753,
-4.71735059875143));
#50973=CARTESIAN_POINT('Ctrl Pts',(0.266047283910979,0.653234819068239,
-4.70149308817548));
#50974=CARTESIAN_POINT('Ctrl Pts',(-0.0784222486577756,0.700961366292738,
-4.68563557759954));
#50975=CARTESIAN_POINT('Ctrl Pts',(-0.403828027874236,0.578290420137434,
-4.66977806702359));
#50976=CARTESIAN_POINT('Ctrl Pts',(-0.625721804684535,0.321234184394516,
-4.65429354836342));
#50977=CARTESIAN_POINT('Ctrl Pts',(-0.676687557236402,0.104410556549851,
-4.64409486656188));
#50978=CARTESIAN_POINT('Ctrl Pts',(-0.67675000022537,-8.01283250002199E-6,
-4.639182021619));
#50979=CARTESIAN_POINT('Origin',(0.,0.,-6.17861797838101));
#50980=CARTESIAN_POINT('',(-0.67675329042481,6.10867791108173E-6,-5.078617978381));
#50981=CARTESIAN_POINT('',(-0.67667814830283,-1.64852909755597E-5,-5.039182021619));
#50982=CARTESIAN_POINT('',(-0.6767,7.27977111083166E-14,-6.17861797838101));
#50983=CARTESIAN_POINT('Ctrl Pts',(-0.67675329042481,6.10867791109304E-6,
-5.078617978381));
#50984=CARTESIAN_POINT('Ctrl Pts',(-0.676702849224836,-0.106411973995982,
-5.07361098656422));
#50985=CARTESIAN_POINT('Ctrl Pts',(-0.624209800255466,-0.325222693532886,
-5.06331815788879));
#50986=CARTESIAN_POINT('Ctrl Pts',(-0.398680950495202,-0.581850829245344,
-5.04773949235472));
#50987=CARTESIAN_POINT('Ctrl Pts',(-0.0721995192170595,-0.701629615399804,
-5.03188198177877));
#50988=CARTESIAN_POINT('Ctrl Pts',(0.271832975057436,-0.650848462741271,
-5.01602447120283));
#50989=CARTESIAN_POINT('Ctrl Pts',(0.549785283183103,-0.441851819252255,
-5.00016696062688));
#50990=CARTESIAN_POINT('Ctrl Pts',(0.694089663396602,-0.125444915988027,
-4.98430945005094));
#50991=CARTESIAN_POINT('Ctrl Pts',(0.669667000279414,0.221456534150661,
-4.968451939475));
#50992=CARTESIAN_POINT('Ctrl Pts',(0.482454226702515,0.514523864284379,
-4.95259442889905));
#50993=CARTESIAN_POINT('Ctrl Pts',(0.177961108082654,0.682515004810329,
-4.93673691832311));
#50994=CARTESIAN_POINT('Ctrl Pts',(-0.169792778098127,0.684592798886295,
-4.92087940774717));
#50995=CARTESIAN_POINT('Ctrl Pts',(-0.476271545316318,0.520252153194254,
-4.90502189717122));
#50996=CARTESIAN_POINT('Ctrl Pts',(-0.645682600184146,0.261909416791567,
-4.89093475404917));
#50997=CARTESIAN_POINT('Ctrl Pts',(-0.676607381407591,0.0747304727380146,
-4.88213344778577));
#50998=CARTESIAN_POINT('Ctrl Pts',(-0.676666391545702,-1.46161483497304E-5,
-4.87861797838101));
#50999=CARTESIAN_POINT('Ctrl Pts',(-0.67667814830283,-1.64852909755875E-5,
-5.039182021619));
#51000=CARTESIAN_POINT('Ctrl Pts',(-0.676708467968247,-0.0331917720224041,
-5.03762161783609));
#51001=CARTESIAN_POINT('Ctrl Pts',(-0.666195069508018,-0.178728635692127,
-5.03077537719454));
#51002=CARTESIAN_POINT('Ctrl Pts',(-0.563529656794226,-0.424182993568702,
-5.01864329969435));
#51003=CARTESIAN_POINT('Ctrl Pts',(-0.292349407557091,-0.641894625324549,
-5.00278578911841));
#51004=CARTESIAN_POINT('Ctrl Pts',(0.0498983906696054,-0.703567364740653,
-4.98692827854246));
#51005=CARTESIAN_POINT('Ctrl Pts',(0.380016332526679,-0.594209115659208,
-4.97107076796653));
#51006=CARTESIAN_POINT('Ctrl Pts',(0.617755673194353,-0.340403898855044,
-4.95521325739056));
#51007=CARTESIAN_POINT('Ctrl Pts',(0.705324086767725,-0.00384951228082019,
-4.93935574681464));
#51008=CARTESIAN_POINT('Ctrl Pts',(0.621434468293966,0.333640656598862,
-4.92349823623868));
#51009=CARTESIAN_POINT('Ctrl Pts',(0.386479640253609,0.590025739937645,
-4.90764072566275));
#51010=CARTESIAN_POINT('Ctrl Pts',(0.0575750382195188,0.702980797101559,
-4.8917832150868));
#51011=CARTESIAN_POINT('Ctrl Pts',(-0.285325545141958,0.645047455160447,
-4.87592570451086));
#51012=CARTESIAN_POINT('Ctrl Pts',(-0.558866018193005,0.430308795899666,
-4.86006819393491));
#51013=CARTESIAN_POINT('Ctrl Pts',(-0.665210108609933,0.183657329584508,
-4.84782029963763));
#51014=CARTESIAN_POINT('Ctrl Pts',(-0.676701742286812,0.0356542112847855,
-4.84085824219899));
#51015=CARTESIAN_POINT('Ctrl Pts',(-0.676671450604501,1.55654194976401E-5,
-4.839182021619));
#51016=CARTESIAN_POINT('Origin',(0.,0.,-6.17861797838101));
#51017=CARTESIAN_POINT('',(-0.676645685622293,6.08692033333708E-6,-5.278617978381));
#51018=CARTESIAN_POINT('',(-0.676744992161023,1.01792954273136E-5,-5.239182021619));
#51019=CARTESIAN_POINT('',(-0.6767,7.27977111083166E-14,-6.17861797838101));
#51020=CARTESIAN_POINT('Ctrl Pts',(-0.676645685622293,6.08692033332928E-6,
-5.278617978381));
#51021=CARTESIAN_POINT('Ctrl Pts',(-0.676625829214806,-0.0628870377702795,
-5.27566019905998));
#51022=CARTESIAN_POINT('Ctrl Pts',(-0.652390634777465,-0.238191234465806,
-5.2674165828803));
#51023=CARTESIAN_POINT('Ctrl Pts',(-0.502946219016085,-0.49451186897655,
-5.25388712984198));
#51024=CARTESIAN_POINT('Ctrl Pts',(-0.205524643813888,-0.674726988171084,
-5.23802961926603));
#51025=CARTESIAN_POINT('Ctrl Pts',(0.141858150105515,-0.690921958711615,
-5.2221721086901));
#51026=CARTESIAN_POINT('Ctrl Pts',(0.454756485457226,-0.539159926845312,
-5.20631459811414));
#51027=CARTESIAN_POINT('Ctrl Pts',(0.65710755109285,-0.256332896987509,
-5.19045708753821));
#51028=CARTESIAN_POINT('Ctrl Pts',(0.699721597013181,0.0888063874649557,
-5.17459957696226));
#51029=CARTESIAN_POINT('Ctrl Pts',(0.572239526473699,0.412357626487503,
-5.15874206638632));
#51030=CARTESIAN_POINT('Ctrl Pts',(0.30565110055879,0.635668382498652,-5.14288455581037));
#51031=CARTESIAN_POINT('Ctrl Pts',(-0.035238397980778,0.704453790598787,
-5.12702704523444));
#51032=CARTESIAN_POINT('Ctrl Pts',(-0.367561754396992,0.601992727934364,
-5.11116953465848));
#51033=CARTESIAN_POINT('Ctrl Pts',(-0.610534107144088,0.353192570413113,
-5.09531202408255));
#51034=CARTESIAN_POINT('Ctrl Pts',(-0.675234784868236,0.124202376260447,
-5.08446150532338));
#51035=CARTESIAN_POINT('Ctrl Pts',(-0.676756099552333,0.00593265216038066,
-5.07889682342287));
#51036=CARTESIAN_POINT('Ctrl Pts',(-0.67675329042481,6.10867791109304E-6,
-5.078617978381));
#51037=CARTESIAN_POINT('Ctrl Pts',(-0.676744992161023,1.01792954273032E-5,
-5.239182021619));
#51038=CARTESIAN_POINT('Ctrl Pts',(-0.67667085383716,-0.101948986768809,
-5.2343849934732));
#51039=CARTESIAN_POINT('Ctrl Pts',(-0.627552308620193,-0.316325790578849,
-5.22430212846876));
#51040=CARTESIAN_POINT('Ctrl Pts',(-0.410116160373992,-0.573848081916823,
-5.20893342660567));
#51041=CARTESIAN_POINT('Ctrl Pts',(-0.0860687518011682,-0.700063608597757,
-5.19307591602972));
#51042=CARTESIAN_POINT('Ctrl Pts',(0.25890120724375,-0.656099878834963,
-5.17721840545379));
#51043=CARTESIAN_POINT('Ctrl Pts',(0.540934578241509,-0.452644085548684,
-5.16136089487784));
#51044=CARTESIAN_POINT('Ctrl Pts',(0.691471549227516,-0.139154528235421,
-5.1455033843019));
#51045=CARTESIAN_POINT('Ctrl Pts',(0.673917917224984,0.208162261139392,
-5.12964587372595));
#51046=CARTESIAN_POINT('Ctrl Pts',(0.492540814542161,0.504876650410443,
-5.11378836315001));
#51047=CARTESIAN_POINT('Ctrl Pts',(0.191431406740854,0.678860002233702,
-5.09793085257407));
#51048=CARTESIAN_POINT('Ctrl Pts',(-0.156213278796698,0.687818506327875,
-5.08207334199812));
#51049=CARTESIAN_POINT('Ctrl Pts',(-0.465883901255171,0.529574429774311,
-5.06621583142218));
#51050=CARTESIAN_POINT('Ctrl Pts',(-0.642974403145626,0.27083467858935,
-5.05191872462914));
#51051=CARTESIAN_POINT('Ctrl Pts',(-0.676605760703141,0.0791888536353506,
-5.04290745469474));
#51052=CARTESIAN_POINT('Ctrl Pts',(-0.67667814830283,-1.64852909755875E-5,
-5.039182021619));
#51053=CARTESIAN_POINT('Origin',(0.,0.,-6.17861797838101));
#51054=CARTESIAN_POINT('',(-0.676720731008515,-1.58587921748656E-5,-5.47861797838101));
#51055=CARTESIAN_POINT('',(-0.676642766387654,2.06514063441632E-6,-5.439182021619));
#51056=CARTESIAN_POINT('',(-0.6767,7.27977111083166E-14,-6.17861797838101));
#51057=CARTESIAN_POINT('Ctrl Pts',(-0.676720731008515,-1.58587921748089E-5,
-5.47861797838101));
#51058=CARTESIAN_POINT('Ctrl Pts',(-0.676739988800954,-0.0193291336136783,
-5.47770941155573));
#51059=CARTESIAN_POINT('Ctrl Pts',(-0.67121548086959,-0.150991703321477,
-5.47151500787181));
#51060=CARTESIAN_POINT('Ctrl Pts',(-0.588509514849396,-0.388784565910968,
-5.46003476732924));
#51061=CARTESIAN_POINT('Ctrl Pts',(-0.331207368228394,-0.622734748534038,
-5.4441772567533));
#51062=CARTESIAN_POINT('Ctrl Pts',(0.00660835310116418,-0.705303634925465,
-5.42831974617736));
#51063=CARTESIAN_POINT('Ctrl Pts',(0.342817642383509,-0.616419460965605,
-5.41246223560141));
#51064=CARTESIAN_POINT('Ctrl Pts',(0.595691002243588,-0.377689181239748,
-5.39660472502547));
#51065=CARTESIAN_POINT('Ctrl Pts',(0.703757160891212,-0.0471460101786735,
-5.38074721444953));
#51066=CARTESIAN_POINT('Ctrl Pts',(0.64074619327961,0.294857937962055,-5.36488970387358));
#51067=CARTESIAN_POINT('Ctrl Pts',(0.421975506976434,0.565184535610204,
-5.34903219329764));
#51068=CARTESIAN_POINT('Ctrl Pts',(0.100626316187652,0.698119783613068,
-5.3331746827217));
#51069=CARTESIAN_POINT('Ctrl Pts',(-0.245184239907299,0.661348301791295,
-5.31731717214575));
#51070=CARTESIAN_POINT('Ctrl Pts',(-0.531392681099133,0.463808911358507,
-5.30145966156981));
#51071=CARTESIAN_POINT('Ctrl Pts',(-0.659134379441101,0.211397173063012,
-5.2885599303149));
#51072=CARTESIAN_POINT('Ctrl Pts',(-0.676661314529693,0.0495090406936801,
-5.28094603591862));
#51073=CARTESIAN_POINT('Ctrl Pts',(-0.676645685622293,6.08692033332928E-6,
-5.278617978381));
#51074=CARTESIAN_POINT('Ctrl Pts',(-0.676642766387654,2.06514063443713E-6,
-5.439182021619));
#51075=CARTESIAN_POINT('Ctrl Pts',(-0.676636540647253,-0.0584271905943807,
-5.43643420596896));
#51076=CARTESIAN_POINT('Ctrl Pts',(-0.654736005126173,-0.229258492031468,
-5.42840055346027));
#51077=CARTESIAN_POINT('Ctrl Pts',(-0.512632811011637,-0.484463091673161,
-5.41508106409294));
#51078=CARTESIAN_POINT('Ctrl Pts',(-0.218835441848411,-0.670528101954526,
-5.39922355351699));
#51079=CARTESIAN_POINT('Ctrl Pts',(0.128158883019949,-0.693593675592924,
-5.38336604294105));
#51080=CARTESIAN_POINT('Ctrl Pts',(0.443998919690547,-0.548052776138566,
-5.3675085323651));
#51081=CARTESIAN_POINT('Ctrl Pts',(0.651906755505725,-0.269285105873896,
-5.35165102178917));
#51082=CARTESIAN_POINT('Ctrl Pts',(0.701341838902262,0.0749433861305649,
-5.33579351121321));
#51083=CARTESIAN_POINT('Ctrl Pts',(0.580286939400919,0.400953805419331,
-5.31993600063728));
#51084=CARTESIAN_POINT('Ctrl Pts',(0.31816942979039,0.62949590949138,-5.30407849006133));
#51085=CARTESIAN_POINT('Ctrl Pts',(-0.0212922472927337,0.705013139114975,
-5.28822097948539));
#51086=CARTESIAN_POINT('Ctrl Pts',(-0.355577967837347,0.609147925308939,
-5.27236346890944));
#51087=CARTESIAN_POINT('Ctrl Pts',(-0.603425836976519,0.365204251602734,
-5.2565059583335));
#51088=CARTESIAN_POINT('Ctrl Pts',(-0.673984377760133,0.13313369579333,
-5.24544547590335));
#51089=CARTESIAN_POINT('Ctrl Pts',(-0.676752546725549,0.0103996386049762,
-5.23967083033185));
#51090=CARTESIAN_POINT('Ctrl Pts',(-0.676744992161023,1.01792954273032E-5,
-5.239182021619));
#51091=CARTESIAN_POINT('Origin',(0.,0.,-6.17861797838101));
#51092=CARTESIAN_POINT('',(-0.676705286336412,1.7378251266052E-5,-5.678617978381));
#51093=CARTESIAN_POINT('',(-0.676733793626987,-1.34876458774968E-5,-5.63918202161899));
#51094=CARTESIAN_POINT('',(-0.6767,7.27977111083166E-14,-6.17861797838101));
#51095=CARTESIAN_POINT('Ctrl Pts',(-0.676705286336412,1.73782512660377E-5,
-5.678617978381));
#51096=CARTESIAN_POINT('Ctrl Pts',(-0.676614630128216,-0.088102164827456,
-5.67447278719284));
#51097=CARTESIAN_POINT('Ctrl Pts',(-0.637255231935198,-0.288668254515342,
-5.66504175914603));
#51098=CARTESIAN_POINT('Ctrl Pts',(-0.444574205494435,-0.547586123312261,
-5.65032489424056));
#51099=CARTESIAN_POINT('Ctrl Pts',(-0.128887172109694,-0.69345876028638,
-5.63446738366463));
#51100=CARTESIAN_POINT('Ctrl Pts',(0.218131180300111,-0.670757513336377,
-5.61860987308867));
#51101=CARTESIAN_POINT('Ctrl Pts',(0.512123781755499,-0.485001168094135,
-5.60275236251274));
#51102=CARTESIAN_POINT('Ctrl Pts',(0.681623629821306,-0.181345284572452,
-5.58689485193679));
#51103=CARTESIAN_POINT('Ctrl Pts',(0.685426818106913,0.166394001985959,
-5.57103734136085));
#51104=CARTESIAN_POINT('Ctrl Pts',(0.522608823274475,0.47368439616164,-5.5551798307849));
#51105=CARTESIAN_POINT('Ctrl Pts',(0.232749257329435,0.665826306056506,
-5.53932232020896));
#51106=CARTESIAN_POINT('Ctrl Pts',(-0.113689589679385,0.69611174793571,
-5.52346480963302));
#51107=CARTESIAN_POINT('Ctrl Pts',(-0.432491505325853,0.557178593751515,
-5.50760729905708));
#51108=CARTESIAN_POINT('Ctrl Pts',(-0.633916371127028,0.298520956886305,
-5.4926583553064));
#51109=CARTESIAN_POINT('Ctrl Pts',(-0.676627951308215,0.0930311431135412,
-5.48299524841438));
#51110=CARTESIAN_POINT('Ctrl Pts',(-0.676720731008515,-1.58587921748089E-5,
-5.47861797838101));
#51111=CARTESIAN_POINT('Ctrl Pts',(-0.676733793626987,-1.34876458775003E-5,
-5.639182021619));
#51112=CARTESIAN_POINT('Ctrl Pts',(-0.676747142672881,-0.0148627663377926,
-5.63848341846471));
#51113=CARTESIAN_POINT('Ctrl Pts',(-0.672645515489534,-0.142058689415187,
-5.63249897845178));
#51114=CARTESIAN_POINT('Ctrl Pts',(-0.596087294840688,-0.377063422523974,
-5.6212287015802));
#51115=CARTESIAN_POINT('Ctrl Pts',(-0.343464771761306,-0.61605911690008,
-5.60537119100425));
#51116=CARTESIAN_POINT('Ctrl Pts',(-0.00734900831199806,-0.705296305700142,
-5.58951368042832));
#51117=CARTESIAN_POINT('Ctrl Pts',(0.330553234139647,-0.623082213877371,
-5.57365616985237));
#51118=CARTESIAN_POINT('Ctrl Pts',(0.588100915954884,-0.389402361121922,
-5.55779865927643));
#51119=CARTESIAN_POINT('Ctrl Pts',(0.70268647930235,-0.0610622463428964,
-5.54194114870048));
#51120=CARTESIAN_POINT('Ctrl Pts',(0.646455189560342,0.282121558884655,
-5.52608363812454));
#51121=CARTESIAN_POINT('Ctrl Pts',(0.433076374763486,0.556724114585172,
-5.5102261275486));
#51122=CARTESIAN_POINT('Ctrl Pts',(0.114420532934634,0.695991973912722,
-5.49436861697265));
#51123=CARTESIAN_POINT('Ctrl Pts',(-0.232049925986955,0.666070355123448,
-5.47851110639671));
#51124=CARTESIAN_POINT('Ctrl Pts',(-0.522111105272023,0.47423293840623,
-5.46265359582076));
#51125=CARTESIAN_POINT('Ctrl Pts',(-0.656982431274472,0.22033182852696,
-5.44954390089486));
#51126=CARTESIAN_POINT('Ctrl Pts',(-0.676648516795683,0.0539702744914142,
-5.4417200428276));
#51127=CARTESIAN_POINT('Ctrl Pts',(-0.676642766387654,2.06514063443713E-6,
-5.439182021619));
#51128=CARTESIAN_POINT('Origin',(1.87869726832665E-16,-4.25270154953079E-17,
-0.0711000000000004));
#51129=CARTESIAN_POINT('',(0.533647856309002,-0.584002718706691,-0.0711000000000004));
#51130=CARTESIAN_POINT('Ctrl Pts',(-0.657933807534666,-0.158364149874852,
-0.0710999999999999));
#51131=CARTESIAN_POINT('Ctrl Pts',(-0.655067175170568,-0.176843370863458,
-0.0711));
#51132=CARTESIAN_POINT('Ctrl Pts',(-0.651433858321437,-0.195176279166223,
-0.0711000000000002));
#51133=CARTESIAN_POINT('Ctrl Pts',(-0.647039750703694,-0.213314001327678,
-0.0711000000000001));
#51134=CARTESIAN_POINT('Ctrl Pts',(-0.640230933967416,-0.241419008522359,
-0.0711));
#51135=CARTESIAN_POINT('Ctrl Pts',(-0.63159703034734,-0.269055704981072,
-0.0711000000000006));
#51136=CARTESIAN_POINT('Ctrl Pts',(-0.621244545257689,-0.296079436761064,
-0.0711000000000008));
#51137=CARTESIAN_POINT('Ctrl Pts',(-0.617380417573146,-0.306166208121415,
-0.0711000000000009));
#51138=CARTESIAN_POINT('Ctrl Pts',(-0.613276543861295,-0.316167552672532,
-0.0710999999999993));
#51139=CARTESIAN_POINT('Ctrl Pts',(-0.608937382020534,-0.32607575008205,
-0.0710999999999992));
#51140=CARTESIAN_POINT('Ctrl Pts',(-0.605509041370034,-0.333904145795049,
-0.0710999999999991));
#51141=CARTESIAN_POINT('Ctrl Pts',(-0.601935083523056,-0.341671178642489,
-0.0710999999999995));
#51142=CARTESIAN_POINT('Ctrl Pts',(-0.598222557587975,-0.349364132086584,
-0.0710999999999997));
#51143=CARTESIAN_POINT('Ctrl Pts',(-0.583545036283053,-0.37977832717853,
-0.0711000000000002));
#51144=CARTESIAN_POINT('Ctrl Pts',(-0.566687660332639,-0.409077303745793,
-0.0711000000000005));
#51145=CARTESIAN_POINT('Ctrl Pts',(-0.547808142714083,-0.437035513090251,
-0.0711000000000012));
#51146=CARTESIAN_POINT('Ctrl Pts',(-0.540578555953244,-0.447741628798144,
-0.0711000000000015));
#51147=CARTESIAN_POINT('Ctrl Pts',(-0.533051911273803,-0.458251009655921,
-0.0711000000000012));
#51148=CARTESIAN_POINT('Ctrl Pts',(-0.525235161508019,-0.468550294116621,
-0.0711000000000016));
#51149=CARTESIAN_POINT('Ctrl Pts',(-0.520149637961148,-0.475250937633454,
-0.0711000000000018));
#51150=CARTESIAN_POINT('Ctrl Pts',(-0.514940349991532,-0.481863803139074,
-0.0711000000000006));
#51151=CARTESIAN_POINT('Ctrl Pts',(-0.50961195342397,-0.488381464082369,
-0.0711000000000006));
#51152=CARTESIAN_POINT('Ctrl Pts',(-0.50174268945366,-0.498007097944534,
-0.0711000000000006));
#51153=CARTESIAN_POINT('Ctrl Pts',(-0.493626185487008,-0.507409974947679,
-0.0711000000000007));
#51154=CARTESIAN_POINT('Ctrl Pts',(-0.485270890711584,-0.516579714254148,
-0.0711000000000008));
#51155=CARTESIAN_POINT('Ctrl Pts',(-0.462359319831774,-0.541724623885286,
-0.0711000000000012));
#51156=CARTESIAN_POINT('Ctrl Pts',(-0.437655716777344,-0.565118419515218,
-0.0711000000000013));
#51157=CARTESIAN_POINT('Ctrl Pts',(-0.411418393873527,-0.586660131434357,
-0.0711000000000024));
#51158=CARTESIAN_POINT('Ctrl Pts',(-0.384942907216212,-0.608397383690681,
-0.0711000000000035));
#51159=CARTESIAN_POINT('Ctrl Pts',(-0.356904820962166,-0.628249603900737,
-0.0711));
#51160=CARTESIAN_POINT('Ctrl Pts',(-0.327527570258942,-0.646080286484725,
-0.0710999999999997));
#51161=CARTESIAN_POINT('Ctrl Pts',(-0.318239054031453,-0.651718002083155,
-0.0710999999999996));
#51162=CARTESIAN_POINT('Ctrl Pts',(-0.308816404956276,-0.657153329266888,
-0.0711000000000009));
#51163=CARTESIAN_POINT('Ctrl Pts',(-0.299266053289952,-0.662381069497827,
-0.0711000000000009));
#51164=CARTESIAN_POINT('Ctrl Pts',(-0.29268155396986,-0.665985340125641,
-0.0711000000000009));
#51165=CARTESIAN_POINT('Ctrl Pts',(-0.286043387081773,-0.66948701230259,
-0.0711000000000016));
#51166=CARTESIAN_POINT('Ctrl Pts',(-0.279358582158395,-0.672882728805687,
-0.0711000000000016));
#51167=CARTESIAN_POINT('Ctrl Pts',(-0.249273658782167,-0.688165130008715,
-0.0711000000000017));
#51168=CARTESIAN_POINT('Ctrl Pts',(-0.218218521949027,-0.701319368658359,
-0.0711000000000021));
#51169=CARTESIAN_POINT('Ctrl Pts',(-0.186415735009314,-0.712239574350195,
-0.0711000000000015));
#51170=CARTESIAN_POINT('Ctrl Pts',(-0.156944284161696,-0.722359263102722,
-0.071100000000001));
#51171=CARTESIAN_POINT('Ctrl Pts',(-0.12682988518337,-0.730560652357132,
-0.0711000000000014));
#51172=CARTESIAN_POINT('Ctrl Pts',(-0.0962629225125643,-0.736850720931549,
-0.0711000000000013));
#51173=CARTESIAN_POINT('Ctrl Pts',(-0.078716983307866,-0.74046132372479,
-0.0711000000000012));
#51174=CARTESIAN_POINT('Ctrl Pts',(-0.0610216276845667,-0.743441599523475,
-0.0711000000000011));
#51175=CARTESIAN_POINT('Ctrl Pts',(-0.0432113397414346,-0.745788198486428,
-0.0711000000000013));
#51176=CARTESIAN_POINT('Ctrl Pts',(-0.0322456473157928,-0.747232986047204,
-0.0711000000000014));
#51177=CARTESIAN_POINT('Ctrl Pts',(-0.0212297038631688,-0.748437831918465,
-0.0711000000000008));
#51178=CARTESIAN_POINT('Ctrl Pts',(-0.0102078164611569,-0.749398841582625,
-0.0711000000000007));
#51179=CARTESIAN_POINT('Ctrl Pts',(0.0255783266149804,-0.752519072091687,
-0.0711000000000004));
#51180=CARTESIAN_POINT('Ctrl Pts',(0.0614807257563876,-0.753082924998665,
-0.0711000000000016));
#51181=CARTESIAN_POINT('Ctrl Pts',(0.0972146459662916,-0.751115790681787,
-0.0711000000000007));
#51182=CARTESIAN_POINT('Ctrl Pts',(0.126022429919159,-0.749529936678811,
-0.0711000000000001));
#51183=CARTESIAN_POINT('Ctrl Pts',(0.154721556272749,-0.746298281511085,
-0.0710999999999997));
#51184=CARTESIAN_POINT('Ctrl Pts',(0.183168524859653,-0.741410164954474,
-0.0710999999999994));
#51185=CARTESIAN_POINT('Ctrl Pts',(0.199846793288582,-0.738544294737266,
-0.0710999999999992));
#51186=CARTESIAN_POINT('Ctrl Pts',(0.216438437569116,-0.73510861830928,
-0.0710999999999984));
#51187=CARTESIAN_POINT('Ctrl Pts',(0.232919227747053,-0.731115468971878,
-0.0710999999999985));
#51188=CARTESIAN_POINT('Ctrl Pts',(0.241823558807982,-0.72895802850379,
-0.0710999999999985));
#51189=CARTESIAN_POINT('Ctrl Pts',(0.250695524136604,-0.72663781184377,
-0.0711000000000005));
#51190=CARTESIAN_POINT('Ctrl Pts',(0.25953123057737,-0.724156453648781,
-0.0711000000000006));
#51191=CARTESIAN_POINT('Ctrl Pts',(0.266656117644727,-0.722155550038926,
-0.0711000000000008));
#51192=CARTESIAN_POINT('Ctrl Pts',(0.27375672049831,-0.720049926629994,
-0.0711000000000007));
#51193=CARTESIAN_POINT('Ctrl Pts',(0.280818325570169,-0.717844754206751,
-0.0711000000000006));
#51194=CARTESIAN_POINT('Ctrl Pts',(0.315496365708099,-0.70701562159085,
-0.0711000000000003));
#51195=CARTESIAN_POINT('Ctrl Pts',(0.349314461131609,-0.693768119967408,
-0.0710999999999986));
#51196=CARTESIAN_POINT('Ctrl Pts',(0.382044763390059,-0.678267148964668,
-0.0710999999999989));
#51197=CARTESIAN_POINT('Ctrl Pts',(0.415042655619168,-0.662639448170585,
-0.0710999999999991));
#51198=CARTESIAN_POINT('Ctrl Pts',(0.446936060969254,-0.644720926130431,
-0.0710999999999995));
#51199=CARTESIAN_POINT('Ctrl Pts',(0.477482228286911,-0.624629210095727,
-0.0710999999999994));
#51200=CARTESIAN_POINT('Ctrl Pts',(0.496763176301389,-0.611947182646645,
-0.0710999999999993));
#51201=CARTESIAN_POINT('Ctrl Pts',(0.51550711528861,-0.598398299343742,
-0.0711000000000005));
#51202=CARTESIAN_POINT('Ctrl Pts',(0.533647856309002,-0.584002718706691,
-0.0711000000000004));
#51203=CARTESIAN_POINT('',(-0.7911,-9.68818082805472E-17,-0.0711000000000002));
#51204=CARTESIAN_POINT('Origin',(0.,0.,-0.0711000000000004));
#51205=CARTESIAN_POINT('',(0.789514313045754,0.0505148300805575,-0.0711000000000008));
#51206=CARTESIAN_POINT('Origin',(0.,0.,-0.0711000000000004));
#51207=CARTESIAN_POINT('Ctrl Pts',(0.789514313045754,0.0505148300805575,
-0.0711000000000008));
#51208=CARTESIAN_POINT('Ctrl Pts',(0.786646978061939,0.0720310274345683,
-0.0711000000000009));
#51209=CARTESIAN_POINT('Ctrl Pts',(0.782893056548073,0.0933955551493298,
-0.0711000000000011));
#51210=CARTESIAN_POINT('Ctrl Pts',(0.778246937672325,0.114553731850933,
-0.0711000000000015));
#51211=CARTESIAN_POINT('Ctrl Pts',(0.771351411757343,0.145955587821779,
-0.071100000000002));
#51212=CARTESIAN_POINT('Ctrl Pts',(0.762491759243552,0.176903771447525,
-0.0711000000000021));
#51213=CARTESIAN_POINT('Ctrl Pts',(0.751744397702525,0.207227273368498,
-0.0711000000000022));
#51214=CARTESIAN_POINT('Ctrl Pts',(0.747529533840752,0.219119441685457,
-0.0711000000000022));
#51215=CARTESIAN_POINT('Ctrl Pts',(0.743024048428749,0.2309153715258,-0.0711000000000015));
#51216=CARTESIAN_POINT('Ctrl Pts',(0.738231505771285,0.242604011376074,
-0.0711000000000015));
#51217=CARTESIAN_POINT('Ctrl Pts',(0.734846385381388,0.250860057470042,
-0.0711000000000016));
#51218=CARTESIAN_POINT('Ctrl Pts',(0.731318354610578,0.259061428072549,
-0.0711000000000027));
#51219=CARTESIAN_POINT('Ctrl Pts',(0.727654054345844,0.267193088850121,
-0.0711000000000026));
#51220=CARTESIAN_POINT('Ctrl Pts',(0.712237780878605,0.30140423347065,-0.0711000000000021));
#51221=CARTESIAN_POINT('Ctrl Pts',(0.694391329924917,0.334439112533965,
-0.0711000000000008));
#51222=CARTESIAN_POINT('Ctrl Pts',(0.674232315159198,0.366018489702608,
-0.0711000000000009));
#51223=CARTESIAN_POINT('Ctrl Pts',(0.661954695941359,0.385251551065925,
-0.071100000000001));
#51224=CARTESIAN_POINT('Ctrl Pts',(0.64881830561573,0.403944116210025,-0.0711000000000001));
#51225=CARTESIAN_POINT('Ctrl Pts',(0.634841970653168,0.422025133375404,
-0.0710999999999997));
#51226=CARTESIAN_POINT('Ctrl Pts',(0.629531677098083,0.428894996553405,
-0.0710999999999995));
#51227=CARTESIAN_POINT('Ctrl Pts',(0.624104492788437,0.435670645433795,
-0.0711000000000013));
#51228=CARTESIAN_POINT('Ctrl Pts',(0.618566742729686,0.442342896181215,
-0.0711000000000013));
#51229=CARTESIAN_POINT('Ctrl Pts',(0.614748344734689,0.44694355684769,-0.0711000000000013));
#51230=CARTESIAN_POINT('Ctrl Pts',(0.610876694281843,0.451495942259902,
-0.0711000000000009));
#51231=CARTESIAN_POINT('Ctrl Pts',(0.606952317219739,0.455998969182275,
-0.0711000000000009));
#51232=CARTESIAN_POINT('Ctrl Pts',(0.583540589687488,0.48286275869808,-0.071100000000001));
#51233=CARTESIAN_POINT('Ctrl Pts',(0.558255129692067,0.507973159032313,
-0.0711000000000011));
#51234=CARTESIAN_POINT('Ctrl Pts',(0.531324903596647,0.53118307146707,-0.0711000000000014));
#51235=CARTESIAN_POINT('Ctrl Pts',(0.504630859305665,0.554189429762315,
-0.0711000000000016));
#51236=CARTESIAN_POINT('Ctrl Pts',(0.47631965093766,0.575329052982221,-0.0711000000000001));
#51237=CARTESIAN_POINT('Ctrl Pts',(0.446590446866821,0.59441407859226,-0.0711));
#51238=CARTESIAN_POINT('Ctrl Pts',(0.437640726063256,0.60015946115722,-0.0711));
#51239=CARTESIAN_POINT('Ctrl Pts',(0.428562395620676,0.605718303647675,
-0.0710999999999995));
#51240=CARTESIAN_POINT('Ctrl Pts',(0.419360692132523,0.611084560737194,
-0.0710999999999993));
#51241=CARTESIAN_POINT('Ctrl Pts',(0.413137738253102,0.614713668153683,
-0.0710999999999991));
#51242=CARTESIAN_POINT('Ctrl Pts',(0.406859115394236,0.618254100749264,
-0.0711000000000006));
#51243=CARTESIAN_POINT('Ctrl Pts',(0.400537808541689,0.621698188698112,
-0.0711000000000007));
#51244=CARTESIAN_POINT('Ctrl Pts',(0.369358146635338,0.638686052177249,
-0.0711000000000012));
#51245=CARTESIAN_POINT('Ctrl Pts',(0.337070510684383,0.65337634097395,-0.0711000000000023));
#51246=CARTESIAN_POINT('Ctrl Pts',(0.303891343528074,0.665602796457808,
-0.0711000000000025));
#51247=CARTESIAN_POINT('Ctrl Pts',(0.275872617224997,0.675927640003309,
-0.0711000000000027));
#51248=CARTESIAN_POINT('Ctrl Pts',(0.2472171506619,0.684494612208159,-0.0711000000000028));
#51249=CARTESIAN_POINT('Ctrl Pts',(0.218096358592357,0.691272993639705,
-0.071100000000003));
#51250=CARTESIAN_POINT('Ctrl Pts',(0.202620172922082,0.694875350654172,
-0.0711000000000031));
#51251=CARTESIAN_POINT('Ctrl Pts',(0.187012534642492,0.697972065861056,
-0.0711000000000009));
#51252=CARTESIAN_POINT('Ctrl Pts',(0.171299516949898,0.700555257048155,
-0.071100000000001));
#51253=CARTESIAN_POINT('Ctrl Pts',(0.163746901610617,0.701796893108501,
-0.0711000000000011));
#51254=CARTESIAN_POINT('Ctrl Pts',(0.156169947568287,0.702919853992287,
-0.0711000000000002));
#51255=CARTESIAN_POINT('Ctrl Pts',(0.148571605417996,0.703923076234743,
-0.0711000000000002));
#51256=CARTESIAN_POINT('Ctrl Pts',(0.140949579614127,0.704929425470902,
-0.0711000000000003));
#51257=CARTESIAN_POINT('Ctrl Pts',(0.133314942393103,0.705814064021666,
-0.0711000000000012));
#51258=CARTESIAN_POINT('Ctrl Pts',(0.125675256770885,0.706576348697078,
-0.0711000000000011));
#51259=CARTESIAN_POINT('Ctrl Pts',(0.0918942032621264,0.709947008261146,
-0.0711000000000007));
#51260=CARTESIAN_POINT('Ctrl Pts',(0.0579854030734698,0.710933280173858,
-0.0710999999999987));
#51261=CARTESIAN_POINT('Ctrl Pts',(0.0242035334269883,0.709501173726401,
-0.0710999999999993));
#51262=CARTESIAN_POINT('Ctrl Pts',(-0.000358657995172887,0.70845991481837,
-0.0710999999999997));
#51263=CARTESIAN_POINT('Ctrl Pts',(-0.024853941788823,0.706139122614643,
-0.0711000000000006));
#51264=CARTESIAN_POINT('Ctrl Pts',(-0.0491808006996979,0.702508747012482,
-0.0711000000000007));
#51265=CARTESIAN_POINT('Ctrl Pts',(-0.0650275557039196,0.700143884662125,
-0.0711000000000008));
#51266=CARTESIAN_POINT('Ctrl Pts',(-0.080802759147321,0.697222993781091,
-0.0711000000000019));
#51267=CARTESIAN_POINT('Ctrl Pts',(-0.0964785109981452,0.693753240057663,
-0.0711000000000019));
#51268=CARTESIAN_POINT('Ctrl Pts',(-0.104693255733889,0.691934945062622,
-0.0711000000000019));
#51269=CARTESIAN_POINT('Ctrl Pts',(-0.112880665544142,0.689965885761257,
-0.071100000000001));
#51270=CARTESIAN_POINT('Ctrl Pts',(-0.121036547279302,0.687846867496625,
-0.071100000000001));
#51271=CARTESIAN_POINT('Ctrl Pts',(-0.12712368240448,0.686265340087524,
-0.071100000000001));
#51272=CARTESIAN_POINT('Ctrl Pts',(-0.133191875532908,0.684600545569067,
-0.0711000000000012));
#51273=CARTESIAN_POINT('Ctrl Pts',(-0.139230257177048,0.682855775576718,
-0.0711000000000012));
#51274=CARTESIAN_POINT('Ctrl Pts',(-0.171263564902799,0.673599859443985,
-0.0711000000000012));
#51275=CARTESIAN_POINT('Ctrl Pts',(-0.202532061429895,0.662078717887296,
-0.071100000000002));
#51276=CARTESIAN_POINT('Ctrl Pts',(-0.23280063481128,0.648397909317886,
-0.0711000000000016));
#51277=CARTESIAN_POINT('Ctrl Pts',(-0.262509394373431,0.634970125745688,
-0.0711000000000013));
#51278=CARTESIAN_POINT('Ctrl Pts',(-0.291255846843352,0.619461112155213,
-0.0710999999999998));
#51279=CARTESIAN_POINT('Ctrl Pts',(-0.318789308023056,0.601930587013271,
-0.0710999999999998));
#51280=CARTESIAN_POINT('Ctrl Pts',(-0.334282722599328,0.592065946603873,
-0.0710999999999997));
#51281=CARTESIAN_POINT('Ctrl Pts',(-0.349391454463959,0.581560537742664,
-0.0711000000000004));
#51282=CARTESIAN_POINT('Ctrl Pts',(-0.364065050236216,0.570420484551968,
-0.0711000000000004));
#51283=CARTESIAN_POINT('Ctrl Pts',(-0.292601934307084,0.610169646934156,
-5.87494887079529));
#51284=CARTESIAN_POINT('Ctrl Pts',(-0.393926377869307,0.561580327016552,
-5.86966303393665));
#51285=CARTESIAN_POINT('Ctrl Pts',(-0.571801589437153,0.41300180871426,
-5.85909136021935));
#51286=CARTESIAN_POINT('Ctrl Pts',(-0.699630454730174,0.089520482193593,
-5.84323384964341));
#51287=CARTESIAN_POINT('Ctrl Pts',(-0.65737507433218,-0.255632286976451,
-5.82737633906746));
#51288=CARTESIAN_POINT('Ctrl Pts',(-0.455323085285772,-0.53868739721303,
-5.81151882849152));
#51289=CARTESIAN_POINT('Ctrl Pts',(-0.142583287492297,-0.690769884805212,
-5.79566131791557));
#51290=CARTESIAN_POINT('Ctrl Pts',(0.204815806457288,-0.674943835808658,
-5.77980380733964));
#51291=CARTESIAN_POINT('Ctrl Pts',(0.502426729513632,-0.495039039708356,
-5.76394629676369));
#51292=CARTESIAN_POINT('Ctrl Pts',(0.677901792498161,-0.194797654574707,
-5.74808878618775));
#51293=CARTESIAN_POINT('Ctrl Pts',(0.688585132880224,0.152798855491627,
-5.7322312756118));
#51294=CARTESIAN_POINT('Ctrl Pts',(0.531879433776216,0.463250529001845,
-5.71637376503586));
#51295=CARTESIAN_POINT('Ctrl Pts',(0.245878610535506,0.661090510301056,
-5.70051625445991));
#51296=CARTESIAN_POINT('Ctrl Pts',(-0.0998931488246837,0.698225042897434,
-5.68465874388397));
#51297=CARTESIAN_POINT('Ctrl Pts',(-0.421381756118886,0.565627364000294,
-5.66880123330803));
#51298=CARTESIAN_POINT('Ctrl Pts',(-0.640436201277647,0.295530633571676,
-5.65294372273209));
#51299=CARTESIAN_POINT('Ctrl Pts',(-0.70380628058059,-0.0464069459234262,
-5.63708621215614));
#51300=CARTESIAN_POINT('Ctrl Pts',(-0.596087294840688,-0.377063422523974,
-5.6212287015802));
#51301=CARTESIAN_POINT('Ctrl Pts',(-0.343464771761306,-0.61605911690008,
-5.60537119100425));
#51302=CARTESIAN_POINT('Ctrl Pts',(-0.00734900831199806,-0.705296305700142,
-5.58951368042832));
#51303=CARTESIAN_POINT('Ctrl Pts',(0.330553234139647,-0.623082213877371,
-5.57365616985237));
#51304=CARTESIAN_POINT('Ctrl Pts',(0.588100915954884,-0.389402361121922,
-5.55779865927643));
#51305=CARTESIAN_POINT('Ctrl Pts',(0.70268647930235,-0.0610622463428964,
-5.54194114870048));
#51306=CARTESIAN_POINT('Ctrl Pts',(0.646455189560342,0.282121558884655,
-5.52608363812454));
#51307=CARTESIAN_POINT('Ctrl Pts',(0.433076374763486,0.556724114585172,
-5.5102261275486));
#51308=CARTESIAN_POINT('Ctrl Pts',(0.114420532934634,0.695991973912722,
-5.49436861697265));
#51309=CARTESIAN_POINT('Ctrl Pts',(-0.232049925986955,0.666070355123448,
-5.47851110639671));
#51310=CARTESIAN_POINT('Ctrl Pts',(-0.522111105272023,0.47423293840623,
-5.46265359582076));
#51311=CARTESIAN_POINT('Ctrl Pts',(-0.685251703933044,0.167113698949432,
-5.44679608524482));
#51312=CARTESIAN_POINT('Ctrl Pts',(-0.681813688851661,-0.180629399086395,
-5.43093857466888));
#51313=CARTESIAN_POINT('Ctrl Pts',(-0.512632811011637,-0.484463091673161,
-5.41508106409294));
#51314=CARTESIAN_POINT('Ctrl Pts',(-0.218835441848411,-0.670528101954526,
-5.39922355351699));
#51315=CARTESIAN_POINT('Ctrl Pts',(0.128158883019949,-0.693593675592924,
-5.38336604294105));
#51316=CARTESIAN_POINT('Ctrl Pts',(0.443998919690547,-0.548052776138566,
-5.3675085323651));
#51317=CARTESIAN_POINT('Ctrl Pts',(0.651906755505725,-0.269285105873896,
-5.35165102178917));
#51318=CARTESIAN_POINT('Ctrl Pts',(0.701341838902262,0.0749433861305649,
-5.33579351121321));
#51319=CARTESIAN_POINT('Ctrl Pts',(0.580286939400919,0.400953805419331,
-5.31993600063728));
#51320=CARTESIAN_POINT('Ctrl Pts',(0.31816942979039,0.62949590949138,-5.30407849006133));
#51321=CARTESIAN_POINT('Ctrl Pts',(-0.0212922472927337,0.705013139114975,
-5.28822097948539));
#51322=CARTESIAN_POINT('Ctrl Pts',(-0.355577967837347,0.609147925308939,
-5.27236346890944));
#51323=CARTESIAN_POINT('Ctrl Pts',(-0.603425836976519,0.365204251602734,
-5.2565059583335));
#51324=CARTESIAN_POINT('Ctrl Pts',(-0.704586235156745,0.0324826622549327,
-5.24064844775756));
#51325=CARTESIAN_POINT('Ctrl Pts',(-0.634467966474636,-0.30813517429379,
-5.22479093718161));
#51326=CARTESIAN_POINT('Ctrl Pts',(-0.410116160373992,-0.573848081916823,
-5.20893342660567));
#51327=CARTESIAN_POINT('Ctrl Pts',(-0.0860687518011682,-0.700063608597757,
-5.19307591602972));
#51328=CARTESIAN_POINT('Ctrl Pts',(0.25890120724375,-0.656099878834963,
-5.17721840545379));
#51329=CARTESIAN_POINT('Ctrl Pts',(0.540934578241509,-0.452644085548684,
-5.16136089487784));
#51330=CARTESIAN_POINT('Ctrl Pts',(0.691471549227516,-0.139154528235421,
-5.1455033843019));
#51331=CARTESIAN_POINT('Ctrl Pts',(0.673917917224984,0.208162261139392,
-5.12964587372595));
#51332=CARTESIAN_POINT('Ctrl Pts',(0.492540814542161,0.504876650410443,
-5.11378836315001));
#51333=CARTESIAN_POINT('Ctrl Pts',(0.191431406740854,0.678860002233702,
-5.09793085257407));
#51334=CARTESIAN_POINT('Ctrl Pts',(-0.156213278796698,0.687818506327875,
-5.08207334199812));
#51335=CARTESIAN_POINT('Ctrl Pts',(-0.465883901255171,0.529574429774311,
-5.06621583142218));
#51336=CARTESIAN_POINT('Ctrl Pts',(-0.662302277873419,0.242595504581606,
-5.05035832084624));
#51337=CARTESIAN_POINT('Ctrl Pts',(-0.697720842752782,-0.103356236908438,
-5.03450081027029));
#51338=CARTESIAN_POINT('Ctrl Pts',(-0.563529656794226,-0.424182993568702,
-5.01864329969435));
#51339=CARTESIAN_POINT('Ctrl Pts',(-0.292349407557091,-0.641894625324549,
-5.00278578911841));
#51340=CARTESIAN_POINT('Ctrl Pts',(0.0498983906696054,-0.703567364740653,
-4.98692827854246));
#51341=CARTESIAN_POINT('Ctrl Pts',(0.380016332526679,-0.594209115659208,
-4.97107076796653));
#51342=CARTESIAN_POINT('Ctrl Pts',(0.617755673194353,-0.340403898855044,
-4.95521325739056));
#51343=CARTESIAN_POINT('Ctrl Pts',(0.705324086767725,-0.00384951228082019,
-4.93935574681464));
#51344=CARTESIAN_POINT('Ctrl Pts',(0.621434468293966,0.333640656598862,
-4.92349823623868));
#51345=CARTESIAN_POINT('Ctrl Pts',(0.386479640253609,0.590025739937645,
-4.90764072566275));
#51346=CARTESIAN_POINT('Ctrl Pts',(0.0575750382195188,0.702980797101559,
-4.8917832150868));
#51347=CARTESIAN_POINT('Ctrl Pts',(-0.285325545141958,0.645047455160447,
-4.87592570451086));
#51348=CARTESIAN_POINT('Ctrl Pts',(-0.558866018193005,0.430308795899666,
-4.86006819393491));
#51349=CARTESIAN_POINT('Ctrl Pts',(-0.696551117161325,0.110965883499543,
-4.84421068335897));
#51350=CARTESIAN_POINT('Ctrl Pts',(-0.664910815212153,-0.23535185134907,
-4.82835317278303));
#51351=CARTESIAN_POINT('Ctrl Pts',(-0.471636589224496,-0.524457637778504,
-4.81249566220709));
#51352=CARTESIAN_POINT('Ctrl Pts',(-0.163711689954952,-0.686072422337189,
-4.79663815163114));
#51353=CARTESIAN_POINT('Ctrl Pts',(0.184010069664874,-0.680909083785385,
-4.7807806410552));
#51354=CARTESIAN_POINT('Ctrl Pts',(0.487000612793599,-0.510222783946564,
-4.76492313047925));
#51355=CARTESIAN_POINT('Ctrl Pts',(0.671605624729155,-0.215505848996464,
-4.74906561990332));
#51356=CARTESIAN_POINT('Ctrl Pts',(0.692949263789228,0.131598647156757,
-4.73320810932736));
#51357=CARTESIAN_POINT('Ctrl Pts',(0.545843080552321,0.446712678947753,
-4.71735059875143));
#51358=CARTESIAN_POINT('Ctrl Pts',(0.266047283910979,0.653234819068239,
-4.70149308817548));
#51359=CARTESIAN_POINT('Ctrl Pts',(-0.0784222486577756,0.700961366292738,
-4.68563557759954));
#51360=CARTESIAN_POINT('Ctrl Pts',(-0.403828027874236,0.578290420137434,
-4.66977806702359));
#51361=CARTESIAN_POINT('Ctrl Pts',(-0.631066793878241,0.315042200004637,
-4.65392055644765));
#51362=CARTESIAN_POINT('Ctrl Pts',(-0.704898817366892,-0.0247899857660444,
-4.6380630458717));
#51363=CARTESIAN_POINT('Ctrl Pts',(-0.607376188029295,-0.358595945786518,
-4.62220553529577));
#51364=CARTESIAN_POINT('Ctrl Pts',(-0.362205792415875,-0.605230410719679,
-4.60634802471981));
#51365=CARTESIAN_POINT('Ctrl Pts',(-0.0289863800046666,-0.704738728816396,
-4.59049051414388));
#51366=CARTESIAN_POINT('Ctrl Pts',(0.311279364390673,-0.632931310194133,
-4.57463300356793));
#51367=CARTESIAN_POINT('Ctrl Pts',(0.575875855124356,-0.407263901671038,
-4.55877549299199));
#51368=CARTESIAN_POINT('Ctrl Pts',(0.700482031227543,-0.0825942494781502,
-4.54291798241604));
#51369=CARTESIAN_POINT('Ctrl Pts',(0.654807236055464,0.262153332477254,
-4.5270604718401));
#51370=CARTESIAN_POINT('Ctrl Pts',(0.449954607358944,0.543173763574772,
-4.51120296126416));
#51371=CARTESIAN_POINT('Ctrl Pts',(0.13572200293829,0.692153468558775,-4.49534545068821));
#51372=CARTESIAN_POINT('Ctrl Pts',(-0.211503417077158,0.672876802010746,
-4.47948794011228));
#51373=CARTESIAN_POINT('Ctrl Pts',(-0.507314231603265,0.49002975066042,
-4.46363042953633));
#51374=CARTESIAN_POINT('Ctrl Pts',(-0.679801454305346,0.188060811558017,
-4.44777291896038));
#51375=CARTESIAN_POINT('Ctrl Pts',(-0.687034970626699,-0.159624043475585,
-4.43191540838445));
#51376=CARTESIAN_POINT('Ctrl Pts',(-0.527256376882394,-0.468505708776717,
-4.41605789780849));
#51377=CARTESIAN_POINT('Ctrl Pts',(-0.239306432604977,-0.663497790074244,
-4.40020038723256));
#51378=CARTESIAN_POINT('Ctrl Pts',(0.106816783733375,-0.697199441216343,
-4.38434287665661));
#51379=CARTESIAN_POINT('Ctrl Pts',(0.426973786990221,-0.561418089611258,
-4.36848536608067));
#51380=CARTESIAN_POINT('Ctrl Pts',(0.64333724820522,-0.289160977988487,
-4.35262785550472));
#51381=CARTESIAN_POINT('Ctrl Pts',(0.703311128248571,0.0533886036645251,
-4.33677034492878));
#51382=CARTESIAN_POINT('Ctrl Pts',(0.592316308613785,0.382959889113288,
-4.32091283435284));
#51383=CARTESIAN_POINT('Ctrl Pts',(0.337334645867288,0.619437020864201,
-4.3050553237769));
#51384=CARTESIAN_POINT('Ctrl Pts',(0.000349921539867571,0.7053345048092,
-4.28919781320095));
#51385=CARTESIAN_POINT('Ctrl Pts',(-0.336719865611468,0.619771424173557,
-4.27334030262501));
#51386=CARTESIAN_POINT('Ctrl Pts',(-0.591936038811396,0.383547405252334,
-4.25748279204906));
#51387=CARTESIAN_POINT('Ctrl Pts',(-0.70325780911707,0.0540864126688136,
-4.24162528147312));
#51388=CARTESIAN_POINT('Ctrl Pts',(-0.643623841152751,-0.288522507301082,
-4.22576777089717));
#51389=CARTESIAN_POINT('Ctrl Pts',(-0.427530623812185,-0.560994163804123,
-4.20991026032124));
#51390=CARTESIAN_POINT('Ctrl Pts',(-0.107508502335302,-0.697093112894644,
-4.19405274974529));
#51391=CARTESIAN_POINT('Ctrl Pts',(0.238647982882395,-0.663734906710268,
-4.17819523916935));
#51392=CARTESIAN_POINT('Ctrl Pts',(0.526791259328862,-0.469028629418541,
-4.1623377285934));
#51393=CARTESIAN_POINT('Ctrl Pts',(0.68687625119572,-0.160305650751426,
-4.14648021801746));
#51394=CARTESIAN_POINT('Ctrl Pts',(0.679987716283376,0.187386210333744,
-4.13062270744152));
#51395=CARTESIAN_POINT('Ctrl Pts',(0.507800196354854,0.489526145064282,
-4.11476519686557));
#51396=CARTESIAN_POINT('Ctrl Pts',(0.212170950879785,0.672666614098168,
-4.09890768628963));
#51397=CARTESIAN_POINT('Ctrl Pts',(-0.135035171633647,0.692287793147759,
-4.08305017571368));
#51398=CARTESIAN_POINT('Ctrl Pts',(-0.449415441152957,0.543619947548669,
-4.06719266513775));
#51399=CARTESIAN_POINT('Ctrl Pts',(-0.654546801472525,0.262802912467901,
-4.0513351545618));
#51400=CARTESIAN_POINT('Ctrl Pts',(-0.700563637605738,-0.0818991806072614,
-4.03547764398586));
#51401=CARTESIAN_POINT('Ctrl Pts',(-0.576279664676672,-0.406692308999895,
-4.01962013340991));
#51402=CARTESIAN_POINT('Ctrl Pts',(-0.311907214595146,-0.632622142833319,
-4.00376262283397));
#51403=CARTESIAN_POINT('Ctrl Pts',(0.0282871139661857,-0.70476714261023,
-3.98790511225803));
#51404=CARTESIAN_POINT('Ctrl Pts',(0.361605095917608,-0.6055894985268,-3.97204760168208));
#51405=CARTESIAN_POINT('Ctrl Pts',(0.607020085064156,-0.35919841654471,
-3.95619009110614));
#51406=CARTESIAN_POINT('Ctrl Pts',(0.704873873408482,-0.0254893841755349,
-3.9403325805302));
#51407=CARTESIAN_POINT('Ctrl Pts',(0.631379072581692,0.31441589149629,-3.92447506995425));
#51408=CARTESIAN_POINT('Ctrl Pts',(0.40440161705542,0.57788945157572,-3.90861755937831));
#51409=CARTESIAN_POINT('Ctrl Pts',(0.0791177138722245,0.700883209579997,
-3.89276004880237));
#51410=CARTESIAN_POINT('Ctrl Pts',(-0.265399004090862,0.653498473408395,
-3.87690253822642));
#51411=CARTESIAN_POINT('Ctrl Pts',(-0.545399577203117,0.447254052308289,
-3.86104502765048));
#51412=CARTESIAN_POINT('Ctrl Pts',(-0.692818348643004,0.132286136473575,
-3.84518751707454));
#51413=CARTESIAN_POINT('Ctrl Pts',(-0.67181912209725,-0.214839366280961,
-3.82933000649859));
#51414=CARTESIAN_POINT('Ctrl Pts',(-0.487506623358711,-0.50973932387144,
-3.81347249592265));
#51415=CARTESIAN_POINT('Ctrl Pts',(-0.184685586744943,-0.680726171208512,
-3.79761498534671));
#51416=CARTESIAN_POINT('Ctrl Pts',(0.163030878572916,-0.686234521684292,
-3.78175747477076));
#51417=CARTESIAN_POINT('Ctrl Pts',(0.471115982751349,-0.524925344135482,
-3.76589996419482));
#51418=CARTESIAN_POINT('Ctrl Pts',(0.664676968465788,-0.236011469447257,
-3.75004245361887));
#51419=CARTESIAN_POINT('Ctrl Pts',(0.696660876212486,0.110274700971604,
-3.73418494304293));
#51420=CARTESIAN_POINT('Ctrl Pts',(0.559292701589483,0.429754069286446,
-3.71832743246699));
#51421=CARTESIAN_POINT('Ctrl Pts',(0.285965429933078,0.644764033583383,
-3.70246992189105));
#51422=CARTESIAN_POINT('Ctrl Pts',(-0.0568775023532221,0.703037577833207,
-3.6866124113151));
#51423=CARTESIAN_POINT('Ctrl Pts',(-0.385894018096841,0.590408920085563,
-3.67075490073916));
#51424=CARTESIAN_POINT('Ctrl Pts',(-0.621103119400875,0.334257088466388,
-3.65489739016321));
#51425=CARTESIAN_POINT('Ctrl Pts',(-0.70532755911646,-0.00314967781535797,
-3.63903987958727));
#51426=CARTESIAN_POINT('Ctrl Pts',(-0.618093122687726,-0.339790785345425,
-3.62318236901133));
#51427=CARTESIAN_POINT('Ctrl Pts',(-0.380605728184695,-0.593831765563718,
-3.60732485843538));
#51428=CARTESIAN_POINT('Ctrl Pts',(-0.0505964556334205,-0.703517508521898,
-3.59146734785944));
#51429=CARTESIAN_POINT('Ctrl Pts',(0.291712366691096,-0.642184382587279,
-3.5756098372835));
#51430=CARTESIAN_POINT('Ctrl Pts',(0.563108499012531,-0.424741926891352,
-3.55975232670755));
#51431=CARTESIAN_POINT('Ctrl Pts',(0.697617947778104,-0.104048474555806,
-3.54389481613161));
#51432=CARTESIAN_POINT('Ctrl Pts',(0.66254265856183,0.241938239444174,-3.52803730555567));
#51433=CARTESIAN_POINT('Ctrl Pts',(0.466409123192545,0.529111912474371,
-3.51217979497972));
#51434=CARTESIAN_POINT('Ctrl Pts',(0.156895665186708,0.687663170720335,
-3.49632228440378));
#51435=CARTESIAN_POINT('Ctrl Pts',(-0.19075773797954,0.679049609027539,
-3.48046477382783));
#51436=CARTESIAN_POINT('Ctrl Pts',(-0.492039626312628,0.505365107875141,
-3.4646072632519));
#51437=CARTESIAN_POINT('Ctrl Pts',(-0.67371104394227,0.208830829595975,
-3.44874975267595));
#51438=CARTESIAN_POINT('Ctrl Pts',(-0.691609279952494,-0.138468371851177,
-3.43289224210001));
#51439=CARTESIAN_POINT('Ctrl Pts',(-0.541383431856071,-0.452107139770282,
-3.41703473152406));
#51440=CARTESIAN_POINT('Ctrl Pts',(-0.259552071413764,-0.655842670420542,
-3.40117722094812));
#51441=CARTESIAN_POINT('Ctrl Pts',(0.0853740963848333,-0.700148662632442,
-3.38531971037218));
#51442=CARTESIAN_POINT('Ctrl Pts',(0.409546578284193,-0.574254722518878,
-3.36946219979623));
#51443=CARTESIAN_POINT('Ctrl Pts',(0.634161918067455,-0.308764550738151,
-3.35360468922029));
#51444=CARTESIAN_POINT('Ctrl Pts',(0.70461811808652,0.0317835458017981,
-3.33774717864434));
#51445=CARTESIAN_POINT('Ctrl Pts',(0.603787900785698,0.364605344152174,
-3.32188966806841));
#51446=CARTESIAN_POINT('Ctrl Pts',(0.356182198023997,0.608794815952237,
-3.30603215749246));
#51447=CARTESIAN_POINT('Ctrl Pts',(0.021991760855621,0.704991665606051,
-3.29017464691652));
#51448=CARTESIAN_POINT('Ctrl Pts',(-0.317544678396473,0.629811291849872,
-3.27431713634057));
#51449=CARTESIAN_POINT('Ctrl Pts',(-0.579888821700749,0.401529376990078,
-3.25845962576463));
#51450=CARTESIAN_POINT('Ctrl Pts',(-0.701267133779017,0.0756392305677909,
-3.24260211518869));
#51451=CARTESIAN_POINT('Ctrl Pts',(-0.652173623112518,-0.268638142183524,
-3.22674460461274));
#51452=CARTESIAN_POINT('Ctrl Pts',(-0.44454248687824,-0.547611964332075,
-3.2108870940368));
#51453=CARTESIAN_POINT('Ctrl Pts',(-0.128847013424495,-0.693466173112368,
-3.19502958346085));
#51454=CARTESIAN_POINT('Ctrl Pts',(0.218170026627314,-0.670744903522167,
-3.17917207288491));
#51455=CARTESIAN_POINT('Ctrl Pts',(0.512151867514703,-0.484971494750699,
-3.16331456230897));
#51456=CARTESIAN_POINT('Ctrl Pts',(0.681634130178766,-0.181305815392006,
-3.14745705173302));
#51457=CARTESIAN_POINT('Ctrl Pts',(0.68541717920589,0.166433700220129,-3.13159954115708));
#51458=CARTESIAN_POINT('Ctrl Pts',(0.522581388918324,0.473714658920027,
-3.11574203058114));
#51459=CARTESIAN_POINT('Ctrl Pts',(0.232710696222986,0.665839784019352,
-3.0998845200052));
#51460=CARTESIAN_POINT('Ctrl Pts',(-0.113729903497026,0.696105160999459,
-3.08402700942925));
#51461=CARTESIAN_POINT('Ctrl Pts',(-0.432523772013128,0.557153545051146,
-3.0681694988533));
#51462=CARTESIAN_POINT('Ctrl Pts',(-0.646174946334819,0.282762842058002,
-3.05231198827737));
#51463=CARTESIAN_POINT('Ctrl Pts',(-0.702746720228755,-0.0603650008469461,
-3.03645447770142));
#51464=CARTESIAN_POINT('Ctrl Pts',(-0.588486997030099,-0.388818647245757,
-3.02059696712548));
#51465=CARTESIAN_POINT('Ctrl Pts',(-0.331171302414811,-0.62275392778882,
-3.00473945654953));
#51466=CARTESIAN_POINT('Ctrl Pts',(0.00664919963267667,-0.70530324986049,
-2.98888194597359));
#51467=CARTESIAN_POINT('Ctrl Pts',(0.342853340201669,-0.61639960515244,
-2.97302443539765));
#51468=CARTESIAN_POINT('Ctrl Pts',(0.595712873526129,-0.377654681468092,
-2.9571669248217));
#51469=CARTESIAN_POINT('Ctrl Pts',(0.703759888922834,-0.0471052530281482,
-2.94130941424576));
#51470=CARTESIAN_POINT('Ctrl Pts',(0.640729114900228,0.29489504478491,-2.92545190366982));
#51471=CARTESIAN_POINT('Ctrl Pts',(0.421942773788548,0.565208971768099,
-2.90959439309387));
#51472=CARTESIAN_POINT('Ctrl Pts',(0.100585885339081,0.698125608891462,
-2.89373688251793));
#51473=CARTESIAN_POINT('Ctrl Pts',(-0.245222540035754,0.661334100117283,
-2.87787937194199));
#51474=CARTESIAN_POINT('Ctrl Pts',(-0.531419540085806,0.463778135032813,
-2.86202186136604));
#51475=CARTESIAN_POINT('Ctrl Pts',(-0.688433161538855,0.153481817206925,
-2.8461643507901));
#51476=CARTESIAN_POINT('Ctrl Pts',(-0.678094785111951,-0.194124569602876,
-2.83030684021415));
#51477=CARTESIAN_POINT('Ctrl Pts',(-0.502917578453797,-0.494540994662418,
-2.81444932963821));
#51478=CARTESIAN_POINT('Ctrl Pts',(-0.205485567371259,-0.674738888549961,
-2.79859181906227));
#51479=CARTESIAN_POINT('Ctrl Pts',(0.141898163291737,-0.690913740906892,
-2.78273430848633));
#51480=CARTESIAN_POINT('Ctrl Pts',(0.454787708536229,-0.539133588532463,
-2.76687679791038));
#51481=CARTESIAN_POINT('Ctrl Pts',(0.657122394010951,-0.256294840776867,
-2.75101928733444));
#51482=CARTESIAN_POINT('Ctrl Pts',(0.69971645158859,0.0888469104459926,
-2.7351617767585));
#51483=CARTESIAN_POINT('Ctrl Pts',(0.572215643513511,0.412390765461524,
-2.71930426618255));
#51484=CARTESIAN_POINT('Ctrl Pts',(0.305614285798879,0.635686081674883,
-2.70344675560661));
#51485=CARTESIAN_POINT('Ctrl Pts',(-0.0352791951986797,0.704451747464407,
-2.68758924503067));
#51486=CARTESIAN_POINT('Ctrl Pts',(-0.367596616630921,0.601971439157228,
-2.67173173445472));
#51487=CARTESIAN_POINT('Ctrl Pts',(-0.610554559694072,0.353157211106192,
-2.65587422387878));
#51488=CARTESIAN_POINT('Ctrl Pts',(-0.705092102509325,0.0184935961484815,
-2.64001671330283));
#51489=CARTESIAN_POINT('Ctrl Pts',(-0.628228006593883,-0.320665648067582,
-2.62415920272689));
#51490=CARTESIAN_POINT('Ctrl Pts',(-0.398647252183052,-0.581873916279484,
-2.60830169215095));
#51491=CARTESIAN_POINT('Ctrl Pts',(-0.072158885197231,-0.701633794373258,
-2.59244418157501));
#51492=CARTESIAN_POINT('Ctrl Pts',(0.271870667014987,-0.650832717782648,
-2.57658667099906));
#51493=CARTESIAN_POINT('Ctrl Pts',(0.549810870497681,-0.441819977821406,
-2.56072916042312));
#51494=CARTESIAN_POINT('Ctrl Pts',(0.694096926018893,-0.125404718454481,
-2.54487164984717));
#51495=CARTESIAN_POINT('Ctrl Pts',(0.669654172730331,0.221495316122894,
-2.52901413927123));
#51496=CARTESIAN_POINT('Ctrl Pts',(0.48242442724551,0.514551803141691,-2.51315662869529));
#51497=CARTESIAN_POINT('Ctrl Pts',(0.17792158070152,0.682525308864219,-2.49729911811934));
#51498=CARTESIAN_POINT('Ctrl Pts',(-0.169832424647492,0.684582963312612,
-2.4814416075434));
#51499=CARTESIAN_POINT('Ctrl Pts',(-0.476301673309269,0.520224568933759,
-2.46558409696745));
#51500=CARTESIAN_POINT('Ctrl Pts',(-0.666986208109069,0.229404194189668,
-2.44972658639152));
#51501=CARTESIAN_POINT('Ctrl Pts',(-0.695532309257702,-0.11718230625044,
-2.43386907581557));
#51502=CARTESIAN_POINT('Ctrl Pts',(-0.555000672657401,-0.435282826986497,
-2.41801156523963));
#51503=CARTESIAN_POINT('Ctrl Pts',(-0.27955329320369,-0.647569951726063,
-2.40215405466368));
#51504=CARTESIAN_POINT('Ctrl Pts',(0.0638510132913964,-0.702438562595467,
-2.38629654408774));
#51505=CARTESIAN_POINT('Ctrl Pts',(0.391733704562298,-0.586550586760786,
-2.3704390335118));
#51506=CARTESIAN_POINT('Ctrl Pts',(0.624389405388874,-0.328077363677613,
-2.35458152293585));
#51507=CARTESIAN_POINT('Ctrl Pts',(0.70526157763973,0.0101485577617963,
-2.33872401235991));
#51508=CARTESIAN_POINT('Ctrl Pts',(0.614690913258262,0.345907454787038,
-2.32286650178397));
#51509=CARTESIAN_POINT('Ctrl Pts',(0.374694337750614,0.59757931639001,-2.30700899120802));
#51510=CARTESIAN_POINT('Ctrl Pts',(0.0436128907985044,0.703984944353017,
-2.29115148063208));
#51511=CARTESIAN_POINT('Ctrl Pts',(-0.298070463232192,0.639258073916999,
-2.27529397005614));
#51512=CARTESIAN_POINT('Ctrl Pts',(-0.567295530361938,0.419133233412588,
-2.25943645948019));
#51513=CARTESIAN_POINT('Ctrl Pts',(-0.698616083737257,0.0971208199262295,
-2.24357894890425));
#51514=CARTESIAN_POINT('Ctrl Pts',(-0.660109261128591,-0.248500803805119,
-2.22772143832831));
#51515=CARTESIAN_POINT('Ctrl Pts',(-0.461135729708285,-0.533714085354632,
-2.21186392775236));
#51516=CARTESIAN_POINT('Ctrl Pts',(-0.150064190853226,-0.689186204695865,
-2.19600641717642));
#51517=CARTESIAN_POINT('Ctrl Pts',(0.197486622320041,-0.677123268042198,
-2.18014890660047));
#51518=CARTESIAN_POINT('Ctrl Pts',(0.497030188535669,-0.500457668343409,
-2.16429139602453));
#51519=CARTESIAN_POINT('Ctrl Pts',(0.675750122618055,-0.20213524655836,
-2.14843388544859));
#51520=CARTESIAN_POINT('Ctrl Pts',(0.690201193133537,0.145324461521679,
-2.13257637487265));
#51521=CARTESIAN_POINT('Ctrl Pts',(0.536870472963871,0.457457081461282,
-2.1167188642967));
#51522=CARTESIAN_POINT('Ctrl Pts',(0.253031300742842,0.65838594073986,-2.10086135372076));
#51523=CARTESIAN_POINT('Ctrl Pts',(-0.0923175372979227,0.699267015114235,
-2.08500384314482));
#51524=CARTESIAN_POINT('Ctrl Pts',(-0.415224800514443,0.57016247785808,
-2.06914633256887));
#51525=CARTESIAN_POINT('Ctrl Pts',(-0.637194596134153,0.302456497329714,
-2.05328882199293));
#51526=CARTESIAN_POINT('Ctrl Pts',(-0.70426803483956,-0.0387739761018672,
-2.03743131141698));
#51527=CARTESIAN_POINT('Ctrl Pts',(-0.600140158358559,-0.370578839715501,
-2.02157380084104));
#51528=CARTESIAN_POINT('Ctrl Pts',(-0.350123530259618,-0.612299272968753,
-2.0057162902651));
#51529=CARTESIAN_POINT('Ctrl Pts',(-0.0149949761710098,-0.705175181645777,
-1.98985877968915));
#51530=CARTESIAN_POINT('Ctrl Pts',(0.323778723678411,-0.626629255790618,
-1.97400126911321));
#51531=CARTESIAN_POINT('Ctrl Pts',(0.583844686443398,-0.395755313585723,
-1.95814375853727));
#51532=CARTESIAN_POINT('Ctrl Pts',(0.701983182336375,-0.0686767634387369,
-1.94228624796132));
#51533=CARTESIAN_POINT('Ctrl Pts',(0.649475790428822,0.275096499007858,
-1.92642873738538));
#51534=CARTESIAN_POINT('Ctrl Pts',(0.439086592159748,0.551996241567879,
-1.91057122680944));
#51535=CARTESIAN_POINT('Ctrl Pts',(0.121959336304979,0.694710591834882,
-1.89471371623349));
#51536=CARTESIAN_POINT('Ctrl Pts',(-0.224815152906662,0.668546956573044,
-1.87885620565755));
#51537=CARTESIAN_POINT('Ctrl Pts',(-0.516939071671466,0.479865483546136,
-1.86299869508161));
#51538=CARTESIAN_POINT('Ctrl Pts',(-0.68339968532608,0.174532965985627,
-1.84714118450566));
#51539=CARTESIAN_POINT('Ctrl Pts',(-0.683731894540956,-0.173226968186133,
-1.83128367392972));
#51540=CARTESIAN_POINT('Ctrl Pts',(-0.51785494220135,-0.478876962232637,
-1.81542616335378));
#51541=CARTESIAN_POINT('Ctrl Pts',(-0.226092044745908,-0.668116212512566,
-1.79956865277784));
#51542=CARTESIAN_POINT('Ctrl Pts',(0.120631824241489,-0.694942335089534,
-1.78371114220189));
#51543=CARTESIAN_POINT('Ctrl Pts',(0.438031166284854,-0.552834137407103,
-1.76785363162595));
#51544=CARTESIAN_POINT('Ctrl Pts',(0.648949015415239,-0.276336862381976,
-1.75199612105));
#51545=CARTESIAN_POINT('Ctrl Pts',(0.702113112519488,0.0673354538688382,
-1.73613861047406));
#51546=CARTESIAN_POINT('Ctrl Pts',(0.584599736947659,0.394639118284352,
-1.72028109989812));
#51547=CARTESIAN_POINT('Ctrl Pts',(0.324975348420559,0.626009511939285,
-1.70442358932217));
#51548=CARTESIAN_POINT('Ctrl Pts',(-0.0136476660564434,0.705202543480052,
-1.68856607874623));
#51549=CARTESIAN_POINT('Ctrl Pts',(-0.348953053916159,0.612967089069317,
-1.67270856817029));
#51550=CARTESIAN_POINT('Ctrl Pts',(-0.599431048207782,0.371724769909193,
-1.65685105759434));
#51551=CARTESIAN_POINT('Ctrl Pts',(-0.704192669272103,0.0401194549184884,
-1.6409935470184));
#51552=CARTESIAN_POINT('Ctrl Pts',(-0.637771295851261,-0.301238543861383,
-1.62513603644245));
#51553=CARTESIAN_POINT('Ctrl Pts',(-0.416313374927947,-0.569368123427741,
-1.60927852586652));
#51554=CARTESIAN_POINT('Ctrl Pts',(-0.0936533636192634,-0.699089360241109,
-1.59342101529057));
#51555=CARTESIAN_POINT('Ctrl Pts',(0.251772950048864,-0.658868171748504,
-1.57756350471463));
#51556=CARTESIAN_POINT('Ctrl Pts',(0.535995491794349,-0.458481972268986,
-1.56170599413868));
#51557=CARTESIAN_POINT('Ctrl Pts',(0.689922281653143,-0.146642870259839,
-1.54584848356274));
#51558=CARTESIAN_POINT('Ctrl Pts',(0.676135081734832,0.200843813364896,
-1.5299909729868));
#51559=CARTESIAN_POINT('Ctrl Pts',(0.49798543810141,0.49950714665405,-1.51413346241085));
#51560=CARTESIAN_POINT('Ctrl Pts',(0.198779949634609,0.676744721252252,
-1.49827595183491));
#51561=CARTESIAN_POINT('Ctrl Pts',(-0.148747182193283,0.689471654173747,
-1.48241844125896));
#51562=CARTESIAN_POINT('Ctrl Pts',(-0.460115192831522,0.534594140863082,
-1.46656093068302));
#51563=CARTESIAN_POINT('Ctrl Pts',(-0.659633279501605,0.249761531652658,
-1.45070342010708));
#51564=CARTESIAN_POINT('Ctrl Pts',(-0.698800364273488,-0.0957858915016492,
-1.43484590953114));
#51565=CARTESIAN_POINT('Ctrl Pts',(-0.568095276096871,-0.418048613675424,
-1.41898839895519));
#51566=CARTESIAN_POINT('Ctrl Pts',(-0.299291263068257,-0.638687424309053,
-1.40313088837925));
#51567=CARTESIAN_POINT('Ctrl Pts',(0.0422678024777705,-0.704066984734566,
-1.3872733778033));
#51568=CARTESIAN_POINT('Ctrl Pts',(0.373551939990352,-0.598294103471671,
-1.37141586722736));
#51569=CARTESIAN_POINT('Ctrl Pts',(0.614028912825419,-0.347081230166595,
-1.35555835665142));
#51570=CARTESIAN_POINT('Ctrl Pts',(0.705240900970187,-0.0114959870512474,
-1.33970084607548));
#51571=CARTESIAN_POINT('Ctrl Pts',(0.625015078797678,0.326883828592142,
-1.32384333549953));
#51572=CARTESIAN_POINT('Ctrl Pts',(0.392853632391026,0.585801083676619,
-1.30798582492359));
#51573=CARTESIAN_POINT('Ctrl Pts',(0.0651929510142312,0.702315289067225,
-1.29212831434764));
#51574=CARTESIAN_POINT('Ctrl Pts',(-0.27831555874946,0.648102874455513,
-1.2762708037717));
#51575=CARTESIAN_POINT('Ctrl Pts',(-0.554168023743774,0.43634239718304,
-1.26041329319576));
#51576=CARTESIAN_POINT('Ctrl Pts',(-0.69530715545327,0.118510951793518,
-1.24455578261981));
#51577=CARTESIAN_POINT('Ctrl Pts',(-0.667423282307466,-0.228129455251735,
-1.22869827204387));
#51578=CARTESIAN_POINT('Ctrl Pts',(-0.477294726647991,-0.519313614334867,
-1.21284076146793));
#51579=CARTESIAN_POINT('Ctrl Pts',(-0.171140054664367,-0.684257238039178,
-1.19698325089199));
#51580=CARTESIAN_POINT('Ctrl Pts',(0.176617247270067,-0.682863993842307,
-1.18112574031604));
#51581=CARTESIAN_POINT('Ctrl Pts',(0.481440462292368,-0.515472567055936,
-1.1652682297401));
#51582=CARTESIAN_POINT('Ctrl Pts',(0.669229769411713,-0.222774329429288,
-1.14941071916415));
#51583=CARTESIAN_POINT('Ctrl Pts',(0.694335253018772,0.124078372550911,
-1.13355320858821));
#51584=CARTESIAN_POINT('Ctrl Pts',(0.550653992635405,0.440768722250355,
-1.11769569801226));
#51585=CARTESIAN_POINT('Ctrl Pts',(0.273113628774048,0.650312103452947,
-1.10183818743633));
#51586=CARTESIAN_POINT('Ctrl Pts',(-0.0708182368002938,0.701770378012652,
-1.08598067686038));
#51587=CARTESIAN_POINT('Ctrl Pts',(-0.397534816887265,0.582634495616192,
-1.07012316628444));
#51588=CARTESIAN_POINT('Ctrl Pts',(-0.627614207556722,0.321865333008187,
-1.05426565570849));
#51589=CARTESIAN_POINT('Ctrl Pts',(-0.705126148834749,-0.0171464383765556,
-1.03840814513255));
#51590=CARTESIAN_POINT('Ctrl Pts',(-0.61122817502222,-0.35199006261332,
-1.0225506345566));
#51591=CARTESIAN_POINT('Ctrl Pts',(-0.368746051047842,-0.601268023394017,
-1.00669312398066));
#51592=CARTESIAN_POINT('Ctrl Pts',(-0.0366250313885693,-0.704383058566367,
-0.990835613404718));
#51593=CARTESIAN_POINT('Ctrl Pts',(0.304399208681507,-0.636268817304129,
-0.974978102828775));
#51594=CARTESIAN_POINT('Ctrl Pts',(0.571426699942949,-0.413483267753163,
-0.959120592252834));
#51595=CARTESIAN_POINT('Ctrl Pts',(0.699545426752022,-0.0901836017791227,
-0.943263081676888));
#51596=CARTESIAN_POINT('Ctrl Pts',(0.657610862529838,0.25503889821415,-0.927405571100947));
#51597=CARTESIAN_POINT('Ctrl Pts',(0.455816928044417,0.538263703241892,
-0.911548060525));
#51598=CARTESIAN_POINT('Ctrl Pts',(0.14321793965191,0.690641374290149,-0.89569054994906));
#51599=CARTESIAN_POINT('Ctrl Pts',(-0.204196060091041,0.675130250516757,
-0.879833039373114));
#51600=CARTESIAN_POINT('Ctrl Pts',(-0.501971808040508,0.495500948588465,
-0.863975528797173));
#51601=CARTESIAN_POINT('Ctrl Pts',(-0.677722659967801,0.195419759199761,
-0.848118018221228));
#51602=CARTESIAN_POINT('Ctrl Pts',(-0.688725141987106,-0.152166241046976,
-0.832260507645285));
#51603=CARTESIAN_POINT('Ctrl Pts',(-0.532304648268198,-0.462761977210308,
-0.816402997069341));
#51604=CARTESIAN_POINT('Ctrl Pts',(-0.246485614000569,-0.660864379589555,
-0.800545486493398));
#51605=CARTESIAN_POINT('Ctrl Pts',(0.0992518876742048,-0.698316510554226,
-0.784687975917454));
#51606=CARTESIAN_POINT('Ctrl Pts',(0.420862135428632,-0.566014089119677,
-0.76883046534151));
#51607=CARTESIAN_POINT('Ctrl Pts',(0.64016452944956,-0.296118660935354,
-0.752972954765568));
#51608=CARTESIAN_POINT('Ctrl Pts',(0.703848602098822,0.0457605883163558,
-0.737115444189624));
#51609=CARTESIAN_POINT('Ctrl Pts',(0.596433319942227,0.37651584426451,-0.721257933613681));
#51610=CARTESIAN_POINT('Ctrl Pts',(0.34403038572165,0.615743436684253,-0.705400423037737));
#51611=CARTESIAN_POINT('Ctrl Pts',(0.0079967149263957,0.705289258864694,
-0.689542912461795));
#51612=CARTESIAN_POINT('Ctrl Pts',(-0.329980886368106,0.623385515352452,
-0.67368540188585));
#51613=CARTESIAN_POINT('Ctrl Pts',(-0.58774305981707,0.389942280031795,
-0.657827891309908));
#51614=CARTESIAN_POINT('Ctrl Pts',(-0.702630106390092,0.0617075336872955,
-0.641970380733964));
#51615=CARTESIAN_POINT('Ctrl Pts',(-0.646714003660805,-0.281527766993847,
-0.62611287015802));
#51616=CARTESIAN_POINT('Ctrl Pts',(-0.433587460447112,-0.556326163561039,
-0.610255359582076));
#51617=CARTESIAN_POINT('Ctrl Pts',(-0.11505964981147,-0.695886602188015,
-0.594397849006135));
#51618=CARTESIAN_POINT('Ctrl Pts',(0.231438141567586,-0.66628317759591,
-0.578540338430189));
#51619=CARTESIAN_POINT('Ctrl Pts',(0.521675372676006,-0.474712219837212,
-0.562682827854247));
#51620=CARTESIAN_POINT('Ctrl Pts',(0.685097945892652,-0.167742930263535,
-0.546825317278303));
#51621=CARTESIAN_POINT('Ctrl Pts',(0.681979282582143,0.180003178438481,
-0.53096780670236));
#51622=CARTESIAN_POINT('Ctrl Pts',(0.513077502146677,0.483992110380683,
-0.515110296126415));
#51623=CARTESIAN_POINT('Ctrl Pts',(0.219451129913428,0.670326851393724,
-0.499252785550473));
#51624=CARTESIAN_POINT('Ctrl Pts',(-0.127521866330539,0.693711077989502,
-0.483395274974529));
#51625=CARTESIAN_POINT('Ctrl Pts',(-0.443495427494386,0.54846029201429,
-0.467537764398586));
#51626=CARTESIAN_POINT('Ctrl Pts',(-0.651659182275599,0.269883671725193,
-0.451680253822642));
#51627=CARTESIAN_POINT('Ctrl Pts',(-0.701410367526853,-0.0742992763408459,
-0.435822743246699));
#51628=CARTESIAN_POINT('Ctrl Pts',(-0.580654911117769,-0.400420729098558,
-0.419965232670754));
#51629=CARTESIAN_POINT('Ctrl Pts',(-0.318747394057519,-0.629203452711689,
-0.404107722094813));
#51630=CARTESIAN_POINT('Ctrl Pts',(0.0206447886986398,-0.705032395634334,
-0.388250211518869));
#51631=CARTESIAN_POINT('Ctrl Pts',(0.355018405902544,-0.609474213827725,
-0.372392700942925));
#51632=CARTESIAN_POINT('Ctrl Pts',(0.603090197140036,-0.365758254686112,
-0.356535190366982));
#51633=CARTESIAN_POINT('Ctrl Pts',(0.704556106741155,-0.0331297058619517,
-0.340677679791039));
#51634=CARTESIAN_POINT('Ctrl Pts',(0.634750676840949,0.307552379158318,
-0.324820169215095));
#51635=CARTESIAN_POINT('Ctrl Pts',(0.410642978477166,0.573471210647949,
-0.308962658639151));
#51636=CARTESIAN_POINT('Ctrl Pts',(0.0867116258434061,0.699984269273112,
-0.293105148063209));
#51637=CARTESIAN_POINT('Ctrl Pts',(-0.258298579659923,0.656337369834618,
-0.277247637487264));
#51638=CARTESIAN_POINT('Ctrl Pts',(-0.540518640889337,0.453140652074363,
-0.261390126911321));
#51639=CARTESIAN_POINT('Ctrl Pts',(-0.69134350977243,0.139789503985527,
-0.245532616335378));
#51640=CARTESIAN_POINT('Ctrl Pts',(-0.674108711481695,-0.207543320295039,
-0.229675105759435));
#51641=CARTESIAN_POINT('Ctrl Pts',(-0.493004432164587,-0.504424033259022,
-0.21381759518349));
#51642=CARTESIAN_POINT('Ctrl Pts',(-0.192054423564975,-0.67868406853937,
-0.197960084607548));
#51643=CARTESIAN_POINT('Ctrl Pts',(0.155580900692857,-0.687961374427907,
-0.182102574031604));
#51644=CARTESIAN_POINT('Ctrl Pts',(0.465398645427725,-0.530002638582951,
-0.16624506345566));
#51645=CARTESIAN_POINT('Ctrl Pts',(0.662076718045427,-0.243202481582967,
-0.150387552879718));
#51646=CARTESIAN_POINT('Ctrl Pts',(0.697820336995596,0.102713198692547,
-0.134530042303775));
#51647=CARTESIAN_POINT('Ctrl Pts',(0.563909430812559,0.423669692494884,
-0.11867253172783));
#51648=CARTESIAN_POINT('Ctrl Pts',(0.292957635797326,0.641617108208754,
-0.102815021151888));
#51649=CARTESIAN_POINT('Ctrl Pts',(-0.0492916150247689,0.703631926771629,
-0.0869575105759442));
#51650=CARTESIAN_POINT('Ctrl Pts',(-0.269341331211303,0.630876931084481,
-0.0763858368586482));
#51651=CARTESIAN_POINT('Ctrl Pts',(-0.364065050236216,0.570420484551968,
-0.0711000000000004));
#51652=CARTESIAN_POINT('Ctrl Pts',(-0.309090610374637,0.644553868208607,
-5.8529325805302));
#51653=CARTESIAN_POINT('Ctrl Pts',(-0.416124879237838,0.59322644760701,
-5.84764674367155));
#51654=CARTESIAN_POINT('Ctrl Pts',(-0.604023697624738,0.436275246927602,
-5.83707506995425));
#51655=CARTESIAN_POINT('Ctrl Pts',(-0.739055962843632,0.0945651317985082,
-5.82121755937831));
#51656=CARTESIAN_POINT('Ctrl Pts',(-0.694419411312428,-0.270037653032367,
-5.80536004880237));
#51657=CARTESIAN_POINT('Ctrl Pts',(-0.480981408007158,-0.569043457624426,
-5.78950253822642));
#51658=CARTESIAN_POINT('Ctrl Pts',(-0.150618127199263,-0.729696082934229,
-5.77364502765047));
#51659=CARTESIAN_POINT('Ctrl Pts',(0.21635756708914,-0.712978205946341,
-5.75778751707454));
#51660=CARTESIAN_POINT('Ctrl Pts',(0.5307394322654,-0.522935432074558,-5.74193000649859));
#51661=CARTESIAN_POINT('Ctrl Pts',(0.716102849126797,-0.205774873274938,
-5.72607249592265));
#51662=CARTESIAN_POINT('Ctrl Pts',(0.727388216078832,0.161409361904243,
-5.71021498534671));
#51663=CARTESIAN_POINT('Ctrl Pts',(0.561851852486622,0.489355578269279,
-5.69435747477076));
#51664=CARTESIAN_POINT('Ctrl Pts',(0.259734338354457,0.698344219171774,
-5.67849996419482));
#51665=CARTESIAN_POINT('Ctrl Pts',(-0.10552231794224,0.737571353378428,
-5.66264245361887));
#51666=CARTESIAN_POINT('Ctrl Pts',(-0.445127420322624,0.597501542829726,
-5.64678494304293));
#51667=CARTESIAN_POINT('Ctrl Pts',(-0.676526000512249,0.312184347418576,
-5.63092743246699));
#51668=CARTESIAN_POINT('Ctrl Pts',(-0.743467104430853,-0.0490220656779446,
-5.61506992189104));
#51669=CARTESIAN_POINT('Ctrl Pts',(-0.629677948764027,-0.398311664254308,
-5.59921241131511));
#51670=CARTESIAN_POINT('Ctrl Pts',(-0.362819665554462,-0.650775221019765,
-5.58335490073915));
#51671=CARTESIAN_POINT('Ctrl Pts',(-0.00776313892176305,-0.745041095302672,
-5.56749739016322));
#51672=CARTESIAN_POINT('Ctrl Pts',(0.349180538206236,-0.658194082882626,
-5.55163987958727));
#51673=CARTESIAN_POINT('Ctrl Pts',(0.621241522223168,-0.411345925533695,
-5.53578236901133));
#51674=CARTESIAN_POINT('Ctrl Pts',(0.742284200218653,-0.0645032201774955,
-5.51992485843538));
#51675=CARTESIAN_POINT('Ctrl Pts',(0.682884170243905,0.298019645844122,
-5.50406734785944));
#51676=CARTESIAN_POINT('Ctrl Pts',(0.457481052992605,0.58809657835964,-5.4882098372835));
#51677=CARTESIAN_POINT('Ctrl Pts',(0.120868347804697,0.735212446705008,
-5.47235232670755));
#51678=CARTESIAN_POINT('Ctrl Pts',(-0.245126381103904,0.703604687730767,
-5.45649481613161));
#51679=CARTESIAN_POINT('Ctrl Pts',(-0.551533060073818,0.500956867352424,
-5.44063730555566));
#51680=CARTESIAN_POINT('Ctrl Pts',(-0.723866942064143,0.176530874044159,
-5.42477979497972));
#51681=CARTESIAN_POINT('Ctrl Pts',(-0.720235188287465,-0.190808209615675,
-5.40892228440378));
#51682=CARTESIAN_POINT('Ctrl Pts',(-0.541520645886632,-0.511763509232599,
-5.39306477382784));
#51683=CARTESIAN_POINT('Ctrl Pts',(-0.231167235625787,-0.708313637082648,
-5.37720726325189));
#51684=CARTESIAN_POINT('Ctrl Pts',(0.135380880073045,-0.732678999708892,
-5.36134975267595));
#51685=CARTESIAN_POINT('Ctrl Pts',(0.469019104121168,-0.578936593482661,
-5.3454922421));
#51686=CARTESIAN_POINT('Ctrl Pts',(0.688642942309262,-0.284459834267554,
-5.32963473152407));
#51687=CARTESIAN_POINT('Ctrl Pts',(0.74086378677203,0.0791665886197745,
-5.31377722094811));
#51688=CARTESIAN_POINT('Ctrl Pts',(0.612987213213766,0.423548315709454,
-5.29791971037218));
#51689=CARTESIAN_POINT('Ctrl Pts',(0.336098882905021,0.664969202455183,
-5.28206219979623));
#51690=CARTESIAN_POINT('Ctrl Pts',(-0.0224921059648668,0.744741971741325,
-5.26620468922029));
#51691=CARTESIAN_POINT('Ctrl Pts',(-0.375615463291068,0.643474570624608,
-5.25034717864435));
#51692=CARTESIAN_POINT('Ctrl Pts',(-0.637430031720678,0.3857842064736,-5.23448966806841));
#51693=CARTESIAN_POINT('Ctrl Pts',(-0.744291010932289,0.0343131221150161,
-5.21863215749246));
#51694=CARTESIAN_POINT('Ctrl Pts',(-0.670221444315478,-0.325499178007507,
-5.20277464691652));
#51695=CARTESIAN_POINT('Ctrl Pts',(-0.433226986809527,-0.606185513851847,
-5.18691713634057));
#51696=CARTESIAN_POINT('Ctrl Pts',(-0.090918889826903,-0.739513525756312,
-5.17105962576463));
#51697=CARTESIAN_POINT('Ctrl Pts',(0.273490783180252,-0.693072356121164,
-5.15520211518868));
#51698=CARTESIAN_POINT('Ctrl Pts',(0.57141727158215,-0.478151441534479,
-5.13934460461274));
#51699=CARTESIAN_POINT('Ctrl Pts',(0.730437287482592,-0.146996150830428,
-5.1234870940368));
#51700=CARTESIAN_POINT('Ctrl Pts',(0.711894474897284,0.219892600863718,
-5.10762958346085));
#51701=CARTESIAN_POINT('Ctrl Pts',(0.52029642716401,0.533327410869022,-5.09177207288491));
#51702=CARTESIAN_POINT('Ctrl Pts',(0.202218930966826,0.71711505580522,-5.07591456230897));
#51703=CARTESIAN_POINT('Ctrl Pts',(-0.165016194463095,0.726578388660719,
-5.06005705173302));
#51704=CARTESIAN_POINT('Ctrl Pts',(-0.492137346062618,0.559416957120834,
-5.04419954115708));
#51705=CARTESIAN_POINT('Ctrl Pts',(-0.699624272153859,0.256266223129524,
-5.02834203058114));
#51706=CARTESIAN_POINT('Ctrl Pts',(-0.737038740595704,-0.109180557632705,
-5.01248452000518));
#51707=CARTESIAN_POINT('Ctrl Pts',(-0.595285625828881,-0.448086512835865,
-4.99662700942926));
#51708=CARTESIAN_POINT('Ctrl Pts',(-0.308823853261501,-0.67806660953081,
-4.98076949885331));
#51709=CARTESIAN_POINT('Ctrl Pts',(0.0527102599827489,-0.743214725228477,
-4.96491198827736));
#51710=CARTESIAN_POINT('Ctrl Pts',(0.401430976357553,-0.627693930609904,
-4.94905447770142));
#51711=CARTESIAN_POINT('Ctrl Pts',(0.652567381491205,-0.359586306632499,
-4.93319696712547));
#51712=CARTESIAN_POINT('Ctrl Pts',(0.745070441886303,-0.00406643962672281,
-4.91733945654954));
#51713=CARTESIAN_POINT('Ctrl Pts',(0.656453483698541,0.352441942799008,
-4.90148194597359));
#51714=CARTESIAN_POINT('Ctrl Pts',(0.408258503780039,0.623274813701928,
-4.88562443539765));
#51715=CARTESIAN_POINT('Ctrl Pts',(0.0608195012372539,0.742595103386185,
-4.8697669248217));
#51716=CARTESIAN_POINT('Ctrl Pts',(-0.301404182826923,0.681397107330463,
-4.85390941424576));
#51717=CARTESIAN_POINT('Ctrl Pts',(-0.590359182313632,0.454557515790763,
-4.83805190366981));
#51718=CARTESIAN_POINT('Ctrl Pts',(-0.735803098740191,0.117219022296814,
-4.82219439309388));
#51719=CARTESIAN_POINT('Ctrl Pts',(-0.702379805537885,-0.248614376246535,
-4.80633688251792));
#51720=CARTESIAN_POINT('Ctrl Pts',(-0.498214208951246,-0.554011824154478,
-4.79047937194199));
#51721=CARTESIAN_POINT('Ctrl Pts',(-0.172937155365935,-0.724733909512883,
-4.77462186136604));
#51722=CARTESIAN_POINT('Ctrl Pts',(0.194379387417532,-0.719279607003476,
-4.7587643507901));
#51723=CARTESIAN_POINT('Ctrl Pts',(0.514444024499226,-0.538974809208119,
-4.74290684021415));
#51724=CARTESIAN_POINT('Ctrl Pts',(0.709451880317066,-0.227650013877596,
-4.72704932963821));
#51725=CARTESIAN_POINT('Ctrl Pts',(0.731998274073198,0.139014481467747,
-4.71119181906227));
#51726=CARTESIAN_POINT('Ctrl Pts',(0.576602377343207,0.471885788879101,
-4.69533430848633));
#51727=CARTESIAN_POINT('Ctrl Pts',(0.281039554872709,0.690045844781952,
-4.67947679791038));
#51728=CARTESIAN_POINT('Ctrl Pts',(-0.0828414916736168,0.7404618738066,
-4.66361928733444));
#51729=CARTESIAN_POINT('Ctrl Pts',(-0.426584506071773,0.610878186288715,
-4.6477617767585));
#51730=CARTESIAN_POINT('Ctrl Pts',(-0.666628609167968,0.332795427767074,
-4.63190426618255));
#51731=CARTESIAN_POINT('Ctrl Pts',(-0.744621207745086,-0.0261869486603079,
-4.61604675560661));
#51732=CARTESIAN_POINT('Ctrl Pts',(-0.641602992576138,-0.378803510043443,
-4.60018924503066));
#51733=CARTESIAN_POINT('Ctrl Pts',(-0.382616778402954,-0.639336296629898,
-4.58433173445473));
#51734=CARTESIAN_POINT('Ctrl Pts',(-0.0306198177035606,-0.744452097899986,
-4.56847422387878));
#51735=CARTESIAN_POINT('Ctrl Pts',(0.328820549202407,-0.668598194528011,
-4.55261671330283));
#51736=CARTESIAN_POINT('Ctrl Pts',(0.608327555940194,-0.430213997898396,
-4.53675920272689));
#51737=CARTESIAN_POINT('Ctrl Pts',(0.7399555272979,-0.087248592683062,-4.52090169215095));
#51738=CARTESIAN_POINT('Ctrl Pts',(0.691706870460046,0.276926171862212,
-4.50504418157501));
#51739=CARTESIAN_POINT('Ctrl Pts',(0.475310406128392,0.573782639272009,
-4.48918667099905));
#51740=CARTESIAN_POINT('Ctrl Pts',(0.1433701961978,0.731157634266437,-4.47332916042313));
#51741=CARTESIAN_POINT('Ctrl Pts',(-0.223422037299627,0.7107946908586,-4.45747164984717));
#51742=CARTESIAN_POINT('Ctrl Pts',(-0.535902354402842,0.517643860051851,
-4.44161413927123));
#51743=CARTESIAN_POINT('Ctrl Pts',(-0.718109560493481,0.198658396328338,
-4.42575662869528));
#51744=CARTESIAN_POINT('Ctrl Pts',(-0.72575069923105,-0.16861916222521,
-4.40989911811935));
#51745=CARTESIAN_POINT('Ctrl Pts',(-0.556968277535239,-0.494906897429525,
-4.39404160754339));
#51746=CARTESIAN_POINT('Ctrl Pts',(-0.252791805685121,-0.700887153743271,
-4.37818409696747));
#51747=CARTESIAN_POINT('Ctrl Pts',(0.11283611285958,-0.73648795709002,-4.3623265863915));
#51748=CARTESIAN_POINT('Ctrl Pts',(0.451034572779929,-0.59305506781505,
-4.34646907581558));
#51749=CARTESIAN_POINT('Ctrl Pts',(0.679590526957342,-0.305455749616425,
-4.33061156523962));
#51750=CARTESIAN_POINT('Ctrl Pts',(0.742944049322229,0.0563971531247643,
-4.31475405466369));
#51751=CARTESIAN_POINT('Ctrl Pts',(0.625694460283858,0.4045404079619,-4.29889654408774));
#51752=CARTESIAN_POINT('Ctrl Pts',(0.356344095395492,0.654343476303278,
-4.2830390335118));
#51753=CARTESIAN_POINT('Ctrl Pts',(0.000369640284832444,0.745081447004251,
-4.26718152293585));
#51754=CARTESIAN_POINT('Ctrl Pts',(-0.355694671101819,0.654696723875764,
-4.25132401235991));
#51755=CARTESIAN_POINT('Ctrl Pts',(-0.625292761554132,0.405161031753915,
-4.23546650178396));
#51756=CARTESIAN_POINT('Ctrl Pts',(-0.742887725556159,0.0571342849949572,
-4.21960899120803));
#51757=CARTESIAN_POINT('Ctrl Pts',(-0.679893269963091,-0.304781299890241,
-4.20375148063208));
#51758=CARTESIAN_POINT('Ctrl Pts',(-0.451622788416938,-0.592607252981601,
-4.18789397005613));
#51759=CARTESIAN_POINT('Ctrl Pts',(-0.113566811121643,-0.736375636964961,
-4.17203645948019));
#51760=CARTESIAN_POINT('Ctrl Pts',(0.252096251067092,-0.701137632353168,
-4.15617894890425));
#51761=CARTESIAN_POINT('Ctrl Pts',(0.556476949722059,-0.49545928564507,
-4.1403214383283));
#51762=CARTESIAN_POINT('Ctrl Pts',(0.725583035657959,-0.169339179368713,
-4.12446392775236));
#51763=CARTESIAN_POINT('Ctrl Pts',(0.718306318688587,0.197945780040748,
-4.10860641717642));
#51764=CARTESIAN_POINT('Ctrl Pts',(0.536415704193378,0.51711187532159,-4.09274890660048));
#51765=CARTESIAN_POINT('Ctrl Pts',(0.224127187902907,0.710572658456983,
-4.07689139602453));
#51766=CARTESIAN_POINT('Ctrl Pts',(-0.142644660641527,0.731299528301743,
-4.06103388544859));
#51767=CARTESIAN_POINT('Ctrl Pts',(-0.474740856880215,0.574253966562295,
-4.04517637487265));
#51768=CARTESIAN_POINT('Ctrl Pts',(-0.691431759892533,0.277612356922026,
-4.0293188642967));
#51769=CARTESIAN_POINT('Ctrl Pts',(-0.740041732350872,-0.0865143553580023,
-4.01346135372077));
#51770=CARTESIAN_POINT('Ctrl Pts',(-0.608754120929568,-0.429610194892017,
-3.99760384314481));
#51771=CARTESIAN_POINT('Ctrl Pts',(-0.329483779961226,-0.668271604997811,
-3.98174633256888));
#51772=CARTESIAN_POINT('Ctrl Pts',(0.0298811466925253,-0.744482112865198,
-3.96588882199293));
#51773=CARTESIAN_POINT('Ctrl Pts',(0.381982231513381,-0.639715619718594,
-3.95003131141699));
#51774=CARTESIAN_POINT('Ctrl Pts',(0.641226822530954,-0.379439931175865,
-3.93417380084104));
#51775=CARTESIAN_POINT('Ctrl Pts',(0.74459485814713,-0.0269257595017122,
-3.9183162902651));
#51776=CARTESIAN_POINT('Ctrl Pts',(0.666958485370885,0.332133825581894,
-3.90245877968916));
#51777=CARTESIAN_POINT('Ctrl Pts',(0.427190418095336,0.610454622385171,
-3.88660126911321));
#51778=CARTESIAN_POINT('Ctrl Pts',(0.0835761476769501,0.740379312814297,
-3.87074375853727));
#51779=CARTESIAN_POINT('Ctrl Pts',(-0.280354743250511,0.690324356546131,
-3.85488624796132));
#51780=CARTESIAN_POINT('Ctrl Pts',(-0.576133881735919,0.472457669659188,
-3.83902873738538));
#51781=CARTESIAN_POINT('Ctrl Pts',(-0.731859981609243,0.139740712116434,
-3.82317122680944));
#51782=CARTESIAN_POINT('Ctrl Pts',(-0.709677408668316,-0.226945973592202,
-3.80731371623349));
#51783=CARTESIAN_POINT('Ctrl Pts',(-0.514978549723044,-0.538464105237332,
-3.79145620565755));
#51784=CARTESIAN_POINT('Ctrl Pts',(-0.195092971171135,-0.71908638695466,
-3.77559869508161));
#51785=CARTESIAN_POINT('Ctrl Pts',(0.172217978966369,-0.724905143466804,
-3.75974118450566));
#51786=CARTESIAN_POINT('Ctrl Pts',(0.497664265312189,-0.554505886655109,
-3.74388367392972));
#51787=CARTESIAN_POINT('Ctrl Pts',(0.702132781082156,-0.249311165080358,
-3.72802616335378));
#51788=CARTESIAN_POINT('Ctrl Pts',(0.735919042922848,0.116488890317527,
-3.71216865277783));
#51789=CARTESIAN_POINT('Ctrl Pts',(0.590809910131837,0.453971529276781,
-3.69631114220189));
#51790=CARTESIAN_POINT('Ctrl Pts',(0.302080126344257,0.681097714407944,
-3.68045363162595));
#51791=CARTESIAN_POINT('Ctrl Pts',(-0.0600826578968981,0.742655083820162,
-3.66459612105001));
#51792=CARTESIAN_POINT('Ctrl Pts',(-0.407639880699809,0.623679586780693,
-3.64873861047406));
#51793=CARTESIAN_POINT('Ctrl Pts',(-0.656103462664489,0.353093111775854,
-3.63288109989812));
#51794=CARTESIAN_POINT('Ctrl Pts',(-0.745074109908502,-0.00332716815676224,
-3.61702358932217));
#51795=CARTESIAN_POINT('Ctrl Pts',(-0.652923846905976,-0.358938643009346,
-3.60116607874623));
#51796=CARTESIAN_POINT('Ctrl Pts',(-0.402053585583011,-0.627295316118121,
-3.58530856817028));
#51797=CARTESIAN_POINT('Ctrl Pts',(-0.0534476622362749,-0.743162059516877,
-3.56945105759435));
#51798=CARTESIAN_POINT('Ctrl Pts',(0.308150913929887,-0.678372695166945,
-3.5535935470184));
#51799=CARTESIAN_POINT('Ctrl Pts',(0.594840735004374,-0.448676943115362,
-3.53773603644246));
#51800=CARTESIAN_POINT('Ctrl Pts',(0.736930047293309,-0.109911804189408,
-3.52187852586651));
#51801=CARTESIAN_POINT('Ctrl Pts',(0.699878198751708,0.255571919850272,
-3.50602101529057));
#51802=CARTESIAN_POINT('Ctrl Pts',(0.492692165256099,0.558928376090486,
-3.49016350471463));
#51803=CARTESIAN_POINT('Ctrl Pts',(0.165737034625333,0.72641429959596,-3.47430599413868));
#51804=CARTESIAN_POINT('Ctrl Pts',(-0.201507299688257,0.71731534730287,
-3.45844848356274));
#51805=CARTESIAN_POINT('Ctrl Pts',(-0.519766996023564,0.533843393841798,
-3.44259097298679));
#51806=CARTESIAN_POINT('Ctrl Pts',(-0.711675943911235,0.220598844425674,
-3.42673346241086));
#51807=CARTESIAN_POINT('Ctrl Pts',(-0.730582779596139,-0.146271328227603,
-3.4108759518349));
#51808=CARTESIAN_POINT('Ctrl Pts',(-0.571891418952435,-0.477584237839209,
-3.39501844125897));
#51809=CARTESIAN_POINT('Ctrl Pts',(-0.274178324785384,-0.692800653522907,
-3.37916093068302));
#51810=CARTESIAN_POINT('Ctrl Pts',(0.0901850892553483,-0.739603372747782,
-3.36330342010708));
#51811=CARTESIAN_POINT('Ctrl Pts',(0.432625307684578,-0.606615069426003,
-3.34744590953114));
#51812=CARTESIAN_POINT('Ctrl Pts',(0.669898149497886,-0.326164021012737,
-3.33158839895519));
#51813=CARTESIAN_POINT('Ctrl Pts',(0.744324690525857,0.0335746091187453,
-3.31573088837925));
#51814=CARTESIAN_POINT('Ctrl Pts',(0.637812498514814,0.38515154944798,-3.2998733778033));
#51815=CARTESIAN_POINT('Ctrl Pts',(0.376253742999091,0.643101562883393,
-3.28401586722737));
#51816=CARTESIAN_POINT('Ctrl Pts',(0.0232310384487809,0.744719288159291,
-3.26815835665141));
#51817=CARTESIAN_POINT('Ctrl Pts',(-0.335438925580633,0.665302357210013,
-3.25230084607548));
#51818=CARTESIAN_POINT('Ctrl Pts',(-0.612566660823242,0.424156321834006,
-3.23644333549953));
#51819=CARTESIAN_POINT('Ctrl Pts',(-0.740784871872864,0.0799016452158113,
-3.22058582492359));
#51820=CARTESIAN_POINT('Ctrl Pts',(-0.688924848413769,-0.283776412941517,
-3.20472831434764));
#51821=CARTESIAN_POINT('Ctrl Pts',(-0.46959330235475,-0.578470941091642,
-3.1888708037717));
#51822=CARTESIAN_POINT('Ctrl Pts',(-0.136107787935974,-0.732544312220813,
-3.17301329319576));
#51823=CARTESIAN_POINT('Ctrl Pts',(0.23046432299014,-0.708542655831381,
-3.15715578261981));
#51824=CARTESIAN_POINT('Ctrl Pts',(0.541012600308007,-0.512300561791472,
-3.14129827204387));
#51825=CARTESIAN_POINT('Ctrl Pts',(0.720045511141503,-0.191522743267892,
-3.12544076146793));
#51826=CARTESIAN_POINT('Ctrl Pts',(0.724041742183651,0.175812556091856,
-3.10958325089198));
#51827=CARTESIAN_POINT('Ctrl Pts',(0.552029845098931,0.500409381830454,
-3.09372574031604));
#51828=CARTESIAN_POINT('Ctrl Pts',(0.245824387000732,0.703361123505987,
-3.0778682297401));
#51829=CARTESIAN_POINT('Ctrl Pts',(-0.120138800083435,0.73533201209957,
-3.06201071916415));
#51830=CARTESIAN_POINT('Ctrl Pts',(-0.456897310025201,0.588550208049937,
-3.04615320858821));
#51831=CARTESIAN_POINT('Ctrl Pts',(-0.682588134779086,0.298697066545184,
-3.03029569801227));
#51832=CARTESIAN_POINT('Ctrl Pts',(-0.742347835835951,-0.0637666835704077,
-3.01443818743632));
#51833=CARTESIAN_POINT('Ctrl Pts',(-0.621649359702007,-0.410729318269314,
-2.99858067686038));
#51834=CARTESIAN_POINT('Ctrl Pts',(-0.349833435805405,-0.657847297247982,
-2.98272316628444));
#51835=CARTESIAN_POINT('Ctrl Pts',(0.0070238946910416,-0.745048430779676,
-2.96686565570849));
#51836=CARTESIAN_POINT('Ctrl Pts',(0.362173778662374,-0.651134896433379,
-2.95100814513255));
#51837=CARTESIAN_POINT('Ctrl Pts',(0.629282428095556,-0.398936241765586,
-2.9351506345566));
#51838=CARTESIAN_POINT('Ctrl Pts',(0.74341809851486,-0.0497597237174798,
-2.91929312398067));
#51839=CARTESIAN_POINT('Ctrl Pts',(0.676835420375122,0.31151294199362,-2.90343561340472));
#51840=CARTESIAN_POINT('Ctrl Pts',(0.445720052406056,0.597059573398696,
-2.88757810282878));
#51841=CARTESIAN_POINT('Ctrl Pts',(0.106254091478081,0.737466316076915,
-2.87172059225283));
#51842=CARTESIAN_POINT('Ctrl Pts',(-0.259041297032996,0.698601535737899,
-2.85586308167689));
#51843=CARTESIAN_POINT('Ctrl Pts',(-0.561366042911193,0.489912915904567,
-2.84000557110094));
#51844=CARTESIAN_POINT('Ctrl Pts',(-0.727227680863051,0.162130809812444,
-2.824148060525));
#51845=CARTESIAN_POINT('Ctrl Pts',(-0.716306717241799,-0.205063858683501,
-2.80829054994906));
#51846=CARTESIAN_POINT('Ctrl Pts',(-0.531257941477839,-0.522409321242087,
-2.79243303937311));
#51847=CARTESIAN_POINT('Ctrl Pts',(-0.217065070305726,-0.71276170951943,
-2.77657552879717));
#51848=CARTESIAN_POINT('Ctrl Pts',(0.149894394945637,-0.729848045601117,
-2.76071801822123));
#51849=CARTESIAN_POINT('Ctrl Pts',(0.480415861758509,-0.569514792674184,
-2.74486050764528));
#51850=CARTESIAN_POINT('Ctrl Pts',(0.694152491974035,-0.270737543000829,
-2.72900299706934));
#51851=CARTESIAN_POINT('Ctrl Pts',(0.739146805788744,0.0938536030005615,
-2.7131454864934));
#51852=CARTESIAN_POINT('Ctrl Pts',(0.604461084436589,0.435629770224248,
-2.69728797591746));
#51853=CARTESIAN_POINT('Ctrl Pts',(0.322836232646514,0.671508202626368,
-2.68143046534151));
#51854=CARTESIAN_POINT('Ctrl Pts',(-0.0372672450143224,0.744148944602444,
-2.66557295476557));
#51855=CARTESIAN_POINT('Ctrl Pts',(-0.388311385825831,0.635893675815314,
-2.64971544418962));
#51856=CARTESIAN_POINT('Ctrl Pts',(-0.644960471535362,0.373058292309355,
-2.63385793361369));
#51857=CARTESIAN_POINT('Ctrl Pts',(-0.744825384873282,0.019535745500423,
-2.61800042303773));
#51858=CARTESIAN_POINT('Ctrl Pts',(-0.663629850815514,-0.338735767834558,
-2.6021429124618));
#51859=CARTESIAN_POINT('Ctrl Pts',(-0.42111178380698,-0.614663619260805,
-2.58628540188585));
#51860=CARTESIAN_POINT('Ctrl Pts',(-0.076225175757575,-0.741172194489656,
-2.57042789130991));
#51861=CARTESIAN_POINT('Ctrl Pts',(0.287191096701467,-0.687508380515683,
-2.55457038073397));
#51862=CARTESIAN_POINT('Ctrl Pts',(0.580793759806059,-0.466717374729323,
-2.53871287015802));
#51863=CARTESIAN_POINT('Ctrl Pts',(0.733210609254479,-0.132471513090796,
-2.52285535958208));
#51864=CARTESIAN_POINT('Ctrl Pts',(0.707390460282839,0.233976998879638,
-2.50699784900613));
#51865=CARTESIAN_POINT('Ctrl Pts',(0.509609962183139,0.543547776876688,
-2.49114033843019));
#51866=CARTESIAN_POINT('Ctrl Pts',(0.187947800509531,0.720986909442548,
-2.47528282785425));
#51867=CARTESIAN_POINT('Ctrl Pts',(-0.179402805111352,0.723160516636568,
-2.4594253172783));
#51868=CARTESIAN_POINT('Ctrl Pts',(-0.50314217940581,0.54954021382121,-2.44356780670236));
#51869=CARTESIAN_POINT('Ctrl Pts',(-0.704572150775774,0.242331557282762,
-2.42771029612642));
#51870=CARTESIAN_POINT('Ctrl Pts',(-0.734726879071544,-0.123785752304851,
-2.41185278555047));
#51871=CARTESIAN_POINT('Ctrl Pts',(-0.586276017198065,-0.459811842999138,
-2.39599527497453));
#51872=CARTESIAN_POINT('Ctrl Pts',(-0.295306653502441,-0.684061751380004,
-2.38013776439859));
#51873=CARTESIAN_POINT('Ctrl Pts',(0.0674491394529376,-0.742022312933343,
-2.36428025382264));
#51874=CARTESIAN_POINT('Ctrl Pts',(0.413808644615465,-0.619603829027388,
-2.3484227432467));
#51875=CARTESIAN_POINT('Ctrl Pts',(0.659574937124499,-0.34656514772998,
-2.33256523267076));
#51876=CARTESIAN_POINT('Ctrl Pts',(0.745004410249938,0.01072044831298,-2.31670772209481));
#51877=CARTESIAN_POINT('Ctrl Pts',(0.649329916497877,0.365399998419196,
-2.30085021151887));
#51878=CARTESIAN_POINT('Ctrl Pts',(0.395809077043586,0.631254048568238,
-2.28499270094292));
#51879=CARTESIAN_POINT('Ctrl Pts',(0.0460705602272718,0.743655836247005,
-2.26913519036698));
#51880=CARTESIAN_POINT('Ctrl Pts',(-0.314867301315917,0.675281483431852,
-2.25327767979104));
#51881=CARTESIAN_POINT('Ctrl Pts',(-0.599263713541787,0.442752189080975,
-2.2374201692151));
#51882=CARTESIAN_POINT('Ctrl Pts',(-0.737984430114058,0.10259376303226,
-2.22156265863915));
#51883=CARTESIAN_POINT('Ctrl Pts',(-0.697307674740288,-0.262504297207077,
-2.20570514806321));
#51884=CARTESIAN_POINT('Ctrl Pts',(-0.487121606009267,-0.563789890174383,
-2.18984763748727));
#51885=CARTESIAN_POINT('Ctrl Pts',(-0.158520593707075,-0.728023159435637,
-2.17399012691132));
#51886=CARTESIAN_POINT('Ctrl Pts',(0.208615369472112,-0.715280453335545,
-2.15813261633538));
#51887=CARTESIAN_POINT('Ctrl Pts',(0.525038785929141,-0.528659410749439,
-2.14227510575943));
#51888=CARTESIAN_POINT('Ctrl Pts',(0.713829928552495,-0.213525952536522,
-2.12641759518349));
#51889=CARTESIAN_POINT('Ctrl Pts',(0.729095344404152,0.153513771603985,
-2.11056008460755));
#51890=CARTESIAN_POINT('Ctrl Pts',(0.567124146234676,0.483235658929967,
-2.0947025740316));
#51891=CARTESIAN_POINT('Ctrl Pts',(0.267290096272606,0.695487241966717,
-2.07884506345566));
#51892=CARTESIAN_POINT('Ctrl Pts',(-0.0975198062831407,0.7386720427134,
-2.06298755287972));
#51893=CARTESIAN_POINT('Ctrl Pts',(-0.438623508547968,0.602292218987561,
-2.04713004230377));
#51894=CARTESIAN_POINT('Ctrl Pts',(-0.673101724747398,0.319500496785165,
-2.03127253172783));
#51895=CARTESIAN_POINT('Ctrl Pts',(-0.743954879421426,-0.0409589634749339,
-2.01541502115189));
#51896=CARTESIAN_POINT('Ctrl Pts',(-0.633959198857162,-0.391461662858922,
-1.99955751057594));
#51897=CARTESIAN_POINT('Ctrl Pts',(-0.369853657771412,-0.646803502724741,
-1.9837));
#51898=CARTESIAN_POINT('Ctrl Pts',(-0.015839971626384,-0.744913145677242,
-1.96784248942406));
#51899=CARTESIAN_POINT('Ctrl Pts',(0.342024271182878,-0.661941007360709,
-1.95198497884811));
#51900=CARTESIAN_POINT('Ctrl Pts',(0.6167454460755,-0.418056878963882,-1.93612746827217));
#51901=CARTESIAN_POINT('Ctrl Pts',(0.741541271129677,-0.0725468298085624,
-1.92026995769623));
#51902=CARTESIAN_POINT('Ctrl Pts',(0.686074987722085,0.290598710468627,
-1.90441244712028));
#51903=CARTESIAN_POINT('Ctrl Pts',(0.463829957581682,0.583102280696676,
-1.88855493654435));
#51904=CARTESIAN_POINT('Ctrl Pts',(0.12883197709769,0.733858856307525,-1.87269742596839));
#51905=CARTESIAN_POINT('Ctrl Pts',(-0.237483914786634,0.706220850387119,
-1.85683991539246));
#51906=CARTESIAN_POINT('Ctrl Pts',(-0.546069572533108,0.506906817134467,
-1.84098240481651));
#51907=CARTESIAN_POINT('Ctrl Pts',(-0.721910558682716,0.184368230902995,
-1.82512489424057));
#51908=CARTESIAN_POINT('Ctrl Pts',(-0.722261488519323,-0.182988637641087,
-1.80926738366462));
#51909=CARTESIAN_POINT('Ctrl Pts',(-0.547037054111024,-0.505862590762966,
-1.79340987308868));
#51910=CARTESIAN_POINT('Ctrl Pts',(-0.238832761912019,-0.705765833078766,
-1.77755236251274));
#51911=CARTESIAN_POINT('Ctrl Pts',(0.12742965720205,-0.734103658735778,
-1.76169485193679));
#51912=CARTESIAN_POINT('Ctrl Pts',(0.462715056449375,-0.583987393561662,
-1.74583734136085));
#51913=CARTESIAN_POINT('Ctrl Pts',(0.685518527933592,-0.29190897068033,
-1.72997983078491));
#51914=CARTESIAN_POINT('Ctrl Pts',(0.741678523125974,0.0711299348907594,
-1.71412232020896));
#51915=CARTESIAN_POINT('Ctrl Pts',(0.617543045113172,0.416877783932221,
-1.69826480963302));
#51916=CARTESIAN_POINT('Ctrl Pts',(0.343288328007429,0.66128633976346,-1.68240729905708));
#51917=CARTESIAN_POINT('Ctrl Pts',(-0.0144167380217974,0.744942049402972,
-1.66654978848113));
#51918=CARTESIAN_POINT('Ctrl Pts',(-0.368617222857599,0.647508951533985,
-1.65069227790519));
#51919=CARTESIAN_POINT('Ctrl Pts',(-0.633210128999356,0.392672168400699,
-1.63483476732924));
#51920=CARTESIAN_POINT('Ctrl Pts',(-0.743875266860757,0.0423802625844482,
-1.6189772567533));
#51921=CARTESIAN_POINT('Ctrl Pts',(-0.673710922591512,-0.318213909320104,
-1.60311974617735));
#51922=CARTESIAN_POINT('Ctrl Pts',(-0.439773426202145,-0.601453101172749,
-1.58726223560142));
#51923=CARTESIAN_POINT('Ctrl Pts',(-0.0989309089608898,-0.738484376649947,
-1.57140472502547));
#51924=CARTESIAN_POINT('Ctrl Pts',(0.265960835121323,-0.69599664761079,
-1.55554721444953));
#51925=CARTESIAN_POINT('Ctrl Pts',(0.566199858210426,-0.484318304285913,
-1.53968970387358));
#51926=CARTESIAN_POINT('Ctrl Pts',(0.728800715730834,-0.15490647518458,
-1.52383219329764));
#51927=CARTESIAN_POINT('Ctrl Pts',(0.714236580848404,0.212161744623924,
-1.5079746827217));
#51928=CARTESIAN_POINT('Ctrl Pts',(0.526047865626554,0.527655325353243,
-1.49211717214575));
#51929=CARTESIAN_POINT('Ctrl Pts',(0.209981578243146,0.714880574713293,
-1.47625966156981));
#51930=CARTESIAN_POINT('Ctrl Pts',(-0.157129369101771,0.728324694535046,
-1.46040215099387));
#51931=CARTESIAN_POINT('Ctrl Pts',(-0.486043559936557,0.564719538486219,
-1.44454464041792));
#51932=CARTESIAN_POINT('Ctrl Pts',(-0.696804870642429,0.263836069469049,
-1.42868712984198));
#51933=CARTESIAN_POINT('Ctrl Pts',(-0.738179095209345,-0.101183608849463,
-1.41282961926604));
#51934=CARTESIAN_POINT('Ctrl Pts',(-0.600108526471472,-0.441606448956679,
-1.39697210869009));
#51935=CARTESIAN_POINT('Ctrl Pts',(-0.316156895546953,-0.674678676632072,
-1.38111459811415));
#51936=CARTESIAN_POINT('Ctrl Pts',(0.0446496736188302,-0.743742499760246,
-1.36525708753821));
#51937=CARTESIAN_POINT('Ctrl Pts',(0.39460230299459,-0.632009115262792,
-1.34939957696226));
#51938=CARTESIAN_POINT('Ctrl Pts',(0.648630611080299,-0.366639918276074,
-1.33354206638632));
#51939=CARTESIAN_POINT('Ctrl Pts',(0.744982568410704,-0.0121438078081822,
-1.31768455581038));
#51940=CARTESIAN_POINT('Ctrl Pts',(0.66023586842107,0.345304354670142,-1.30182704523443));
#51941=CARTESIAN_POINT('Ctrl Pts',(0.414991682509506,0.618812090017495,
-1.28596953465849));
#51942=CARTESIAN_POINT('Ctrl Pts',(0.0688666979212898,0.741892092707091,
-1.27011202408255));
#51943=CARTESIAN_POINT('Ctrl Pts',(-0.293999170355266,0.684624705319858,
-1.2542545135066));
#51944=CARTESIAN_POINT('Ctrl Pts',(-0.585396446932924,0.46093112199351,
-1.23839700293066));
#51945=CARTESIAN_POINT('Ctrl Pts',(-0.734489037421575,0.12518926955381,
-1.22253949235471));
#51946=CARTESIAN_POINT('Ctrl Pts',(-0.705033854937372,-0.240984984378776,
-1.20668198177877));
#51947=CARTESIAN_POINT('Ctrl Pts',(-0.504191193190784,-0.54857792519636,
-1.19082447120283));
#51948=CARTESIAN_POINT('Ctrl Pts',(-0.180784122569197,-0.722816436123844,
-1.17496696062689));
#51949=CARTESIAN_POINT('Ctrl Pts',(0.186569965405974,-0.721344679963956,
-1.15910945005094));
#51950=CARTESIAN_POINT('Ctrl Pts',(0.508570548931574,-0.544520427590487,
-1.143251939475));
#51951=CARTESIAN_POINT('Ctrl Pts',(0.706942141029221,-0.235328087020886,
-1.12739442889906));
#51952=CARTESIAN_POINT('Ctrl Pts',(0.733462366434538,0.131070425070409,
-1.11153691832311));
#51953=CARTESIAN_POINT('Ctrl Pts',(0.581684393481415,0.46560687890542,-1.09567940774717));
#51954=CARTESIAN_POINT('Ctrl Pts',(0.288504101722052,0.686958428577336,
-1.07982189717123));
#51955=CARTESIAN_POINT('Ctrl Pts',(-0.0748089792710891,0.741316474877164,
-1.06396438659528));
#51956=CARTESIAN_POINT('Ctrl Pts',(-0.419936660664375,0.615467058691158,
-1.04810687601934));
#51957=CARTESIAN_POINT('Ctrl Pts',(-0.662981463034035,0.340003057305575,
-1.03224936544339));
#51958=CARTESIAN_POINT('Ctrl Pts',(-0.744861349773961,-0.0181126728232756,
-1.01639185486745));
#51959=CARTESIAN_POINT('Ctrl Pts',(-0.64567204636971,-0.371825372776845,
-1.00053434429151));
#51960=CARTESIAN_POINT('Ctrl Pts',(-0.389525593060484,-0.635150621234654,
-0.984676833715565));
#51961=CARTESIAN_POINT('Ctrl Pts',(-0.0386889216357713,-0.744076384954227,
-0.968819323139621));
#51962=CARTESIAN_POINT('Ctrl Pts',(0.321552683620266,-0.672123776517757,
-0.952961812563677));
#51963=CARTESIAN_POINT('Ctrl Pts',(0.603627682393802,-0.436783837099971,
-0.937104301987736));
#51964=CARTESIAN_POINT('Ctrl Pts',(0.738966143377032,-0.0952656194351606,
-0.92124679141179));
#51965=CARTESIAN_POINT('Ctrl Pts',(0.694668486623927,0.269410825683588,
-0.905389280835849));
#51966=CARTESIAN_POINT('Ctrl Pts',(0.481503079745453,0.568595887691366,
-0.889531770259903));
#51967=CARTESIAN_POINT('Ctrl Pts',(0.15128854321635,0.729560330606979,-0.873674259683962));
#51968=CARTESIAN_POINT('Ctrl Pts',(-0.215702896835252,0.713175125478146,
-0.857816749108016));
#51969=CARTESIAN_POINT('Ctrl Pts',(-0.530258875101165,0.523423370399467,
-0.841959238532075));
#51970=CARTESIAN_POINT('Ctrl Pts',(-0.715913622137308,0.206432034680005,
-0.82610172795613));
#51971=CARTESIAN_POINT('Ctrl Pts',(-0.727536114965444,-0.160741098431234,
-0.810244217380188));
#51972=CARTESIAN_POINT('Ctrl Pts',(-0.562301028624769,-0.488839495654161,
-0.794386706804242));
#51973=CARTESIAN_POINT('Ctrl Pts',(-0.260375547620419,-0.698105345564161,
-0.778529196228302));
#51974=CARTESIAN_POINT('Ctrl Pts',(0.104844920505069,-0.737667975411821,
-0.762671685652355));
#51975=CARTESIAN_POINT('Ctrl Pts',(0.444578518017195,-0.597910060645851,
-0.746814175076414));
#51976=CARTESIAN_POINT('Ctrl Pts',(0.676239019459429,-0.312805511243711,
-0.730956664500469));
#51977=CARTESIAN_POINT('Ctrl Pts',(0.743511810847211,0.0483392845891503,
-0.715099153924527));
#51978=CARTESIAN_POINT('Ctrl Pts',(0.630043473038817,0.397733228917417,
-0.699241643348582));
#51979=CARTESIAN_POINT('Ctrl Pts',(0.363417152938314,0.65044175162277,-0.68338413277264));
#51980=CARTESIAN_POINT('Ctrl Pts',(0.00844734503701607,0.74503365136463,
-0.667526622196697));
#51981=CARTESIAN_POINT('Ctrl Pts',(-0.348575937548106,0.658514475973267,
-0.651669111620753));
#51982=CARTESIAN_POINT('Ctrl Pts',(-0.620863500210685,0.411916269902062,
-0.63581160104481));
#51983=CARTESIAN_POINT('Ctrl Pts',(-0.742224650585465,0.0651848706922794,
-0.619954090468866));
#51984=CARTESIAN_POINT('Ctrl Pts',(-0.68315756901167,-0.297392392649777,
-0.604096579892923));
#51985=CARTESIAN_POINT('Ctrl Pts',(-0.458020939327533,-0.587676202037661,
-0.588239069316978));
#51986=CARTESIAN_POINT('Ctrl Pts',(-0.121543480134323,-0.735101137082999,
-0.572381558741037));
#51987=CARTESIAN_POINT('Ctrl Pts',(0.244480121467758,-0.703829503154735,
-0.556524048165091));
#51988=CARTESIAN_POINT('Ctrl Pts',(0.551072773116448,-0.50146315720452,
-0.54066653758915));
#51989=CARTESIAN_POINT('Ctrl Pts',(0.723704519465442,-0.177195563740772,
-0.524809027013205));
#51990=CARTESIAN_POINT('Ctrl Pts',(0.720410113539927,0.190146700242023,
-0.508951516437263));
#51991=CARTESIAN_POINT('Ctrl Pts',(0.541990396213754,0.511265987247614,
-0.493094005861317));
#51992=CARTESIAN_POINT('Ctrl Pts',(0.231817618885443,0.708101045669594,
-0.477236495285376));
#51993=CARTESIAN_POINT('Ctrl Pts',(-0.134707966280404,0.732803017954034,
-0.461378984709431));
#51994=CARTESIAN_POINT('Ctrl Pts',(-0.468487239181182,0.579367073653829,
-0.445521474133488));
#51995=CARTESIAN_POINT('Ctrl Pts',(-0.688381417856275,0.28509213044415,
-0.429663963557544));
#51996=CARTESIAN_POINT('Ctrl Pts',(-0.740936177115086,-0.0784861820171191,
-0.413806452981602));
#51997=CARTESIAN_POINT('Ctrl Pts',(-0.613375920837422,-0.422985199523109,
-0.397948942405657));
#51998=CARTESIAN_POINT('Ctrl Pts',(-0.336709416558958,-0.664660265179164,
-0.382091431829715));
#51999=CARTESIAN_POINT('Ctrl Pts',(0.0218081618463334,-0.744762313402212,
-0.366233921253771));
#52000=CARTESIAN_POINT('Ctrl Pts',(0.375024368975919,-0.643819246122629,
-0.350376410677828));
#52001=CARTESIAN_POINT('Ctrl Pts',(0.637075477940402,-0.386369428685465,
-0.334518900101884));
#52002=CARTESIAN_POINT('Ctrl Pts',(0.744259184723121,-0.0349966278611624,
-0.318661389525941));
#52003=CARTESIAN_POINT('Ctrl Pts',(0.67052008594917,0.324883541256598,-0.302803878949998));
#52004=CARTESIAN_POINT('Ctrl Pts',(0.433783492115795,0.605787405169466,
-0.286946368374054));
#52005=CARTESIAN_POINT('Ctrl Pts',(0.091597991045355,0.739429715509674,
-0.271088857798111));
#52006=CARTESIAN_POINT('Ctrl Pts',(-0.272854196384765,0.693323230190796,
-0.255231347222167));
#52007=CARTESIAN_POINT('Ctrl Pts',(-0.570977895368302,0.478675990529267,
-0.239373836646224));
#52008=CARTESIAN_POINT('Ctrl Pts',(-0.730302032760444,0.147666908672949,
-0.22351632607028));
#52009=CARTESIAN_POINT('Ctrl Pts',(-0.712096020773603,-0.219238781524417,
-0.207658815494337));
#52010=CARTESIAN_POINT('Ctrl Pts',(-0.520786170522117,-0.532849287879404,
-0.191801304918392));
#52011=CARTESIAN_POINT('Ctrl Pts',(-0.202877055975114,-0.716929207912262,
-0.17594379434245));
#52012=CARTESIAN_POINT('Ctrl Pts',(0.164348180649151,-0.726729307650186,
-0.160086283766506));
#52013=CARTESIAN_POINT('Ctrl Pts',(0.491624745145442,-0.559869296311085,
-0.144228773190563));
#52014=CARTESIAN_POINT('Ctrl Pts',(0.699386001600128,-0.256907404440502,
-0.12837126261462));
#52015=CARTESIAN_POINT('Ctrl Pts',(0.737143841528523,0.108501282989102,
-0.112513752038677));
#52016=CARTESIAN_POINT('Ctrl Pts',(0.595686800836177,0.44754428626929,-0.0966562414627327));
#52017=CARTESIAN_POINT('Ctrl Pts',(0.309466356321048,0.67777345379719,-0.0807987308867902));
#52018=CARTESIAN_POINT('Ctrl Pts',(-0.0520692913751179,0.743282925452814,
-0.0649412203108465));
#52019=CARTESIAN_POINT('Ctrl Pts',(-0.284519228009777,0.666428047244306,
-0.0543695465935505));
#52020=CARTESIAN_POINT('Ctrl Pts',(-0.384580808941221,0.602564764849855,
-0.0490837097349027));
#52021=CARTESIAN_POINT('Ctrl Pts',(-0.325579286442189,0.678938089483059,
-5.8309162902651));
#52022=CARTESIAN_POINT('Ctrl Pts',(-0.438323380606369,0.624872568197468,
-5.82563045340645));
#52023=CARTESIAN_POINT('Ctrl Pts',(-0.636245805812322,0.459548685140943,
-5.81505877968916));
#52024=CARTESIAN_POINT('Ctrl Pts',(-0.778481470957093,0.0996097814034236,
-5.79920126911321));
#52025=CARTESIAN_POINT('Ctrl Pts',(-0.731463748292673,-0.284443019088282,
-5.78334375853727));
#52026=CARTESIAN_POINT('Ctrl Pts',(-0.506639730728544,-0.599399518035823,
-5.76748624796132));
#52027=CARTESIAN_POINT('Ctrl Pts',(-0.158652966906228,-0.768622281063247,
-5.75162873738538));
#52028=CARTESIAN_POINT('Ctrl Pts',(0.227899327720991,-0.751012576084023,
-5.73577122680944));
#52029=CARTESIAN_POINT('Ctrl Pts',(0.559052135017169,-0.550831824440762,
-5.7199137162335));
#52030=CARTESIAN_POINT('Ctrl Pts',(0.754303905755431,-0.216752091975169,
-5.70405620565754));
#52031=CARTESIAN_POINT('Ctrl Pts',(0.766191299277441,0.170019868316858,
-5.68819869508161));
#52032=CARTESIAN_POINT('Ctrl Pts',(0.591824271197026,0.515460627536713,
-5.67234118450566));
#52033=CARTESIAN_POINT('Ctrl Pts',(0.273590066173409,0.735597928042492,
-5.65648367392972));
#52034=CARTESIAN_POINT('Ctrl Pts',(-0.111151487059797,0.776917663859421,
-5.64062616335378));
#52035=CARTESIAN_POINT('Ctrl Pts',(-0.468873084526362,0.629375721659158,
-5.62476865277783));
#52036=CARTESIAN_POINT('Ctrl Pts',(-0.712615799746851,0.328838061265476,
-5.60891114220189));
#52037=CARTESIAN_POINT('Ctrl Pts',(-0.783127928281117,-0.0516371854324633,
-5.59305363162595));
#52038=CARTESIAN_POINT('Ctrl Pts',(-0.663268602687365,-0.419559905984642,
-5.57719612105));
#52039=CARTESIAN_POINT('Ctrl Pts',(-0.382174559347619,-0.68549132513945,
-5.56133861047406));
#52040=CARTESIAN_POINT('Ctrl Pts',(-0.00817726953152785,-0.784785884905202,
-5.54548109989812));
#52041=CARTESIAN_POINT('Ctrl Pts',(0.367807842272825,-0.693305951887881,
-5.52962358932217));
#52042=CARTESIAN_POINT('Ctrl Pts',(0.654382128491452,-0.433289489945468,
-5.51376607874623));
#52043=CARTESIAN_POINT('Ctrl Pts',(0.781881921134958,-0.067944194012094,
-5.49790856817029));
#52044=CARTESIAN_POINT('Ctrl Pts',(0.719313150927466,0.313917732803588,
-5.48205105759434));
#52045=CARTESIAN_POINT('Ctrl Pts',(0.481885731221726,0.61946904213411,-5.4661935470184));
#52046=CARTESIAN_POINT('Ctrl Pts',(0.127316162674759,0.774432919497292,
-5.45033603644246));
#52047=CARTESIAN_POINT('Ctrl Pts',(-0.258202836220851,0.741139020338087,
-5.43447852586652));
#52048=CARTESIAN_POINT('Ctrl Pts',(-0.580955014875615,0.527680796298617,
-5.41862101529056));
#52049=CARTESIAN_POINT('Ctrl Pts',(-0.762482180195239,0.185948049138887,
-5.40276350471463));
#52050=CARTESIAN_POINT('Ctrl Pts',(-0.758656687723272,-0.200987020144955,
-5.38690599413869));
#52051=CARTESIAN_POINT('Ctrl Pts',(-0.570408480761624,-0.539063926792038,
-5.37104848356273));
#52052=CARTESIAN_POINT('Ctrl Pts',(-0.243499029403163,-0.746099172210769,
-5.3551909729868));
#52053=CARTESIAN_POINT('Ctrl Pts',(0.142602877126142,-0.771764323824862,
-5.33933346241085));
#52054=CARTESIAN_POINT('Ctrl Pts',(0.49403928855179,-0.609820410826756,
-5.3234759518349));
#52055=CARTESIAN_POINT('Ctrl Pts',(0.725379129112798,-0.299634562661213,
-5.30761844125897));
#52056=CARTESIAN_POINT('Ctrl Pts',(0.780385734641799,0.0833897911089845,
-5.29176093068301));
#52057=CARTESIAN_POINT('Ctrl Pts',(0.645687487026613,0.446142825999577,
-5.27590342010709));
#52058=CARTESIAN_POINT('Ctrl Pts',(0.354028336019651,0.700442495418987,
-5.26004590953113));
#52059=CARTESIAN_POINT('Ctrl Pts',(-0.0236919646369996,0.784470804367675,
-5.2441883989552));
#52060=CARTESIAN_POINT('Ctrl Pts',(-0.39565295874479,0.677801215940276,
-5.22833088837924));
#52061=CARTESIAN_POINT('Ctrl Pts',(-0.671434226464838,0.406364161344466,
-5.21247337780331));
#52062=CARTESIAN_POINT('Ctrl Pts',(-0.783995786707833,0.0361435819750997,
-5.19661586722736));
#52063=CARTESIAN_POINT('Ctrl Pts',(-0.705974922156322,-0.342863181721224,
-5.18075835665142));
#52064=CARTESIAN_POINT('Ctrl Pts',(-0.45633781324506,-0.638522945786869,
-5.16490084607547));
#52065=CARTESIAN_POINT('Ctrl Pts',(-0.0957690278526387,-0.778963442914869,
-5.14904333549954));
#52066=CARTESIAN_POINT('Ctrl Pts',(0.288080359116754,-0.730044833407365,
-5.13318582492359));
#52067=CARTESIAN_POINT('Ctrl Pts',(0.601899964922791,-0.503658797520275,
-5.11732831434764));
#52068=CARTESIAN_POINT('Ctrl Pts',(0.769403025737667,-0.154837773425435,
-5.1014708037717));
#52069=CARTESIAN_POINT('Ctrl Pts',(0.749871032569584,0.231622940588045,
-5.08561329319576));
#52070=CARTESIAN_POINT('Ctrl Pts',(0.548052039785859,0.5617781713276,-5.06975578261982));
#52071=CARTESIAN_POINT('Ctrl Pts',(0.213006455192798,0.755370109376738,
-5.05389827204387));
#52072=CARTESIAN_POINT('Ctrl Pts',(-0.173819110129491,0.765338270993563,
-5.03804076146793));
#52073=CARTESIAN_POINT('Ctrl Pts',(-0.518390790870064,0.589259484467356,
-5.02218325089199));
#52074=CARTESIAN_POINT('Ctrl Pts',(-0.7369462664343,0.269936941677441,-5.00632574031604));
#52075=CARTESIAN_POINT('Ctrl Pts',(-0.776356638438626,-0.115004878356971,
-4.9904682297401));
#52076=CARTESIAN_POINT('Ctrl Pts',(-0.627041594863537,-0.471990032103027,
-4.97461071916415));
#52077=CARTESIAN_POINT('Ctrl Pts',(-0.32529829896591,-0.714238593737072,
-4.95875320858822));
#52078=CARTESIAN_POINT('Ctrl Pts',(0.055522129295891,-0.7828620857163,-4.94289569801226));
#52079=CARTESIAN_POINT('Ctrl Pts',(0.422845620188429,-0.6611787455606,-4.92703818743633));
#52080=CARTESIAN_POINT('Ctrl Pts',(0.687379089788056,-0.378768714409952,
-4.91118067686037));
#52081=CARTESIAN_POINT('Ctrl Pts',(0.784816797004884,-0.00428336697262591,
-4.89532316628444));
#52082=CARTESIAN_POINT('Ctrl Pts',(0.691472499103114,0.371243228999155,
-4.87946565570849));
#52083=CARTESIAN_POINT('Ctrl Pts',(0.43003736730647,0.656523887466211,-4.86360814513256));
#52084=CARTESIAN_POINT('Ctrl Pts',(0.0640639642549887,0.782209409670812,
-4.8477506345566));
#52085=CARTESIAN_POINT('Ctrl Pts',(-0.317482820511887,0.71774675950048,
-4.83189312398067));
#52086=CARTESIAN_POINT('Ctrl Pts',(-0.621852346434259,0.47880623568186,
-4.81603561340471));
#52087=CARTESIAN_POINT('Ctrl Pts',(-0.775055080319058,0.123472161094084,
-4.80017810282878));
#52088=CARTESIAN_POINT('Ctrl Pts',(-0.739848795863616,-0.261876901143998,
-4.78432059225283));
#52089=CARTESIAN_POINT('Ctrl Pts',(-0.524791828677996,-0.583566010530454,
-4.76846308167689));
#52090=CARTESIAN_POINT('Ctrl Pts',(-0.182162620776919,-0.763395396688577,
-4.75260557110095));
#52091=CARTESIAN_POINT('Ctrl Pts',(0.204748705170189,-0.757650130221566,
-4.736748060525));
#52092=CARTESIAN_POINT('Ctrl Pts',(0.541887436204854,-0.567726834469673,
-4.72089054994906));
#52093=CARTESIAN_POINT('Ctrl Pts',(0.747298135904977,-0.239794178758729,
-4.70503303937311));
#52094=CARTESIAN_POINT('Ctrl Pts',(0.771047284357168,0.146430315778737,
-4.68917552879717));
#52095=CARTESIAN_POINT('Ctrl Pts',(0.607361674134095,0.497058898810449,
-4.67331801822123));
#52096=CARTESIAN_POINT('Ctrl Pts',(0.296031825834439,0.726856870495665,
-4.65746050764529));
#52097=CARTESIAN_POINT('Ctrl Pts',(-0.0872607346894568,0.77996238132046,
-4.64160299706934));
#52098=CARTESIAN_POINT('Ctrl Pts',(-0.449340984269311,0.643465952439997,
-4.6257454864934));
#52099=CARTESIAN_POINT('Ctrl Pts',(-0.702190424457694,0.350548655529511,
-4.60988797591746));
#52100=CARTESIAN_POINT('Ctrl Pts',(-0.784343598123281,-0.0275839115545715,
-4.59403046534151));
#52101=CARTESIAN_POINT('Ctrl Pts',(-0.675829797122982,-0.399011074300369,
-4.57817295476558));
#52102=CARTESIAN_POINT('Ctrl Pts',(-0.403027764390032,-0.673442182540117,
-4.56231544418962));
#52103=CARTESIAN_POINT('Ctrl Pts',(-0.0322532554024553,-0.784165466983575,
-4.54645793361368));
#52104=CARTESIAN_POINT('Ctrl Pts',(0.346361734014141,-0.704265078861889,
-4.53060042303774));
#52105=CARTESIAN_POINT('Ctrl Pts',(0.64077925675603,-0.453164094125754,
-4.5147429124618));
#52106=CARTESIAN_POINT('Ctrl Pts',(0.779429023368258,-0.0919029358879742,
-4.49888540188585));
#52107=CARTESIAN_POINT('Ctrl Pts',(0.728606504864627,0.291699011247172,
-4.48302789130991));
#52108=CARTESIAN_POINT('Ctrl Pts',(0.500666204897841,0.604391514969245,
-4.46717038073396));
#52109=CARTESIAN_POINT('Ctrl Pts',(0.15101838945731,0.7701617999741,-4.45131287015803));
#52110=CARTESIAN_POINT('Ctrl Pts',(-0.235340657522096,0.748712579706453,
-4.43545535958207));
#52111=CARTESIAN_POINT('Ctrl Pts',(-0.564490477202418,0.545257969443283,
-4.41959784900614));
#52112=CARTESIAN_POINT('Ctrl Pts',(-0.756417666681617,0.209255981098659,
-4.40374033843019));
#52113=CARTESIAN_POINT('Ctrl Pts',(-0.7644664278354,-0.177614280974837,
-4.38788282785425));
#52114=CARTESIAN_POINT('Ctrl Pts',(-0.586680178188085,-0.521308086082331,
-4.3720253172783));
#52115=CARTESIAN_POINT('Ctrl Pts',(-0.266277178765265,-0.738276517412301,
-4.35616780670236));
#52116=CARTESIAN_POINT('Ctrl Pts',(0.118855441985783,-0.775776472963695,
-4.34031029612641));
#52117=CARTESIAN_POINT('Ctrl Pts',(0.475095358569639,-0.624692046018845,
-4.32445278555048));
#52118=CARTESIAN_POINT('Ctrl Pts',(0.715843805709462,-0.321750521244362,
-4.30859527497453));
#52119=CARTESIAN_POINT('Ctrl Pts',(0.782576970395889,0.0594057025850026,
-4.29273776439859));
#52120=CARTESIAN_POINT('Ctrl Pts',(0.659072611953929,0.426120926810512,
-4.27688025382264));
#52121=CARTESIAN_POINT('Ctrl Pts',(0.375353544923698,0.689249931742353,
-4.2610227432467));
#52122=CARTESIAN_POINT('Ctrl Pts',(0.000389359029796799,0.784828389199302,
-4.24516523267075));
#52123=CARTESIAN_POINT('Ctrl Pts',(-0.374669476592169,0.689622023577971,
-4.22930772209482));
#52124=CARTESIAN_POINT('Ctrl Pts',(-0.658649484296868,0.426774658255496,
-4.21345021151887));
#52125=CARTESIAN_POINT('Ctrl Pts',(-0.782517641995249,0.0601821573211011,
-4.19759270094293));
#52126=CARTESIAN_POINT('Ctrl Pts',(-0.71616269877343,-0.321040092479401,
-4.18173519036698));
#52127=CARTESIAN_POINT('Ctrl Pts',(-0.47571495302169,-0.624220342159077,
-4.16587767979104));
#52128=CARTESIAN_POINT('Ctrl Pts',(-0.119625119907983,-0.775658161035277,
-4.15002016921509));
#52129=CARTESIAN_POINT('Ctrl Pts',(0.26554451925179,-0.738540357996068,
-4.13416265863915));
#52130=CARTESIAN_POINT('Ctrl Pts',(0.586162640115255,-0.521889941871598,
-4.11830514806321));
#52131=CARTESIAN_POINT('Ctrl Pts',(0.764289820120199,-0.178372707986,-4.10244763748727));
#52132=CARTESIAN_POINT('Ctrl Pts',(0.756624921093796,0.208505349747752,
-4.08659012691132));
#52133=CARTESIAN_POINT('Ctrl Pts',(0.565031212031903,0.544697605578897,
-4.07073261633538));
#52134=CARTESIAN_POINT('Ctrl Pts',(0.236083424926029,0.748478702815799,
-4.05487510575943));
#52135=CARTESIAN_POINT('Ctrl Pts',(-0.150254149649408,0.770311263455727,
-4.0390175951835));
#52136=CARTESIAN_POINT('Ctrl Pts',(-0.500066272607472,0.604887985575921,
-4.02316008460754));
#52137=CARTESIAN_POINT('Ctrl Pts',(-0.728316718312543,0.292421801376152,
-4.00730257403161));
#52138=CARTESIAN_POINT('Ctrl Pts',(-0.779519827096005,-0.0911295301087435,
-3.99144506345566));
#52139=CARTESIAN_POINT('Ctrl Pts',(-0.641228577182465,-0.452528080784138,
-3.97558755287972));
#52140=CARTESIAN_POINT('Ctrl Pts',(-0.347060345327305,-0.703921067162304,
-3.95973004230377));
#52141=CARTESIAN_POINT('Ctrl Pts',(0.0314751794188634,-0.784197083120166,
-3.94387253172783));
#52142=CARTESIAN_POINT('Ctrl Pts',(0.402359367109157,-0.673841740910389,
-3.92801502115189));
#52143=CARTESIAN_POINT('Ctrl Pts',(0.675433559997749,-0.399681445807019,
-3.91215751057594));
#52144=CARTESIAN_POINT('Ctrl Pts',(0.78431584288578,-0.0283621348278897,
-3.8963));
#52145=CARTESIAN_POINT('Ctrl Pts',(0.702537898160078,0.349851759667497,
-3.88044248942406));
#52146=CARTESIAN_POINT('Ctrl Pts',(0.449979219135252,0.643019793194622,
-3.86458497884811));
#52147=CARTESIAN_POINT('Ctrl Pts',(0.0880345814816758,0.779875416048597,
-3.84872746827217));
#52148=CARTESIAN_POINT('Ctrl Pts',(-0.295310482410159,0.727150239683866,
-3.83286995769623));
#52149=CARTESIAN_POINT('Ctrl Pts',(-0.606868186268723,0.497661287010088,
-3.81701244712028));
#52150=CARTESIAN_POINT('Ctrl Pts',(-0.770901614575481,0.147195287759293,
-3.80115493654434));
#52151=CARTESIAN_POINT('Ctrl Pts',(-0.747535695239384,-0.239052580903443,
-3.7852974259684));
#52152=CARTESIAN_POINT('Ctrl Pts',(-0.542450476087375,-0.567188886603224,
-3.76943991539245));
#52153=CARTESIAN_POINT('Ctrl Pts',(-0.205500355597327,-0.757446602700809,
-3.75358240481651));
#52154=CARTESIAN_POINT('Ctrl Pts',(0.181405079359823,-0.763575765249318,
-3.73772489424057));
#52155=CARTESIAN_POINT('Ctrl Pts',(0.524212547873029,-0.584086429174735,
-3.72186738366462));
#52156=CARTESIAN_POINT('Ctrl Pts',(0.739588593698525,-0.262610860713459,
-3.70600987308868));
#52157=CARTESIAN_POINT('Ctrl Pts',(0.775177209633211,0.122703079663451,
-3.69015236251273));
#52158=CARTESIAN_POINT('Ctrl Pts',(0.62232711867419,0.478188989267114,-3.67429485193679));
#52159=CARTESIAN_POINT('Ctrl Pts',(0.318194822755437,0.717431395232506,
-3.65843734136085));
#52160=CARTESIAN_POINT('Ctrl Pts',(-0.0632878134405744,0.782272589807117,
-3.6425798307849));
#52161=CARTESIAN_POINT('Ctrl Pts',(-0.429385743302777,0.656950253475823,
-3.62672232020896));
#52162=CARTESIAN_POINT('Ctrl Pts',(-0.691103805928104,0.37192913508532,
-3.61086480963302));
#52163=CARTESIAN_POINT('Ctrl Pts',(-0.784820660700543,-0.00350465849816745,
-3.59500729905707));
#52164=CARTESIAN_POINT('Ctrl Pts',(-0.687754571124228,-0.378086500673265,
-3.57914978848113));
#52165=CARTESIAN_POINT('Ctrl Pts',(-0.423501442981327,-0.660758866672525,
-3.56329227790519));
#52166=CARTESIAN_POINT('Ctrl Pts',(-0.0562988688391297,-0.782806610511855,
-3.54743476732924));
#52167=CARTESIAN_POINT('Ctrl Pts',(0.324589461168678,-0.714561007746612,
-3.5315772567533));
#52168=CARTESIAN_POINT('Ctrl Pts',(0.626572970996214,-0.472611959339373,
-3.51571974617736));
#52169=CARTESIAN_POINT('Ctrl Pts',(0.776242146808514,-0.115775133823011,
-3.49986223560142));
#52170=CARTESIAN_POINT('Ctrl Pts',(0.737213738941585,0.269205600256372,
-3.48400472502547));
#52171=CARTESIAN_POINT('Ctrl Pts',(0.518975207319653,0.588744839706599,
-3.46814721444953));
#52172=CARTESIAN_POINT('Ctrl Pts',(0.174578404063956,0.765165428471587,
-3.45228970387358));
#52173=CARTESIAN_POINT('Ctrl Pts',(-0.212256861396975,0.7555810855782,-3.43643219329765));
#52174=CARTESIAN_POINT('Ctrl Pts',(-0.5474943657345,0.562321679808455,-3.42057468272169));
#52175=CARTESIAN_POINT('Ctrl Pts',(-0.749640843880201,0.232366859255372,
-3.40471717214576));
#52176=CARTESIAN_POINT('Ctrl Pts',(-0.769556279239784,-0.15407428460403,
-3.38885966156981));
#52177=CARTESIAN_POINT('Ctrl Pts',(-0.602399406048799,-0.503061335908134,
-3.37300215099387));
#52178=CARTESIAN_POINT('Ctrl Pts',(-0.288804578157005,-0.729758636625274,
-3.35714464041792));
#52179=CARTESIAN_POINT('Ctrl Pts',(0.0949960821258639,-0.779058082863121,
-3.34128712984198));
#52180=CARTESIAN_POINT('Ctrl Pts',(0.455704037084961,-0.638975416333128,
-3.32542961926604));
#52181=CARTESIAN_POINT('Ctrl Pts',(0.705634380928318,-0.343563491287323,
-3.3095721086901));
#52182=CARTESIAN_POINT('Ctrl Pts',(0.784031262965194,0.0353656724356925,
-3.29371459811415));
#52183=CARTESIAN_POINT('Ctrl Pts',(0.671837096243931,0.405697754743786,
-3.27785708753821));
#52184=CARTESIAN_POINT('Ctrl Pts',(0.396325287974185,0.67740830981455,-3.26199957696226));
#52185=CARTESIAN_POINT('Ctrl Pts',(0.024470316041941,0.784446910712531,
-3.24614206638632));
#52186=CARTESIAN_POINT('Ctrl Pts',(-0.353333172764794,0.700793422570154,
-3.23028455581038));
#52187=CARTESIAN_POINT('Ctrl Pts',(-0.645244499945733,0.446783266677934,
-3.21442704523443));
#52188=CARTESIAN_POINT('Ctrl Pts',(-0.780302609966712,0.084164059863832,
-3.19856953465849));
#52189=CARTESIAN_POINT('Ctrl Pts',(-0.72567607371502,-0.298914683699512,
-3.18271202408255));
#52190=CARTESIAN_POINT('Ctrl Pts',(-0.494644117831261,-0.609329917851207,
-3.1668545135066));
#52191=CARTESIAN_POINT('Ctrl Pts',(-0.143368562447453,-0.771622451329261,
-3.15099700293066));
#52192=CARTESIAN_POINT('Ctrl Pts',(0.242758619352965,-0.746340408140593,
-3.13513949235471));
#52193=CARTESIAN_POINT('Ctrl Pts',(0.569873333101313,-0.539629628832245,
-3.11928198177877));
#52194=CARTESIAN_POINT('Ctrl Pts',(0.75845689210424,-0.201739671143779,
-3.10342447120283));
#52195=CARTESIAN_POINT('Ctrl Pts',(0.762666305161411,0.185191411963582,
-3.08756696062689));
#52196=CARTESIAN_POINT('Ctrl Pts',(0.581478301279538,0.527104104740881,
-3.07170945005094));
#52197=CARTESIAN_POINT('Ctrl Pts',(0.258938077778477,0.740882462992621,
-3.055851939475));
#52198=CARTESIAN_POINT('Ctrl Pts',(-0.126547696669843,0.774558863199681,
-3.03999442889905));
#52199=CARTESIAN_POINT('Ctrl Pts',(-0.481270848037274,0.619946871048728,
-3.02413691832312));
#52200=CARTESIAN_POINT('Ctrl Pts',(-0.719001323223353,0.314631291032365,
-3.00827940774716));
#52201=CARTESIAN_POINT('Ctrl Pts',(-0.781948951443148,-0.0671683662938689,
-2.99242189717123));
#52202=CARTESIAN_POINT('Ctrl Pts',(-0.654811722373912,-0.432639989292871,
-2.97656438659528));
#52203=CARTESIAN_POINT('Ctrl Pts',(-0.368495569196001,-0.692940666707143,
-2.96070687601934));
#52204=CARTESIAN_POINT('Ctrl Pts',(0.00739858974940715,-0.784793611698863,
-2.94484936544339));
#52205=CARTESIAN_POINT('Ctrl Pts',(0.381494217123079,-0.685870187714319,
-2.92899185486745));
#52206=CARTESIAN_POINT('Ctrl Pts',(0.662851982664983,-0.42021780206308,
-2.91313434429151));
#52207=CARTESIAN_POINT('Ctrl Pts',(0.783076308106886,-0.0524141944068109,
-2.89727683371557));
#52208=CARTESIAN_POINT('Ctrl Pts',(0.712941725850017,0.328130839202329,
-2.88141932313962));
#52209=CARTESIAN_POINT('Ctrl Pts',(0.469497331023564,0.628910175029293,
-2.86556181256368));
#52210=CARTESIAN_POINT('Ctrl Pts',(0.11192229761708,0.776807023262366,-2.84970430198773));
#52211=CARTESIAN_POINT('Ctrl Pts',(-0.272860054030235,0.735868971358516,
-2.83384679141179));
#52212=CARTESIAN_POINT('Ctrl Pts',(-0.591312545736583,0.516047696776321,
-2.81798928083585));
#52213=CARTESIAN_POINT('Ctrl Pts',(-0.766022200187245,0.170779802417963,
-2.80213177025991));
#52214=CARTESIAN_POINT('Ctrl Pts',(-0.754518649371647,-0.216003147764127,
-2.78627425968396));
#52215=CARTESIAN_POINT('Ctrl Pts',(-0.559598304501882,-0.550277647821756,
-2.77041674910802));
#52216=CARTESIAN_POINT('Ctrl Pts',(-0.228644573240195,-0.750784530488898,
-2.75455923853207));
#52217=CARTESIAN_POINT('Ctrl Pts',(0.157890626599538,-0.768782350295342,
-2.73870172795613));
#52218=CARTESIAN_POINT('Ctrl Pts',(0.506044014980788,-0.599895996815906,
-2.72284421738018));
#52219=CARTESIAN_POINT('Ctrl Pts',(0.73118258993712,-0.285180245224791,
-2.70698670680425));
#52220=CARTESIAN_POINT('Ctrl Pts',(0.778577159988897,0.0988602955551302,
-2.6911291962283));
#52221=CARTESIAN_POINT('Ctrl Pts',(0.636706525359668,0.458868774986972,
-2.67527168565236));
#52222=CARTESIAN_POINT('Ctrl Pts',(0.340058179494149,0.707330323577854,
-2.65941417507641));
#52223=CARTESIAN_POINT('Ctrl Pts',(-0.039255294829966,0.783846141740481,
-2.64355666450047));
#52224=CARTESIAN_POINT('Ctrl Pts',(-0.409026155020739,0.669815912473402,
-2.62769915392453));
#52225=CARTESIAN_POINT('Ctrl Pts',(-0.679366383376654,0.392959373512518,
-2.61184164334858));
#52226=CARTESIAN_POINT('Ctrl Pts',(-0.784558667237237,0.0205778948523656,
-2.59598413277264));
#52227=CARTESIAN_POINT('Ctrl Pts',(-0.699031695037147,-0.356805887601535,
-2.5801266221967));
#52228=CARTESIAN_POINT('Ctrl Pts',(-0.443576315430907,-0.647453322242124,
-2.56426911162075));
#52229=CARTESIAN_POINT('Ctrl Pts',(-0.0802914663179188,-0.780710594606057,
-2.54841160104481));
#52230=CARTESIAN_POINT('Ctrl Pts',(0.302511526387946,-0.724184043248715,
-2.53255409046886));
#52231=CARTESIAN_POINT('Ctrl Pts',(0.611776649114439,-0.49161477163724,
-2.51669657989292));
#52232=CARTESIAN_POINT('Ctrl Pts',(0.772324292490064,-0.139538307727111,
-2.50083906931698));
#52233=CARTESIAN_POINT('Ctrl Pts',(0.745126747835348,0.246458681636383,
-2.48498155874104));
#52234=CARTESIAN_POINT('Ctrl Pts',(0.536795497120767,0.572543750611684,
-2.46912404816509));
#52235=CARTESIAN_POINT('Ctrl Pts',(0.197974020317544,0.75944851002088,-2.45326653758915));
#52236=CARTESIAN_POINT('Ctrl Pts',(-0.188973185575212,0.761738069960523,
-2.4374090270132));
#52237=CARTESIAN_POINT('Ctrl Pts',(-0.52998268550235,0.578855858708663,
-2.42155151643726));
#52238=CARTESIAN_POINT('Ctrl Pts',(-0.742158093442481,0.255258920375855,
-2.40569400586132));
#52239=CARTESIAN_POINT('Ctrl Pts',(-0.773921448885386,-0.130389198359262,
-2.38983649528537));
#52240=CARTESIAN_POINT('Ctrl Pts',(-0.617551361738728,-0.484340859011778,
-2.37397898470943));
#52241=CARTESIAN_POINT('Ctrl Pts',(-0.311060013801192,-0.720553551033945,
-2.35812147413349));
#52242=CARTESIAN_POINT('Ctrl Pts',(0.0710472656144783,-0.781606063271219,
-2.34226396355755));
#52243=CARTESIAN_POINT('Ctrl Pts',(0.435883584668632,-0.65265707129399,
-2.3264064529816));
#52244=CARTESIAN_POINT('Ctrl Pts',(0.694760468860123,-0.365052931782348,
-2.31054894240566));
#52245=CARTESIAN_POINT('Ctrl Pts',(0.784747242860147,0.0112923388641639,
-2.29469143182971));
#52246=CARTESIAN_POINT('Ctrl Pts',(0.683968919737491,0.384892542051355,
-2.27883392125377));
#52247=CARTESIAN_POINT('Ctrl Pts',(0.416923816336558,0.664928780746467,
-2.26297641067783));
#52248=CARTESIAN_POINT('Ctrl Pts',(0.0485282296560387,0.783326728140994,
-2.24711890010188));
#52249=CARTESIAN_POINT('Ctrl Pts',(-0.331664139399642,0.711304892946703,
-2.23126138952594));
#52250=CARTESIAN_POINT('Ctrl Pts',(-0.631231896721636,0.466371144749363,
-2.21540387895));
#52251=CARTESIAN_POINT('Ctrl Pts',(-0.777352776490858,0.10806670613829,
-2.19954636837406));
#52252=CARTESIAN_POINT('Ctrl Pts',(-0.734506088351986,-0.276507790609034,
-2.18368885779811));
#52253=CARTESIAN_POINT('Ctrl Pts',(-0.513107482310247,-0.593865694994133,
-2.16783134722217));
#52254=CARTESIAN_POINT('Ctrl Pts',(-0.166976996560925,-0.766860114175407,
-2.15197383664622));
#52255=CARTESIAN_POINT('Ctrl Pts',(0.219744116624184,-0.753437638628893,
-2.13611632607028));
#52256=CARTESIAN_POINT('Ctrl Pts',(0.553047383322612,-0.556861153155467,
-2.12025881549434));
#52257=CARTESIAN_POINT('Ctrl Pts',(0.751909734486935,-0.224916658514685,
-2.10440130491839));
#52258=CARTESIAN_POINT('Ctrl Pts',(0.767989495674767,0.161703081686291,
-2.08854379434245));
#52259=CARTESIAN_POINT('Ctrl Pts',(0.597377819505481,0.509014236398652,
-2.07268628376651));
#52260=CARTESIAN_POINT('Ctrl Pts',(0.281548891802369,0.732588543193575,
-2.05682877319056));
#52261=CARTESIAN_POINT('Ctrl Pts',(-0.102722075268358,0.778077070312567,
-2.04097126261462));
#52262=CARTESIAN_POINT('Ctrl Pts',(-0.462022216581493,0.634421960117041,
-2.02511375203867));
#52263=CARTESIAN_POINT('Ctrl Pts',(-0.709008853360644,0.336544496240616,
-2.00925624146273));
#52264=CARTESIAN_POINT('Ctrl Pts',(-0.783641724003292,-0.0431439508480003,
-1.99339873088679));
#52265=CARTESIAN_POINT('Ctrl Pts',(-0.667778239355765,-0.412344486002345,
-1.97754122031085));
#52266=CARTESIAN_POINT('Ctrl Pts',(-0.389583785283206,-0.681307732480728,
-1.9616837097349));
#52267=CARTESIAN_POINT('Ctrl Pts',(-0.0166849670817576,-0.784651109708708,
-1.94582619915896));
#52268=CARTESIAN_POINT('Ctrl Pts',(0.360269818687344,-0.697252758930801,
-1.92996868858301));
#52269=CARTESIAN_POINT('Ctrl Pts',(0.649646205707602,-0.44035844434204,
-1.91411117800707));
#52270=CARTESIAN_POINT('Ctrl Pts',(0.781099359922979,-0.076416896178388,
-1.89825366743113));
#52271=CARTESIAN_POINT('Ctrl Pts',(0.722674185015349,0.306100921929396,
-1.88239615685518));
#52272=CARTESIAN_POINT('Ctrl Pts',(0.488573323003616,0.614208319825472,
-1.86653864627924));
#52273=CARTESIAN_POINT('Ctrl Pts',(0.1357046178904,0.773007120780168,-1.8506811357033));
#52274=CARTESIAN_POINT('Ctrl Pts',(-0.250152676666605,0.743894744201193,
-1.83482362512736));
#52275=CARTESIAN_POINT('Ctrl Pts',(-0.575200073394752,0.533948150722799,
-1.81896611455141));
#52276=CARTESIAN_POINT('Ctrl Pts',(-0.760421432039351,0.194203495820362,
-1.80310860397547));
#52277=CARTESIAN_POINT('Ctrl Pts',(-0.76079108249769,-0.192750307096041,
-1.78725109339952));
#52278=CARTESIAN_POINT('Ctrl Pts',(-0.576219166020697,-0.532848219293294,
-1.77139358282358));
#52279=CARTESIAN_POINT('Ctrl Pts',(-0.251573479078132,-0.743415453644965,
-1.75553607224764));
#52280=CARTESIAN_POINT('Ctrl Pts',(0.134227490162612,-0.773264982382023,
-1.73967856167169));
#52281=CARTESIAN_POINT('Ctrl Pts',(0.487398946613895,-0.615140649716218,
-1.72382105109575));
#52282=CARTESIAN_POINT('Ctrl Pts',(0.722088040451945,-0.307481078978686,
-1.70796354051981));
#52283=CARTESIAN_POINT('Ctrl Pts',(0.78124393373246,0.0749244159126821,
-1.69210602994387));
#52284=CARTESIAN_POINT('Ctrl Pts',(0.650486353278686,0.439116449580088,
-1.67624851936792));
#52285=CARTESIAN_POINT('Ctrl Pts',(0.361601307594298,0.696563167587635,
-1.66039100879198));
#52286=CARTESIAN_POINT('Ctrl Pts',(-0.0151858099871515,0.78468155532589,
-1.64453349821603));
#52287=CARTESIAN_POINT('Ctrl Pts',(-0.388281391799038,0.682050813998657,
-1.62867598764009));
#52288=CARTESIAN_POINT('Ctrl Pts',(-0.66698920979093,0.413619566892203,
-1.61281847706415));
#52289=CARTESIAN_POINT('Ctrl Pts',(-0.783557864449414,0.0446410702504095,
-1.5969609664882));
#52290=CARTESIAN_POINT('Ctrl Pts',(-0.70965054933176,-0.335189274778826,
-1.58110345591226));
#52291=CARTESIAN_POINT('Ctrl Pts',(-0.463233477476344,-0.633538078917755,
-1.56524594533632));
#52292=CARTESIAN_POINT('Ctrl Pts',(-0.104208454302516,-0.777879393058787,
-1.54938843476037));
#52293=CARTESIAN_POINT('Ctrl Pts',(0.280148720193781,-0.733125123473075,
-1.53353092418443));
#52294=CARTESIAN_POINT('Ctrl Pts',(0.596404224626504,-0.510154636302842,
-1.51767341360849));
#52295=CARTESIAN_POINT('Ctrl Pts',(0.767679149808526,-0.163170080109321,
-1.50181590303254));
#52296=CARTESIAN_POINT('Ctrl Pts',(0.752338079961976,0.223479675882952,
-1.4859583924566));
#52297=CARTESIAN_POINT('Ctrl Pts',(0.554110293151698,0.555803504052435,
-1.47010088188065));
#52298=CARTESIAN_POINT('Ctrl Pts',(0.221183206851683,0.753016428174334,
-1.45424337130472));
#52299=CARTESIAN_POINT('Ctrl Pts',(-0.165511556010258,0.767177734896347,
-1.43838586072877));
#52300=CARTESIAN_POINT('Ctrl Pts',(-0.511971927041593,0.594844936109356,
-1.42252835015283));
#52301=CARTESIAN_POINT('Ctrl Pts',(-0.733976461783252,0.277910607285441,
-1.40667083957688));
#52302=CARTESIAN_POINT('Ctrl Pts',(-0.777557826145205,-0.106581326197277,
-1.39081332900094));
#52303=CARTESIAN_POINT('Ctrl Pts',(-0.632121776846072,-0.465164284237934,
-1.37495581842499));
#52304=CARTESIAN_POINT('Ctrl Pts',(-0.33302252802565,-0.71066992895509,
-1.35909830784906));
#52305=CARTESIAN_POINT('Ctrl Pts',(0.0470315447598909,-0.783418014785927,
-1.34324079727311));
#52306=CARTESIAN_POINT('Ctrl Pts',(0.415652665998827,-0.665724127053912,
-1.32738328669717));
#52307=CARTESIAN_POINT('Ctrl Pts',(0.68323230933518,-0.386198606385552,
-1.31152577612122));
#52308=CARTESIAN_POINT('Ctrl Pts',(0.784724235851218,-0.0127916285651174,
-1.29566826554528));
#52309=CARTESIAN_POINT('Ctrl Pts',(0.695456658044464,0.363724880748143,
-1.27981075496933));
#52310=CARTESIAN_POINT('Ctrl Pts',(0.437129732627986,0.65182309635837,-1.26395324439339));
#52311=CARTESIAN_POINT('Ctrl Pts',(0.0725404448283483,0.781468896346956,
-1.24809573381745));
#52312=CARTESIAN_POINT('Ctrl Pts',(-0.309682781961072,0.721146536184204,
-1.23223822324151));
#52313=CARTESIAN_POINT('Ctrl Pts',(-0.616624870122073,0.485519846803979,
-1.21638071266556));
#52314=CARTESIAN_POINT('Ctrl Pts',(-0.77367091938988,0.131867587314102,
-1.20052320208962));
#52315=CARTESIAN_POINT('Ctrl Pts',(-0.742644427567277,-0.253840513505818,
-1.18466569151368));
#52316=CARTESIAN_POINT('Ctrl Pts',(-0.531087659733577,-0.577842236057851,
-1.16880818093773));
#52317=CARTESIAN_POINT('Ctrl Pts',(-0.190428190474026,-0.761375634208512,
-1.15295067036179));
#52318=CARTESIAN_POINT('Ctrl Pts',(0.19652268354188,-0.759825366085605,
-1.13709315978584));
#52319=CARTESIAN_POINT('Ctrl Pts',(0.535700635570782,-0.573568288125039,
-1.1212356492099));
#52320=CARTESIAN_POINT('Ctrl Pts',(0.744654512646728,-0.247881844612484,
-1.10537813863396));
#52321=CARTESIAN_POINT('Ctrl Pts',(0.772589479850304,0.138062477589907,
-1.08952062805802));
#52322=CARTESIAN_POINT('Ctrl Pts',(0.612714794327425,0.490445035560485,
-1.07366311748207));
#52323=CARTESIAN_POINT('Ctrl Pts',(0.303894574670057,0.723604753701724,
-1.05780560690613));
#52324=CARTESIAN_POINT('Ctrl Pts',(-0.0787997217418853,0.780862571741677,
-1.04194809633018));
#52325=CARTESIAN_POINT('Ctrl Pts',(-0.442338504441484,0.648299621766123,
-1.02609058575424));
#52326=CARTESIAN_POINT('Ctrl Pts',(-0.698348718511349,0.358140781602964,
-1.0102330751783));
#52327=CARTESIAN_POINT('Ctrl Pts',(-0.784596550713174,-0.0190789072699962,
-0.994375564602355));
#52328=CARTESIAN_POINT('Ctrl Pts',(-0.680115917717199,-0.391660682940369,
-0.978518054026408));
#52329=CARTESIAN_POINT('Ctrl Pts',(-0.410305135073127,-0.669033219075294,
-0.962660543450468));
#52330=CARTESIAN_POINT('Ctrl Pts',(-0.0407528118829727,-0.783769711342085,
-0.946803032874522));
#52331=CARTESIAN_POINT('Ctrl Pts',(0.338706158559024,-0.707978735731387,
-0.93094552229858));
#52332=CARTESIAN_POINT('Ctrl Pts',(0.635828664844656,-0.460084406446779,
-0.915088011722638));
#52333=CARTESIAN_POINT('Ctrl Pts',(0.778386860002041,-0.100347637091199,
-0.899230501146693));
#52334=CARTESIAN_POINT('Ctrl Pts',(0.731726110718017,0.283782753153026,
-0.883372990570751));
#52335=CARTESIAN_POINT('Ctrl Pts',(0.50718923144649,0.598928072140841,-0.867515479994805));
#52336=CARTESIAN_POINT('Ctrl Pts',(0.159359146780791,0.768479286923808,
-0.851657969418865));
#52337=CARTESIAN_POINT('Ctrl Pts',(-0.227209733579464,0.751220000439534,
-0.835800458842918));
#52338=CARTESIAN_POINT('Ctrl Pts',(-0.558545942161822,0.551345792210469,
-0.819942948266977));
#52339=CARTESIAN_POINT('Ctrl Pts',(-0.754104584306817,0.21744431016025,
-0.804085437691032));
#52340=CARTESIAN_POINT('Ctrl Pts',(-0.766347087943781,-0.169315955815492,
-0.78822792711509));
#52341=CARTESIAN_POINT('Ctrl Pts',(-0.592297408981341,-0.514917014098013,
-0.772370416539145));
#52342=CARTESIAN_POINT('Ctrl Pts',(-0.274265481240269,-0.735346311538768,
-0.756512905963204));
#52343=CARTESIAN_POINT('Ctrl Pts',(0.110437953335934,-0.777019440269414,
-0.740655395387258));
#52344=CARTESIAN_POINT('Ctrl Pts',(0.468294900605758,-0.629806032172024,
-0.724797884811316));
#52345=CARTESIAN_POINT('Ctrl Pts',(0.712313509469297,-0.329492361552069,
-0.708940374235371));
#52346=CARTESIAN_POINT('Ctrl Pts',(0.7831750195956,0.0509179808619445,-0.69308286365943));
#52347=CARTESIAN_POINT('Ctrl Pts',(0.663653626135406,0.418950613570325,
-0.677225353083484));
#52348=CARTESIAN_POINT('Ctrl Pts',(0.382803920154978,0.685140066561286,
-0.661367842507542));
#52349=CARTESIAN_POINT('Ctrl Pts',(0.00889797514763637,0.784778043864566,
-0.645510331931599));
#52350=CARTESIAN_POINT('Ctrl Pts',(-0.367170988728106,0.693643436594083,
-0.629652821355654));
#52351=CARTESIAN_POINT('Ctrl Pts',(-0.6539839406043,0.43389025977233,-0.613795310779713));
#52352=CARTESIAN_POINT('Ctrl Pts',(-0.781819194780839,0.0686622076972637,
-0.597937800203768));
#52353=CARTESIAN_POINT('Ctrl Pts',(-0.719601134362537,-0.313257018305708,
-0.582080289627826));
#52354=CARTESIAN_POINT('Ctrl Pts',(-0.482454418207954,-0.619026240514282,
-0.56622277905188));
#52355=CARTESIAN_POINT('Ctrl Pts',(-0.128027310457176,-0.774315671977985,
-0.55036526847594));
#52356=CARTESIAN_POINT('Ctrl Pts',(0.25752210136793,-0.741375828713559,
-0.534507757899993));
#52357=CARTESIAN_POINT('Ctrl Pts',(0.58047017355689,-0.528214094571827,
-0.518650247324052));
#52358=CARTESIAN_POINT('Ctrl Pts',(0.762311093038232,-0.18664819721801,
-0.502792736748107));
#52359=CARTESIAN_POINT('Ctrl Pts',(0.758840944497711,0.200290222045565,
-0.486935226172165));
#52360=CARTESIAN_POINT('Ctrl Pts',(0.570903290280831,0.538539864114544,
-0.471077715596219));
#52361=CARTESIAN_POINT('Ctrl Pts',(0.244184107857459,0.745875239945465,
-0.455220205020278));
#52362=CARTESIAN_POINT('Ctrl Pts',(-0.14189406623027,0.771894957918566,
-0.439362694444333));
#52363=CARTESIAN_POINT('Ctrl Pts',(-0.493479050867978,0.61027385529337,
-0.42350518386839));
#52364=CARTESIAN_POINT('Ctrl Pts',(-0.725103653436951,0.300300589163106,
-0.407647673292446));
#52365=CARTESIAN_POINT('Ctrl Pts',(-0.780461986703319,-0.0826730876933915,
-0.391790162716504));
#52366=CARTESIAN_POINT('Ctrl Pts',(-0.646096930557075,-0.445549669947661,
-0.375932652140559));
#52367=CARTESIAN_POINT('Ctrl Pts',(-0.354671439060398,-0.700117077646639,
-0.360075141564617));
#52368=CARTESIAN_POINT('Ctrl Pts',(0.0229715349940275,-0.784492231170089,
-0.344217630988674));
#52369=CARTESIAN_POINT('Ctrl Pts',(0.395030332049294,-0.678164278417535,
-0.32836012041273));
#52370=CARTESIAN_POINT('Ctrl Pts',(0.67106075874077,-0.406980602684816,
-0.312502609836786));
#52371=CARTESIAN_POINT('Ctrl Pts',(0.783962262705086,-0.0368635498603739,
-0.296645099260844));
#52372=CARTESIAN_POINT('Ctrl Pts',(0.706289495057392,0.342214703354879,
-0.280787588684899));
#52373=CARTESIAN_POINT('Ctrl Pts',(0.456924005754423,0.638103599690982,
-0.264930078108956));
#52374=CARTESIAN_POINT('Ctrl Pts',(0.0964843562473045,0.778875161746238,
-0.249072567533014));
#52375=CARTESIAN_POINT('Ctrl Pts',(-0.287409813109609,0.730309090546973,
-0.233215056957069));
#52376=CARTESIAN_POINT('Ctrl Pts',(-0.601437149847266,0.504211328984171,
-0.217357546381126));
#52377=CARTESIAN_POINT('Ctrl Pts',(-0.769260555748459,0.155544313360371,
-0.201500035805183));
#52378=CARTESIAN_POINT('Ctrl Pts',(-0.750083330065511,-0.230934242753795,
-0.185642525229239));
#52379=CARTESIAN_POINT('Ctrl Pts',(-0.548567908879648,-0.561274542499788,
-0.169785014653295));
#52380=CARTESIAN_POINT('Ctrl Pts',(-0.213699688385254,-0.755174347285152,
-0.153927504077352));
#52381=CARTESIAN_POINT('Ctrl Pts',(0.173115460605444,-0.765497240872467,
-0.138069993501409));
#52382=CARTESIAN_POINT('Ctrl Pts',(0.51785084486316,-0.589735954039219,
-0.122212482925465));
#52383=CARTESIAN_POINT('Ctrl Pts',(0.73669528515483,-0.270612327298038,
-0.106354972349523));
#52384=CARTESIAN_POINT('Ctrl Pts',(0.776467346061449,0.114289367285656,
-0.0904974617735793));
#52385=CARTESIAN_POINT('Ctrl Pts',(0.627464170859799,0.471418880043696,
-0.0746399511976351));
#52386=CARTESIAN_POINT('Ctrl Pts',(0.325975076844769,0.713929799385627,
-0.0587824406216925));
#52387=CARTESIAN_POINT('Ctrl Pts',(-0.0548469677254658,0.782933924134,-0.0429249300457488));
#52388=CARTESIAN_POINT('Ctrl Pts',(-0.29969712480825,0.701979163404131,
-0.0323532563284528));
#52389=CARTESIAN_POINT('Ctrl Pts',(-0.405096567646226,0.634709045147742,
-0.027067419469805));
#52390=CARTESIAN_POINT('Ctrl Pts',(-0.342067962509741,0.71332231075751,
-5.8089));
#52391=CARTESIAN_POINT('Ctrl Pts',(-0.460521881974901,0.656518688787926,
-5.80361416314135));
#52392=CARTESIAN_POINT('Ctrl Pts',(-0.668467913999907,0.482822123354284,
-5.79304248942406));
#52393=CARTESIAN_POINT('Ctrl Pts',(-0.81790697907055,0.104654431008339,
-5.77718497884811));
#52394=CARTESIAN_POINT('Ctrl Pts',(-0.76850808527292,-0.298848385144198,
-5.76132746827218));
#52395=CARTESIAN_POINT('Ctrl Pts',(-0.53229805344993,-0.629755578447219,
-5.74546995769623));
#52396=CARTESIAN_POINT('Ctrl Pts',(-0.166687806613194,-0.807548479192264,
-5.72961244712028));
#52397=CARTESIAN_POINT('Ctrl Pts',(0.239441088352843,-0.789046946221705,
-5.71375493654434));
#52398=CARTESIAN_POINT('Ctrl Pts',(0.587364837768938,-0.578728216806966,
-5.6978974259684));
#52399=CARTESIAN_POINT('Ctrl Pts',(0.792504962384066,-0.2277293106754,-5.68203991539245));
#52400=CARTESIAN_POINT('Ctrl Pts',(0.80499438247605,0.178630374729474,-5.66618240481651));
#52401=CARTESIAN_POINT('Ctrl Pts',(0.621796689907431,0.541565676804147,
-5.65032489424056));
#52402=CARTESIAN_POINT('Ctrl Pts',(0.287445793992361,0.772851636913208,
-5.63446738366463));
#52403=CARTESIAN_POINT('Ctrl Pts',(-0.116780656177354,0.816263974340416,
-5.61860987308867));
#52404=CARTESIAN_POINT('Ctrl Pts',(-0.492618748730099,0.661249900488588,
-5.60275236251274));
#52405=CARTESIAN_POINT('Ctrl Pts',(-0.748705598981454,0.345491775112376,
-5.58689485193679));
#52406=CARTESIAN_POINT('Ctrl Pts',(-0.822788752131379,-0.0542523051869823,
-5.57103734136086));
#52407=CARTESIAN_POINT('Ctrl Pts',(-0.696859256610704,-0.440808147714975,
-5.5551798307849));
#52408=CARTESIAN_POINT('Ctrl Pts',(-0.401529453140775,-0.720207429259136,
-5.53932232020897));
#52409=CARTESIAN_POINT('Ctrl Pts',(-0.00859140014129245,-0.824530674507732,
-5.52346480963302));
#52410=CARTESIAN_POINT('Ctrl Pts',(0.386435146339414,-0.728417820893135,
-5.50760729905707));
#52411=CARTESIAN_POINT('Ctrl Pts',(0.687522734759737,-0.455233054357242,
-5.49174978848114));
#52412=CARTESIAN_POINT('Ctrl Pts',(0.821479642051262,-0.0713851678466922,
-5.47589227790518));
#52413=CARTESIAN_POINT('Ctrl Pts',(0.755742131611029,0.329815819763054,
-5.46003476732925));
#52414=CARTESIAN_POINT('Ctrl Pts',(0.506290409450845,0.650841505908578,
-5.4441772567533));
#52415=CARTESIAN_POINT('Ctrl Pts',(0.133763977544822,0.813653392289577,
-5.42831974617736));
#52416=CARTESIAN_POINT('Ctrl Pts',(-0.271279291337799,0.778673352945406,
-5.41246223560142));
#52417=CARTESIAN_POINT('Ctrl Pts',(-0.61037696967741,0.55440472524481,-5.39660472502547));
#52418=CARTESIAN_POINT('Ctrl Pts',(-0.801097418326339,0.195365224233614,
-5.38074721444952));
#52419=CARTESIAN_POINT('Ctrl Pts',(-0.797078187159076,-0.211165830674235,
-5.36488970387359));
#52420=CARTESIAN_POINT('Ctrl Pts',(-0.599296315636618,-0.566364344351477,
-5.34903219329764));
#52421=CARTESIAN_POINT('Ctrl Pts',(-0.255830823180538,-0.783884707338891,
-5.3331746827217));
#52422=CARTESIAN_POINT('Ctrl Pts',(0.149824874179238,-0.810849647940832,
-5.31731717214575));
#52423=CARTESIAN_POINT('Ctrl Pts',(0.519059472982411,-0.64070422817085,
-5.30145966156981));
#52424=CARTESIAN_POINT('Ctrl Pts',(0.762115315916334,-0.31480929105487,
-5.28560215099387));
#52425=CARTESIAN_POINT('Ctrl Pts',(0.819907682511568,0.0876129935981942,
-5.26974464041792));
#52426=CARTESIAN_POINT('Ctrl Pts',(0.678387760839459,0.468737336289701,
-5.25388712984198));
#52427=CARTESIAN_POINT('Ctrl Pts',(0.371957789134283,0.73591578838279,-5.23802961926604));
#52428=CARTESIAN_POINT('Ctrl Pts',(-0.0248918233091328,0.824199636994026,
-5.22217210869009));
#52429=CARTESIAN_POINT('Ctrl Pts',(-0.415690454198512,0.712127861255944,
-5.20631459811415));
#52430=CARTESIAN_POINT('Ctrl Pts',(-0.705438421208997,0.426944116215333,
-5.19045708753821));
#52431=CARTESIAN_POINT('Ctrl Pts',(-0.823700562483377,0.0379740418351834,
-5.17459957696226));
#52432=CARTESIAN_POINT('Ctrl Pts',(-0.741728399997165,-0.360227185434942,
-5.15874206638631));
#52433=CARTESIAN_POINT('Ctrl Pts',(-0.479448639680594,-0.670860377721891,
-5.14288455581038));
#52434=CARTESIAN_POINT('Ctrl Pts',(-0.100619165878374,-0.818413360073425,
-5.12702704523443));
#52435=CARTESIAN_POINT('Ctrl Pts',(0.302669935053257,-0.767017310693566,
-5.11116953465849));
#52436=CARTESIAN_POINT('Ctrl Pts',(0.632382658263431,-0.52916615350607,
-5.09531202408254));
#52437=CARTESIAN_POINT('Ctrl Pts',(0.808368763992744,-0.162679396020442,
-5.0794545135066));
#52438=CARTESIAN_POINT('Ctrl Pts',(0.787847590241883,0.243353280312371,
-5.06359700293066));
#52439=CARTESIAN_POINT('Ctrl Pts',(0.575807652407709,0.590228931786179,
-5.04773949235471));
#52440=CARTESIAN_POINT('Ctrl Pts',(0.22379397941877,0.793625162948256,-5.03188198177878));
#52441=CARTESIAN_POINT('Ctrl Pts',(-0.182622025795887,0.804098153326407,
-5.01602447120283));
#52442=CARTESIAN_POINT('Ctrl Pts',(-0.544644235677511,0.619102011813879,
-5.00016696062689));
#52443=CARTESIAN_POINT('Ctrl Pts',(-0.77426826071474,0.283607660225359,
-4.98430945005094));
#52444=CARTESIAN_POINT('Ctrl Pts',(-0.815674536281549,-0.120829199081238,
-4.968451939475));
#52445=CARTESIAN_POINT('Ctrl Pts',(-0.658797563898192,-0.49589355137019,
-4.95259442889906));
#52446=CARTESIAN_POINT('Ctrl Pts',(-0.341772744670322,-0.750410577943334,
-4.93673691832311));
#52447=CARTESIAN_POINT('Ctrl Pts',(0.0583339986090347,-0.822509446204123,
-4.92087940774717));
#52448=CARTESIAN_POINT('Ctrl Pts',(0.444260264019303,-0.694663560511296,
-4.90502189717122));
#52449=CARTESIAN_POINT('Ctrl Pts',(0.722190798084908,-0.397951122187407,
-4.88916438659529));
#52450=CARTESIAN_POINT('Ctrl Pts',(0.824563152123462,-0.00450029431852763,
-4.87330687601934));
#52451=CARTESIAN_POINT('Ctrl Pts',(0.726491514507689,0.390044515199301,
-4.85744936544339));
#52452=CARTESIAN_POINT('Ctrl Pts',(0.451816230832899,0.689772961230496,
-4.84159185486746));
#52453=CARTESIAN_POINT('Ctrl Pts',(0.0673084272727246,0.821823715955436,
-4.8257343442915));
#52454=CARTESIAN_POINT('Ctrl Pts',(-0.333561458196853,0.754096411670499,
-4.80987683371557));
#52455=CARTESIAN_POINT('Ctrl Pts',(-0.653345510554885,0.503054955572955,
-4.79401932313961));
#52456=CARTESIAN_POINT('Ctrl Pts',(-0.814307061897926,0.129725299891355,
-4.77816181256369));
#52457=CARTESIAN_POINT('Ctrl Pts',(-0.777317786189346,-0.275139426041463,
-4.76230430198772));
#52458=CARTESIAN_POINT('Ctrl Pts',(-0.551369448404747,-0.613120196906429,
-4.7464467914118));
#52459=CARTESIAN_POINT('Ctrl Pts',(-0.191388086187902,-0.802056883864271,
-4.73058928083584));
#52460=CARTESIAN_POINT('Ctrl Pts',(0.215118022922846,-0.796020653439657,
-4.71473177025991));
#52461=CARTESIAN_POINT('Ctrl Pts',(0.569330847910481,-0.596478859731226,
-4.69887425968396));
#52462=CARTESIAN_POINT('Ctrl Pts',(0.785144391492888,-0.251938343639862,
-4.68301674910802));
#52463=CARTESIAN_POINT('Ctrl Pts',(0.810096294641137,0.153846150089727,
-4.66715923853207));
#52464=CARTESIAN_POINT('Ctrl Pts',(0.638120970924981,0.522232008741798,
-4.65130172795613));
#52465=CARTESIAN_POINT('Ctrl Pts',(0.311024096796169,0.763667896209378,
-4.63544421738018));
#52466=CARTESIAN_POINT('Ctrl Pts',(-0.0916799777052979,0.819462888834321,
-4.61958670680424));
#52467=CARTESIAN_POINT('Ctrl Pts',(-0.472097462466847,0.676053718591279,
-4.6037291962283));
#52468=CARTESIAN_POINT('Ctrl Pts',(-0.737752239747422,0.368301883291948,
-4.58787168565236));
#52469=CARTESIAN_POINT('Ctrl Pts',(-0.824065988501475,-0.0289808744488347,
-4.57201417507641));
#52470=CARTESIAN_POINT('Ctrl Pts',(-0.710056601669826,-0.419218638557295,
-4.55615666450047));
#52471=CARTESIAN_POINT('Ctrl Pts',(-0.423438750377111,-0.707548068450336,
-4.54029915392452));
#52472=CARTESIAN_POINT('Ctrl Pts',(-0.0338866931013497,-0.823878836067166,
-4.52444164334859));
#52473=CARTESIAN_POINT('Ctrl Pts',(0.363902918825875,-0.739931963195765,
-4.50858413277264));
#52474=CARTESIAN_POINT('Ctrl Pts',(0.673230957571867,-0.476114190353113,
-4.4927266221967));
#52475=CARTESIAN_POINT('Ctrl Pts',(0.818902519438615,-0.0965572790928855,
-4.47686911162076));
#52476=CARTESIAN_POINT('Ctrl Pts',(0.765506139269209,0.306471850632131,
-4.46101160104481));
#52477=CARTESIAN_POINT('Ctrl Pts',(0.526022003667289,0.635000390666482,
-4.44515409046887));
#52478=CARTESIAN_POINT('Ctrl Pts',(0.158666582716821,0.809165965681761,
-4.42929657989292));
#52479=CARTESIAN_POINT('Ctrl Pts',(-0.247259277744567,0.786630468554307,
-4.41343906931699));
#52480=CARTESIAN_POINT('Ctrl Pts',(-0.593078600001993,0.572872078834715,
-4.39758155874103));
#52481=CARTESIAN_POINT('Ctrl Pts',(-0.794725772869754,0.21985356586898,
-4.38172404816509));
#52482=CARTESIAN_POINT('Ctrl Pts',(-0.80318215643975,-0.186609399724462,
-4.36586653758915));
#52483=CARTESIAN_POINT('Ctrl Pts',(-0.616392078840929,-0.547709274735137,
-4.3500090270132));
#52484=CARTESIAN_POINT('Ctrl Pts',(-0.279762551845409,-0.775665881081332,
-4.33415151643726));
#52485=CARTESIAN_POINT('Ctrl Pts',(0.124874771111987,-0.815064988837368,
-4.31829400586132));
#52486=CARTESIAN_POINT('Ctrl Pts',(0.499156144359348,-0.65632902422264,
-4.30243649528538));
#52487=CARTESIAN_POINT('Ctrl Pts',(0.752097084461584,-0.338045292872298,
-4.28657898470943));
#52488=CARTESIAN_POINT('Ctrl Pts',(0.822209891469548,0.062414252045241,
-4.27072147413349));
#52489=CARTESIAN_POINT('Ctrl Pts',(0.692450763624001,0.447701445659124,
-4.25486396355754));
#52490=CARTESIAN_POINT('Ctrl Pts',(0.394362994451903,0.72415638718143,-4.23900645298161));
#52491=CARTESIAN_POINT('Ctrl Pts',(0.000409077774761542,0.824575331394352,
-4.22314894240565));
#52492=CARTESIAN_POINT('Ctrl Pts',(-0.39364428208252,0.724547323280179,
-4.20729143182972));
#52493=CARTESIAN_POINT('Ctrl Pts',(-0.692006207039603,0.448388284757077,
-4.19143392125377));
#52494=CARTESIAN_POINT('Ctrl Pts',(-0.822147558434337,0.0632300296472444,
-4.17557641067783));
#52495=CARTESIAN_POINT('Ctrl Pts',(-0.75243212758377,-0.33729888506856,
-4.15971890010188));
#52496=CARTESIAN_POINT('Ctrl Pts',(-0.499807117626442,-0.655833431336555,
-4.14386138952594));
#52497=CARTESIAN_POINT('Ctrl Pts',(-0.125683428694324,-0.814940685105593,
-4.12800387895));
#52498=CARTESIAN_POINT('Ctrl Pts',(0.278992787436487,-0.775943083638968,
-4.11214636837406));
#52499=CARTESIAN_POINT('Ctrl Pts',(0.61584833050845,-0.548320598098126,
-4.09628885779811));
#52500=CARTESIAN_POINT('Ctrl Pts',(0.802996604582439,-0.187406236603287,
-4.08043134722217));
#52501=CARTESIAN_POINT('Ctrl Pts',(0.794943523499005,0.219064919454756,
-4.06457383664622));
#52502=CARTESIAN_POINT('Ctrl Pts',(0.593646719870428,0.572283335836205,
-4.04871632607028));
#52503=CARTESIAN_POINT('Ctrl Pts',(0.24803966194915,0.786384747174615,-4.03285881549433));
#52504=CARTESIAN_POINT('Ctrl Pts',(-0.157863638657288,0.809322998609712,
-4.01700130491839));
#52505=CARTESIAN_POINT('Ctrl Pts',(-0.525391688334729,0.635522004589546,
-4.00114379434245));
#52506=CARTESIAN_POINT('Ctrl Pts',(-0.765201676732551,0.307231245830278,
-3.98528628376651));
#52507=CARTESIAN_POINT('Ctrl Pts',(-0.818997921841139,-0.0957447048594847,
-3.96942877319056));
#52508=CARTESIAN_POINT('Ctrl Pts',(-0.673703033435362,-0.475445966676259,
-3.95357126261462));
#52509=CARTESIAN_POINT('Ctrl Pts',(-0.364636910693384,-0.739570529326795,
-3.93771375203868));
#52510=CARTESIAN_POINT('Ctrl Pts',(0.0330692121452029,-0.823912053375134,
-3.92185624146273));
#52511=CARTESIAN_POINT('Ctrl Pts',(0.42273650270493,-0.707967862102183,
-3.90599873088679));
#52512=CARTESIAN_POINT('Ctrl Pts',(0.709640297464547,-0.419922960438174,
-3.89014122031084));
#52513=CARTESIAN_POINT('Ctrl Pts',(0.824036827624427,-0.029798510154067,
-3.8742837097349));
#52514=CARTESIAN_POINT('Ctrl Pts',(0.738117310949273,0.367569693753101,
-3.85842619915896));
#52515=CARTESIAN_POINT('Ctrl Pts',(0.472768020175167,0.675584964004073,
-3.84256868858302));
#52516=CARTESIAN_POINT('Ctrl Pts',(0.0924930152864017,0.819371519282897,
-3.82671117800707));
#52517=CARTESIAN_POINT('Ctrl Pts',(-0.310266221569808,0.763976122821601,
-3.81085366743113));
#52518=CARTESIAN_POINT('Ctrl Pts',(-0.637602490801524,0.522864904360988,
-3.79499615685519));
#52519=CARTESIAN_POINT('Ctrl Pts',(-0.809943247541721,0.154649863402152,
-3.77913864627924));
#52520=CARTESIAN_POINT('Ctrl Pts',(-0.78539398181045,-0.251159188214685,
-3.7632811357033));
#52521=CARTESIAN_POINT('Ctrl Pts',(-0.569922402451707,-0.595913667969116,
-3.74742362512736));
#52522=CARTESIAN_POINT('Ctrl Pts',(-0.21590774002352,-0.795806818446958,
-3.73156611455141));
#52523=CARTESIAN_POINT('Ctrl Pts',(0.190592179753276,-0.802246387031831,
-3.71570860397547));
#52524=CARTESIAN_POINT('Ctrl Pts',(0.550760830433868,-0.613666971694362,
-3.69985109339953));
#52525=CARTESIAN_POINT('Ctrl Pts',(0.777044406314893,-0.275910556346559,
-3.68399358282358));
#52526=CARTESIAN_POINT('Ctrl Pts',(0.814435376343574,0.128917269009375,
-3.66813607224764));
#52527=CARTESIAN_POINT('Ctrl Pts',(0.653844327216543,0.502406449257448,
-3.65227856167169));
#52528=CARTESIAN_POINT('Ctrl Pts',(0.334309519166617,0.753765076057067,
-3.63642105109575));
#52529=CARTESIAN_POINT('Ctrl Pts',(-0.0664929689842511,0.821890095794073,
-3.6205635405198));
#52530=CARTESIAN_POINT('Ctrl Pts',(-0.451131605905745,0.690220920170952,
-3.60470602994387));
#52531=CARTESIAN_POINT('Ctrl Pts',(-0.72610414919172,0.390765158394787,
-3.58884851936792));
#52532=CARTESIAN_POINT('Ctrl Pts',(-0.824567211492583,-0.00368214883957207,
-3.57299100879198));
#52533=CARTESIAN_POINT('Ctrl Pts',(-0.72258529534248,-0.397234358337186,
-3.55713349821603));
#52534=CARTESIAN_POINT('Ctrl Pts',(-0.444949300379643,-0.694222417226928,
-3.54127598764009));
#52535=CARTESIAN_POINT('Ctrl Pts',(-0.059150075441984,-0.822451161506835,
-3.52541847706415));
#52536=CARTESIAN_POINT('Ctrl Pts',(0.341028008407468,-0.750749320326278,
-3.50956096648821));
#52537=CARTESIAN_POINT('Ctrl Pts',(0.658305206988058,-0.496546975563384,
-3.49370345591226));
#52538=CARTESIAN_POINT('Ctrl Pts',(0.815554246323718,-0.121638463456612,
-3.47784594533632));
#52539=CARTESIAN_POINT('Ctrl Pts',(0.774549279131463,0.282839280662471,
-3.46198843476038));
#52540=CARTESIAN_POINT('Ctrl Pts',(0.545258249383206,0.618561303322714,
-3.44613092418443));
#52541=CARTESIAN_POINT('Ctrl Pts',(0.183419773502581,0.803916557347213,
-3.43027341360849));
#52542=CARTESIAN_POINT('Ctrl Pts',(-0.223006423105693,0.793846823853531,
-3.41441590303254));
#52543=CARTESIAN_POINT('Ctrl Pts',(-0.575221735445436,0.590799965775112,
-3.3985583924566));
#52544=CARTESIAN_POINT('Ctrl Pts',(-0.787605743849167,0.244134874085071,
-3.38270088188066));
#52545=CARTESIAN_POINT('Ctrl Pts',(-0.808529778883429,-0.161877240980456,
-3.36684337130471));
#52546=CARTESIAN_POINT('Ctrl Pts',(-0.632907393145164,-0.528538433977061,
-3.35098586072877));
#52547=CARTESIAN_POINT('Ctrl Pts',(-0.303430831528625,-0.76671661972764,
-3.33512835015283));
#52548=CARTESIAN_POINT('Ctrl Pts',(0.0998070749963794,-0.818512792978461,
-3.31927083957688));
#52549=CARTESIAN_POINT('Ctrl Pts',(0.478782766485345,-0.671335763240253,
-3.30341332900094));
#52550=CARTESIAN_POINT('Ctrl Pts',(0.741370612358751,-0.360962961561908,
-3.287555818425));
#52551=CARTESIAN_POINT('Ctrl Pts',(0.82373783540453,0.0371567357526397,
-3.27169830784905));
#52552=CARTESIAN_POINT('Ctrl Pts',(0.705861693973048,0.426243960039592,
-3.25584079727311));
#52553=CARTESIAN_POINT('Ctrl Pts',(0.416396832949279,0.711715056745706,
-3.23998328669717));
#52554=CARTESIAN_POINT('Ctrl Pts',(0.0257095936351012,0.82417453326577,
-3.22412577612122));
#52555=CARTESIAN_POINT('Ctrl Pts',(-0.371227419948954,0.736284487930295,
-3.20826826554528));
#52556=CARTESIAN_POINT('Ctrl Pts',(-0.677922339068225,0.469410211521862,
-3.19241075496933));
#52557=CARTESIAN_POINT('Ctrl Pts',(-0.81982034806056,0.0884264745118526,
-3.1765532443934));
#52558=CARTESIAN_POINT('Ctrl Pts',(-0.76242729901627,-0.314052954457505,
-3.16069573381745));
#52559=CARTESIAN_POINT('Ctrl Pts',(-0.519694933307771,-0.640188894610773,
-3.14483822324151));
#52560=CARTESIAN_POINT('Ctrl Pts',(-0.150629336958933,-0.810700590437707,
-3.12898071266556));
#52561=CARTESIAN_POINT('Ctrl Pts',(0.255052915715792,-0.784138160449806,
-3.11312320208962));
#52562=CARTESIAN_POINT('Ctrl Pts',(0.598734065894616,-0.566958695873019,
-3.09726569151368));
#52563=CARTESIAN_POINT('Ctrl Pts',(0.796868273066979,-0.211956599019665,
-3.08140818093773));
#52564=CARTESIAN_POINT('Ctrl Pts',(0.80129086813917,0.194570267835308,-3.06555067036179));
#52565=CARTESIAN_POINT('Ctrl Pts',(0.610926757460146,0.553798827651308,
-3.04969315978584));
#52566=CARTESIAN_POINT('Ctrl Pts',(0.272051768556222,0.778403802479257,
-3.0338356492099));
#52567=CARTESIAN_POINT('Ctrl Pts',(-0.132956593256252,0.813785714299792,
-3.01797813863396));
#52568=CARTESIAN_POINT('Ctrl Pts',(-0.505644386049347,0.65134353404752,
-3.00212062805802));
#52569=CARTESIAN_POINT('Ctrl Pts',(-0.755414511667619,0.330565515519547,
-2.98626311748207));
#52570=CARTESIAN_POINT('Ctrl Pts',(-0.821550067050345,-0.0705700490173305,
-2.97040560690613));
#52571=CARTESIAN_POINT('Ctrl Pts',(-0.68797408504582,-0.454550660316427,
-2.95454809633018));
#52572=CARTESIAN_POINT('Ctrl Pts',(-0.387157702586595,-0.728034036166306,
-2.93869058575424));
#52573=CARTESIAN_POINT('Ctrl Pts',(0.00777328480777176,-0.824538792618049,
-2.9228330751783));
#52574=CARTESIAN_POINT('Ctrl Pts',(0.400814655583785,-0.720605478995258,
-2.90697556460235));
#52575=CARTESIAN_POINT('Ctrl Pts',(0.69642153723441,-0.441499362360574,
-2.89111805402641));
#52576=CARTESIAN_POINT('Ctrl Pts',(0.822734517698912,-0.0550686650961424,
-2.87526054345047));
#52577=CARTESIAN_POINT('Ctrl Pts',(0.749048031324911,0.344748736411039,
-2.85940303287452));
#52578=CARTESIAN_POINT('Ctrl Pts',(0.493274609641072,0.660760776659891,
-2.84354552229858));
#52579=CARTESIAN_POINT('Ctrl Pts',(0.117590503756079,0.816147730447817,
-2.82768801172263));
#52580=CARTESIAN_POINT('Ctrl Pts',(-0.286678811027477,0.773136406979133,
-2.8118305011467));
#52581=CARTESIAN_POINT('Ctrl Pts',(-0.621259048561971,0.542182477648074,
-2.79597299057075));
#52582=CARTESIAN_POINT('Ctrl Pts',(-0.80481671951144,0.179428795023482,
-2.78011547999481));
#52583=CARTESIAN_POINT('Ctrl Pts',(-0.792730581501495,-0.226942436844752,
-2.76425796941886));
#52584=CARTESIAN_POINT('Ctrl Pts',(-0.587938667525923,-0.578145974401426,
-2.74840045884292));
#52585=CARTESIAN_POINT('Ctrl Pts',(-0.240224076174663,-0.788807351458366,
-2.73254294826698));
#52586=CARTESIAN_POINT('Ctrl Pts',(0.165886858253439,-0.807716654989569,
-2.71668543769103));
#52587=CARTESIAN_POINT('Ctrl Pts',(0.531672168203069,-0.630277200957627,
-2.70082792711509));
#52588=CARTESIAN_POINT('Ctrl Pts',(0.768212687900203,-0.299622947448753,
-2.68497041653915));
#52589=CARTESIAN_POINT('Ctrl Pts',(0.818007514189052,0.103866988109699,
-2.6691129059632));
#52590=CARTESIAN_POINT('Ctrl Pts',(0.668951966282746,0.482107779749695,
-2.65325539538726));
#52591=CARTESIAN_POINT('Ctrl Pts',(0.357280126341784,0.743152444529339,
-2.63739788481132));
#52592=CARTESIAN_POINT('Ctrl Pts',(-0.0412433446456093,0.823543338878517,
-2.62154037423537));
#52593=CARTESIAN_POINT('Ctrl Pts',(-0.429740924215648,0.703738149131488,
-2.60568286365943));
#52594=CARTESIAN_POINT('Ctrl Pts',(-0.713772295217946,0.412860454715681,
-2.58982535308349));
#52595=CARTESIAN_POINT('Ctrl Pts',(-0.824291949601193,0.0216200442043072,
-2.57396784250754));
#52596=CARTESIAN_POINT('Ctrl Pts',(-0.73443353925878,-0.374876007368511,
-2.5581103319316));
#52597=CARTESIAN_POINT('Ctrl Pts',(-0.466040847054833,-0.680243025223445,
-2.54225282135565));
#52598=CARTESIAN_POINT('Ctrl Pts',(-0.0843577568782632,-0.820248994722455,
-2.52639531077971));
#52599=CARTESIAN_POINT('Ctrl Pts',(0.317831956074426,-0.76085970598175,
-2.51053780020377));
#52600=CARTESIAN_POINT('Ctrl Pts',(0.642759538422818,-0.516512168545157,
-2.49468028962782));
#52601=CARTESIAN_POINT('Ctrl Pts',(0.811437975725651,-0.146605102363427,
-2.47882277905189));
#52602=CARTESIAN_POINT('Ctrl Pts',(0.782863035387856,0.258940364393128,
-2.46296526847593));
#52603=CARTESIAN_POINT('Ctrl Pts',(0.563981032058397,0.601539724346679,
-2.4471077579));
#52604=CARTESIAN_POINT('Ctrl Pts',(0.208000240125556,0.797910110599211,
-2.43125024732405));
#52605=CARTESIAN_POINT('Ctrl Pts',(-0.198543566039071,0.800315623284477,
-2.41539273674811));
#52606=CARTESIAN_POINT('Ctrl Pts',(-0.556823191598891,0.608171503596115,
-2.39953522617216));
#52607=CARTESIAN_POINT('Ctrl Pts',(-0.779744036109187,0.268186283468949,
-2.38367771559622));
#52608=CARTESIAN_POINT('Ctrl Pts',(-0.813116018699228,-0.136992644413672,
-2.36782020502028));
#52609=CARTESIAN_POINT('Ctrl Pts',(-0.648826706279392,-0.508869875024419,
-2.35196269444433));
#52610=CARTESIAN_POINT('Ctrl Pts',(-0.326813374099942,-0.757045350687886,
-2.33610518386839));
#52611=CARTESIAN_POINT('Ctrl Pts',(0.0746453917760193,-0.821189813609094,
-2.32024767329245));
#52612=CARTESIAN_POINT('Ctrl Pts',(0.457958524721799,-0.685710313560593,
-2.3043901627165));
#52613=CARTESIAN_POINT('Ctrl Pts',(0.729946000595748,-0.383540715834715,
-2.28853265214056));
#52614=CARTESIAN_POINT('Ctrl Pts',(0.824490075470356,0.0118642294153475,
-2.27267514156462));
#52615=CARTESIAN_POINT('Ctrl Pts',(0.718607922977105,0.404385085683513,
-2.25681763098867));
#52616=CARTESIAN_POINT('Ctrl Pts',(0.43803855562953,0.698603512924695,-2.24096012041273));
#52617=CARTESIAN_POINT('Ctrl Pts',(0.0509858990848059,0.822997620034983,
-2.22510260983679));
#52618=CARTESIAN_POINT('Ctrl Pts',(-0.348460977483367,0.747328302461555,
-2.20924509926084));
#52619=CARTESIAN_POINT('Ctrl Pts',(-0.663200079901485,0.48999010041775,
-2.1933875886849));
#52620=CARTESIAN_POINT('Ctrl Pts',(-0.816721122867659,0.11353964924432,
-2.17753007810895));
#52621=CARTESIAN_POINT('Ctrl Pts',(-0.771704501963684,-0.290511284010991,
-2.16167256753301));
#52622=CARTESIAN_POINT('Ctrl Pts',(-0.539093358611228,-0.623941499813884,
-2.14581505695707));
#52623=CARTESIAN_POINT('Ctrl Pts',(-0.175433399414776,-0.805697068915178,
-2.12995754638113));
#52624=CARTESIAN_POINT('Ctrl Pts',(0.230872863776256,-0.791594823922241,
-2.11410003580518));
#52625=CARTESIAN_POINT('Ctrl Pts',(0.581055980716084,-0.585062895561496,
-2.09824252522924));
#52626=CARTESIAN_POINT('Ctrl Pts',(0.789989540421377,-0.236307364492848,
-2.08238501465329));
#52627=CARTESIAN_POINT('Ctrl Pts',(0.806883646945381,0.169892391768596,
-2.06652750407735));
#52628=CARTESIAN_POINT('Ctrl Pts',(0.627631492776286,0.534792813867337,
-2.05066999350141));
#52629=CARTESIAN_POINT('Ctrl Pts',(0.295807687332132,0.769689844420431,
-2.03481248292547));
#52630=CARTESIAN_POINT('Ctrl Pts',(-0.107924344253576,0.817482097911734,
-2.01895497234952));
#52631=CARTESIAN_POINT('Ctrl Pts',(-0.485420924615018,0.666551701246522,
-2.00309746177358));
#52632=CARTESIAN_POINT('Ctrl Pts',(-0.74491598197389,0.353588495696068,
-1.98723995119764));
#52633=CARTESIAN_POINT('Ctrl Pts',(-0.823328568585157,-0.0453289382210672,
-1.97138244062169));
#52634=CARTESIAN_POINT('Ctrl Pts',(-0.701597279854368,-0.433227309145766,
-1.95552493004575));
#52635=CARTESIAN_POINT('Ctrl Pts',(-0.409313912795,-0.715811962236716,-1.93966741946981));
#52636=CARTESIAN_POINT('Ctrl Pts',(-0.0175299625371316,-0.824389073740172,
-1.92380990889386));
#52637=CARTESIAN_POINT('Ctrl Pts',(0.378515366191811,-0.732564510500893,
-1.90795239831792));
#52638=CARTESIAN_POINT('Ctrl Pts',(0.682546965339704,-0.462660009720198,
-1.89209488774197));
#52639=CARTESIAN_POINT('Ctrl Pts',(0.82065744871628,-0.0802869625482141,
-1.87623737716603));
#52640=CARTESIAN_POINT('Ctrl Pts',(0.759273382308613,0.321603133390165,
-1.86037986659009));
#52641=CARTESIAN_POINT('Ctrl Pts',(0.51331668842555,0.64531435895427,-1.84452235601415));
#52642=CARTESIAN_POINT('Ctrl Pts',(0.142577258683111,0.812155385252811,
-1.8286648454382));
#52643=CARTESIAN_POINT('Ctrl Pts',(-0.262821438546577,0.781568638015269,
-1.81280733486226));
#52644=CARTESIAN_POINT('Ctrl Pts',(-0.604330574256394,0.560989484311131,
-1.79694982428631));
#52645=CARTESIAN_POINT('Ctrl Pts',(-0.798932305395987,0.204038760737729,
-1.78109231371037));
#52646=CARTESIAN_POINT('Ctrl Pts',(-0.799320676476057,-0.202511976550994,
-1.76523480313443));
#52647=CARTESIAN_POINT('Ctrl Pts',(-0.605401277930371,-0.559833847823624,
-1.74937729255848));
#52648=CARTESIAN_POINT('Ctrl Pts',(-0.264314196244243,-0.781065074211162,
-1.73351978198254));
#52649=CARTESIAN_POINT('Ctrl Pts',(0.141025323123172,-0.812426306028269,
-1.7176622714066));
#52650=CARTESIAN_POINT('Ctrl Pts',(0.512082836778417,-0.646293905870776,
-1.70180476083066));
#52651=CARTESIAN_POINT('Ctrl Pts',(0.758657552970296,-0.32305318727704,
-1.68594725025471));
#52652=CARTESIAN_POINT('Ctrl Pts',(0.820809344338949,0.0787188969346039,
-1.67008973967877));
#52653=CARTESIAN_POINT('Ctrl Pts',(0.683429661444197,0.461355115227956,
-1.65423222910282));
#52654=CARTESIAN_POINT('Ctrl Pts',(0.379914287181169,0.731839995411811,
-1.63837471852688));
#52655=CARTESIAN_POINT('Ctrl Pts',(-0.0159548819525065,0.824421061248809,
-1.62251720795093));
#52656=CARTESIAN_POINT('Ctrl Pts',(-0.407945560740477,0.716592676463325,
-1.606659697375));
#52657=CARTESIAN_POINT('Ctrl Pts',(-0.700768290582505,0.434566965383708,
-1.59080218679905));
#52658=CARTESIAN_POINT('Ctrl Pts',(-0.823240462038068,0.0469018779163698,
-1.57494467622311));
#52659=CARTESIAN_POINT('Ctrl Pts',(-0.74559017607201,-0.352164640237547,
-1.55908716564716));
#52660=CARTESIAN_POINT('Ctrl Pts',(-0.486693528750542,-0.665623056662763,
-1.54322965507122));
#52661=CARTESIAN_POINT('Ctrl Pts',(-0.109485999644142,-0.817274409467625,
-1.52737214449527));
#52662=CARTESIAN_POINT('Ctrl Pts',(0.29433660526624,-0.770253599335362,
-1.51151463391933));
#52663=CARTESIAN_POINT('Ctrl Pts',(0.626608591042582,-0.535990968319769,
-1.49565712334339));
#52664=CARTESIAN_POINT('Ctrl Pts',(0.806557583886217,-0.171433685034062,
-1.47979961276745));
#52665=CARTESIAN_POINT('Ctrl Pts',(0.790439579075549,0.23479760714198,-1.4639421021915));
#52666=CARTESIAN_POINT('Ctrl Pts',(0.582172720676841,0.583951682751627,
-1.44808459161556));
#52667=CARTESIAN_POINT('Ctrl Pts',(0.23238483546022,0.791152281635374,-1.43222708103962));
#52668=CARTESIAN_POINT('Ctrl Pts',(-0.173893742918745,0.806030775257647,
-1.41636957046367));
#52669=CARTESIAN_POINT('Ctrl Pts',(-0.537900294146628,0.624970333732493,
-1.40051205988773));
#52670=CARTESIAN_POINT('Ctrl Pts',(-0.771148052924077,0.291985145101832,
-1.38465454931178));
#52671=CARTESIAN_POINT('Ctrl Pts',(-0.816936557081062,-0.111979043545092,
-1.36879703873584));
#52672=CARTESIAN_POINT('Ctrl Pts',(-0.664135027220673,-0.488722119519188,
-1.3529395281599));
#52673=CARTESIAN_POINT('Ctrl Pts',(-0.349888160504345,-0.746661181278108,
-1.33708201758396));
#52674=CARTESIAN_POINT('Ctrl Pts',(0.0494134159009503,-0.823093529811607,
-1.32122450700801));
#52675=CARTESIAN_POINT('Ctrl Pts',(0.436703029003066,-0.699439138845034,
-1.30536699643207));
#52676=CARTESIAN_POINT('Ctrl Pts',(0.71783400759006,-0.405757294495029,
-1.28950948585612));
#52677=CARTESIAN_POINT('Ctrl Pts',(0.824465903291734,-0.0134394493220526,
-1.27365197528018));
#52678=CARTESIAN_POINT('Ctrl Pts',(0.730677447667856,0.382145406826143,
-1.25779446470424));
#52679=CARTESIAN_POINT('Ctrl Pts',(0.459267782746466,0.684834102699244,
-1.2419369541283));
#52680=CARTESIAN_POINT('Ctrl Pts',(0.0762141917354068,0.821045699986822,
-1.22607944355235));
#52681=CARTESIAN_POINT('Ctrl Pts',(-0.325366393566878,0.757668367048548,
-1.21022193297641));
#52682=CARTESIAN_POINT('Ctrl Pts',(-0.647853293311223,0.510108571614448,
-1.19436442240046));
#52683=CARTESIAN_POINT('Ctrl Pts',(-0.812852801358185,0.138545905074395,
-1.17850691182452));
#52684=CARTESIAN_POINT('Ctrl Pts',(-0.780255000197183,-0.266696042632859,
-1.16264940124858));
#52685=CARTESIAN_POINT('Ctrl Pts',(-0.55798412627637,-0.607106546919343,
-1.14679189067263));
#52686=CARTESIAN_POINT('Ctrl Pts',(-0.200072258378857,-0.799934832293181,
-1.13093438009669));
#52687=CARTESIAN_POINT('Ctrl Pts',(0.206475401677787,-0.798306052207252,
-1.11507686952075));
#52688=CARTESIAN_POINT('Ctrl Pts',(0.562830722209987,-0.602616148659591,
-1.09921935894481));
#52689=CARTESIAN_POINT('Ctrl Pts',(0.782366884264238,-0.260435602204081,
-1.08336184836886));
#52690=CARTESIAN_POINT('Ctrl Pts',(0.811716593266069,0.145054530109405,
-1.06750433779292));
#52691=CARTESIAN_POINT('Ctrl Pts',(0.643745195173435,0.51528319221555,-1.05164682721697));
#52692=CARTESIAN_POINT('Ctrl Pts',(0.31928504761806,0.760251078826112,-1.03578931664103));
#52693=CARTESIAN_POINT('Ctrl Pts',(-0.0827904642126807,0.82040866860619,
-1.01993180606509));
#52694=CARTESIAN_POINT('Ctrl Pts',(-0.464740348218594,0.681132184841088,
-1.00407429548914));
#52695=CARTESIAN_POINT('Ctrl Pts',(-0.733715973988661,0.376278505900353,
-0.988216784913199));
#52696=CARTESIAN_POINT('Ctrl Pts',(-0.824331751652386,-0.0200451417167169,
-0.972359274337258));
#52697=CARTESIAN_POINT('Ctrl Pts',(-0.714559789064689,-0.411495993103893,
-0.956501763761311));
#52698=CARTESIAN_POINT('Ctrl Pts',(-0.431084677085769,-0.702915816915933,
-0.94064425318537));
#52699=CARTESIAN_POINT('Ctrl Pts',(-0.0428167021301743,-0.823463037729944,
-0.924786742609425));
#52700=CARTESIAN_POINT('Ctrl Pts',(0.355859633497782,-0.743833694945016,
-0.908929232033482));
#52701=CARTESIAN_POINT('Ctrl Pts',(0.668029647295509,-0.483384975793587,
-0.89307172145754));
#52702=CARTESIAN_POINT('Ctrl Pts',(0.817807576627052,-0.105429654747237,
-0.877214210881595));
#52703=CARTESIAN_POINT('Ctrl Pts',(0.768783734812105,0.298154680622465,
-0.861356700305653));
#52704=CARTESIAN_POINT('Ctrl Pts',(0.532875383147527,0.629260256590315,
-0.845499189729709));
#52705=CARTESIAN_POINT('Ctrl Pts',(0.16742975034523,0.807398243240637,-0.829641679153766));
#52706=CARTESIAN_POINT('Ctrl Pts',(-0.238716570323675,0.789264875400923,
-0.813784168577821));
#52707=CARTESIAN_POINT('Ctrl Pts',(-0.586833009222479,0.57926821402147,
-0.797926658001879));
#52708=CARTESIAN_POINT('Ctrl Pts',(-0.792295546476325,0.228456585640494,
-0.782069147425936));
#52709=CARTESIAN_POINT('Ctrl Pts',(-0.805158060922119,-0.177890813199751,
-0.766211636849992));
#52710=CARTESIAN_POINT('Ctrl Pts',(-0.622293789337913,-0.540994532541866,
-0.750354126274048));
#52711=CARTESIAN_POINT('Ctrl Pts',(-0.288155414860119,-0.772587277513375,
-0.734496615698105));
#52712=CARTESIAN_POINT('Ctrl Pts',(0.116030986166798,-0.816370905127008,
-0.718639105122162));
#52713=CARTESIAN_POINT('Ctrl Pts',(0.492011283194322,-0.661702003698199,
-0.702781594546217));
#52714=CARTESIAN_POINT('Ctrl Pts',(0.748387999479165,-0.346179211860426,
-0.686924083970274));
#52715=CARTESIAN_POINT('Ctrl Pts',(0.82283822834399,0.053496677134739,-0.671066573394332));
#52716=CARTESIAN_POINT('Ctrl Pts',(0.697263779231996,0.440167998223232,
-0.655209062818386));
#52717=CARTESIAN_POINT('Ctrl Pts',(0.402190687371641,0.719838381499804,
-0.639351552242445));
#52718=CARTESIAN_POINT('Ctrl Pts',(0.00934860525825762,0.824522436364503,
-0.623494041666501));
#52719=CARTESIAN_POINT('Ctrl Pts',(-0.385766039908107,0.728772397214898,
-0.607636531090558));
#52720=CARTESIAN_POINT('Ctrl Pts',(-0.687104380997915,0.455864249642597,
-0.591779020514614));
#52721=CARTESIAN_POINT('Ctrl Pts',(-0.821413738976212,0.0721395447022476,
-0.575921509938671));
#52722=CARTESIAN_POINT('Ctrl Pts',(-0.756044699713402,-0.329121643961638,
-0.560063999362728));
#52723=CARTESIAN_POINT('Ctrl Pts',(-0.506887897088375,-0.650376278990902,
-0.544206488786783));
#52724=CARTESIAN_POINT('Ctrl Pts',(-0.134511140780029,-0.813530206872971,
-0.528348978210842));
#52725=CARTESIAN_POINT('Ctrl Pts',(0.270564081268103,-0.778922154272384,
-0.512491467634896));
#52726=CARTESIAN_POINT('Ctrl Pts',(0.609867573997332,-0.554965031939134,
-0.496633957058954));
#52727=CARTESIAN_POINT('Ctrl Pts',(0.800917666611022,-0.196100830695248,
-0.480776446483009));
#52728=CARTESIAN_POINT('Ctrl Pts',(0.797271775455493,0.210433743849107,
-0.464918935907067));
#52729=CARTESIAN_POINT('Ctrl Pts',(0.599816184347909,0.565813740981475,
-0.449061425331122));
#52730=CARTESIAN_POINT('Ctrl Pts',(0.256550596829474,0.783649434221335,
-0.43320391475518));
#52731=CARTESIAN_POINT('Ctrl Pts',(-0.149080166180136,0.810986897883099,
-0.417346404179236));
#52732=CARTESIAN_POINT('Ctrl Pts',(-0.518470862554774,0.641180636932909,
-0.401488893603293));
#52733=CARTESIAN_POINT('Ctrl Pts',(-0.761825889017629,0.315509047882063,
-0.385631383027349));
#52734=CARTESIAN_POINT('Ctrl Pts',(-0.819987796291551,-0.0868599933696644,
-0.369773872451407));
#52735=CARTESIAN_POINT('Ctrl Pts',(-0.678817940276728,-0.468114140372212,
-0.353916361875461));
#52736=CARTESIAN_POINT('Ctrl Pts',(-0.372633461561838,-0.735573890114115,
-0.33805885129952));
#52737=CARTESIAN_POINT('Ctrl Pts',(0.0241349081417215,-0.824222148937965,
-0.322201340723576));
#52738=CARTESIAN_POINT('Ctrl Pts',(0.415036295122669,-0.712509310712441,
-0.306343830147633));
#52739=CARTESIAN_POINT('Ctrl Pts',(0.705046039541136,-0.427591776684167,
-0.290486319571689));
#52740=CARTESIAN_POINT('Ctrl Pts',(0.823665340687052,-0.0387304718595854,
-0.274628808995746));
#52741=CARTESIAN_POINT('Ctrl Pts',(0.742058904165613,0.35954586545316,-0.258771298419802));
#52742=CARTESIAN_POINT('Ctrl Pts',(0.480064519393053,0.670419794212498,
-0.242913787843858));
#52743=CARTESIAN_POINT('Ctrl Pts',(0.101370721449253,0.818320607982799,
-0.227056277267916));
#52744=CARTESIAN_POINT('Ctrl Pts',(-0.301965429834451,0.767294950903153,
-0.211198766691971));
#52745=CARTESIAN_POINT('Ctrl Pts',(-0.631896404326232,0.529746667439074,
-0.195341256116028));
#52746=CARTESIAN_POINT('Ctrl Pts',(-0.808219078736472,0.163421718047794,
-0.179483745540085));
#52747=CARTESIAN_POINT('Ctrl Pts',(-0.78807063935742,-0.242629703983174,
-0.163626234964142));
#52748=CARTESIAN_POINT('Ctrl Pts',(-0.576349647237178,-0.589699797120169,
-0.147768724388197));
#52749=CARTESIAN_POINT('Ctrl Pts',(-0.224522320795394,-0.793419486658044,
-0.131911213812255));
#52750=CARTESIAN_POINT('Ctrl Pts',(0.181882740561737,-0.804265174094747,
-0.116053703236311));
#52751=CARTESIAN_POINT('Ctrl Pts',(0.544076944580878,-0.619602611767352,
-0.100196192660367));
#52752=CARTESIAN_POINT('Ctrl Pts',(0.77400456870953,-0.284317250155574,
-0.0843386820844249));
#52753=CARTESIAN_POINT('Ctrl Pts',(0.815790850594378,0.120077451582211,
-0.0684811715084816));
#52754=CARTESIAN_POINT('Ctrl Pts',(0.659241540883417,0.495293473818102,
-0.0526236609325374));
#52755=CARTESIAN_POINT('Ctrl Pts',(0.342483797368491,0.750086144974063,
-0.0367661503565947));
#52756=CARTESIAN_POINT('Ctrl Pts',(-0.0576246440758148,0.822584922815185,
-0.0209086397806512));
#52757=CARTESIAN_POINT('Ctrl Pts',(-0.314875021606723,0.737530279563956,
-0.0103369660633551));
#52758=CARTESIAN_POINT('Ctrl Pts',(-0.42561232635123,0.666853325445629,
-0.00505112920470729));
#52759=CARTESIAN_POINT('Ctrl Pts',(-0.79104322765544,1.14479096649424E-5,
-0.173133150823705));
#52760=CARTESIAN_POINT('Ctrl Pts',(-0.791002750150416,-0.0787621090845962,
-0.169964178870517));
#52761=CARTESIAN_POINT('Ctrl Pts',(-0.779310325630016,-0.157547413537066,
-0.166795206917329));
#52762=CARTESIAN_POINT('Ctrl Pts',(-0.756141880567222,-0.232799482500845,
-0.163626234964141));
#52763=CARTESIAN_POINT('Ctrl Pts',(-0.717496975317341,-0.358319735028833,
-0.158340398105494));
#52764=CARTESIAN_POINT('Ctrl Pts',(-0.646923311277268,-0.47400976607449,
-0.153054561246846));
#52765=CARTESIAN_POINT('Ctrl Pts',(-0.552998591516937,-0.565808063186967,
-0.147768724388198));
#52766=CARTESIAN_POINT('Ctrl Pts',(-0.459073871756601,-0.657606360299449,
-0.14248288752955));
#52767=CARTESIAN_POINT('Ctrl Pts',(-0.341798096276011,-0.725512923478742,
-0.137197050670903));
#52768=CARTESIAN_POINT('Ctrl Pts',(-0.215426031642858,-0.761273819641176,
-0.131911213812255));
#52769=CARTESIAN_POINT('Ctrl Pts',(-0.0890539670096971,-0.797034715803612,
-0.126625376953607));
#52770=CARTESIAN_POINT('Ctrl Pts',(0.0464143867760402,-0.80064994494918,
-0.121339540094958));
#52771=CARTESIAN_POINT('Ctrl Pts',(0.174514264338762,-0.771680465800725,
-0.11605370323631));
#52772=CARTESIAN_POINT('Ctrl Pts',(0.302614141901469,-0.742710986652273,
-0.110767866377662));
#52773=CARTESIAN_POINT('Ctrl Pts',(0.423345543241174,-0.681156799209811,
-0.105482029519015));
#52774=CARTESIAN_POINT('Ctrl Pts',(0.522032514599136,-0.594498811886617,
-0.100196192660367));
#52775=CARTESIAN_POINT('Ctrl Pts',(0.620719485957098,-0.507840824563423,
-0.0949103558017196));
#52776=CARTESIAN_POINT('Ctrl Pts',(0.697362027333311,-0.396079037359503,
-0.0896245189430725));
#52777=CARTESIAN_POINT('Ctrl Pts',(0.74264767833556,-0.272799026801247,
-0.084338682084425));
#52778=CARTESIAN_POINT('Ctrl Pts',(0.780454516535908,-0.169878403836554,
-0.0799257880562837));
#52779=CARTESIAN_POINT('Ctrl Pts',(0.796406271019666,-0.0589298248892024,
-0.0755128940281423));
#52780=CARTESIAN_POINT('Ctrl Pts',(0.789514313045754,0.0505148300805575,
-0.0711000000000008));
#52781=CARTESIAN_POINT('',(-0.392914465807693,-0.550975791759097,-5.8089));
#52782=CARTESIAN_POINT('Ctrl Pts',(-0.392914465807689,-0.5509757917591,
-5.8089));
#52783=CARTESIAN_POINT('Ctrl Pts',(-0.408980926181822,-0.541406672716214,
-5.8089));
#52784=CARTESIAN_POINT('Ctrl Pts',(-0.424624980889038,-0.531181210689783,
-5.8089));
#52785=CARTESIAN_POINT('Ctrl Pts',(-0.439803506503688,-0.520323148404966,
-5.8089));
#52786=CARTESIAN_POINT('Ctrl Pts',(-0.463323139664173,-0.503498217693243,
-5.8089));
#52787=CARTESIAN_POINT('Ctrl Pts',(-0.485725932404054,-0.485155747624265,
-5.8089));
#52788=CARTESIAN_POINT('Ctrl Pts',(-0.50691755469692,-0.465448611131913,
-5.8089));
#52789=CARTESIAN_POINT('Ctrl Pts',(-0.514827455118625,-0.458092803959758,
-5.8089));
#52790=CARTESIAN_POINT('Ctrl Pts',(-0.522568471664888,-0.450546591655005,
-5.8089));
#52791=CARTESIAN_POINT('Ctrl Pts',(-0.530135111219165,-0.442816995778067,
-5.8089));
#52792=CARTESIAN_POINT('Ctrl Pts',(-0.53611345887652,-0.436709897498611,
-5.8089));
#52793=CARTESIAN_POINT('Ctrl Pts',(-0.541980440975214,-0.430490694480234,
-5.8089));
#52794=CARTESIAN_POINT('Ctrl Pts',(-0.547726899698063,-0.424170679860769,
-5.8089));
#52795=CARTESIAN_POINT('Ctrl Pts',(-0.570445604559277,-0.399184413747471,
-5.8089));
#52796=CARTESIAN_POINT('Ctrl Pts',(-0.591314828543991,-0.372593498230057,
-5.8089));
#52797=CARTESIAN_POINT('Ctrl Pts',(-0.610184365647462,-0.344628549984071,
-5.8089));
#52798=CARTESIAN_POINT('Ctrl Pts',(-0.617410130397325,-0.333919853943486,
-5.8089));
#52799=CARTESIAN_POINT('Ctrl Pts',(-0.624342346784469,-0.32300922386781,
-5.8089));
#52800=CARTESIAN_POINT('Ctrl Pts',(-0.630971222773021,-0.311908104829863,
-5.8089));
#52801=CARTESIAN_POINT('Ctrl Pts',(-0.63528392404581,-0.304685792889344,
-5.8089));
#52802=CARTESIAN_POINT('Ctrl Pts',(-0.639468933149375,-0.297381521670017,
-5.8089));
#52803=CARTESIAN_POINT('Ctrl Pts',(-0.64352110345146,-0.290002386427528,
-5.8089));
#52804=CARTESIAN_POINT('Ctrl Pts',(-0.649505567320399,-0.279104481119854,
-5.8089));
#52805=CARTESIAN_POINT('Ctrl Pts',(-0.655190978687311,-0.268060576369735,
-5.8089));
#52806=CARTESIAN_POINT('Ctrl Pts',(-0.660570869537721,-0.256882390369936,
-5.8089));
#52807=CARTESIAN_POINT('Ctrl Pts',(-0.675323401225404,-0.226229994669333,
-5.8089));
#52808=CARTESIAN_POINT('Ctrl Pts',(-0.687781723263565,-0.194570433662548,
-5.8089));
#52809=CARTESIAN_POINT('Ctrl Pts',(-0.697948790393408,-0.162181035562999,
-5.8089));
#52810=CARTESIAN_POINT('Ctrl Pts',(-0.708208146688207,-0.129497630306234,
-5.8089));
#52811=CARTESIAN_POINT('Ctrl Pts',(-0.716134890556743,-0.0960699249494282,
-5.8089));
#52812=CARTESIAN_POINT('Ctrl Pts',(-0.72168597652701,-0.0621561899810933,
-5.8089));
#52813=CARTESIAN_POINT('Ctrl Pts',(-0.723441122832596,-0.0514333211663941,
-5.8089));
#52814=CARTESIAN_POINT('Ctrl Pts',(-0.724958404602569,-0.0406617363995879,
-5.8089));
#52815=CARTESIAN_POINT('Ctrl Pts',(-0.726235405139263,-0.0298493434138636,
-5.8089));
#52816=CARTESIAN_POINT('Ctrl Pts',(-0.727115833463151,-0.0223947364970243,
-5.8089));
#52817=CARTESIAN_POINT('Ctrl Pts',(-0.727881038038328,-0.0149287234917137,
-5.8089));
#52818=CARTESIAN_POINT('Ctrl Pts',(-0.728530533992226,-0.00745907930554179,
-5.8089));
#52819=CARTESIAN_POINT('Ctrl Pts',(-0.731453588396324,0.0261580297840189,
-5.8089));
#52820=CARTESIAN_POINT('Ctrl Pts',(-0.732040069074509,0.0598791137304111,
-5.8089));
#52821=CARTESIAN_POINT('Ctrl Pts',(-0.730275016954016,0.0934581668363401,
-5.8089));
#52822=CARTESIAN_POINT('Ctrl Pts',(-0.728639353757938,0.124575673615201,
-5.8089));
#52823=CARTESIAN_POINT('Ctrl Pts',(-0.724984137270265,0.155572115372472,
-5.8089));
#52824=CARTESIAN_POINT('Ctrl Pts',(-0.719387035599625,0.186273529871663,
-5.8089));
#52825=CARTESIAN_POINT('Ctrl Pts',(-0.716174207421376,0.203896645444594,
-5.8089));
#52826=CARTESIAN_POINT('Ctrl Pts',(-0.712320910059993,0.221422620213725,
-5.8089));
#52827=CARTESIAN_POINT('Ctrl Pts',(-0.707836932295669,0.238818219202657,
-5.8089));
#52828=CARTESIAN_POINT('Ctrl Pts',(-0.705076172277217,0.249528592159403,
-5.8089));
#52829=CARTESIAN_POINT('Ctrl Pts',(-0.70207408761155,0.260195841798999,
-5.8089));
#52830=CARTESIAN_POINT('Ctrl Pts',(-0.698843635371611,0.270777419289408,
-5.8089));
#52831=CARTESIAN_POINT('Ctrl Pts',(-0.68835492234885,0.305133949391549,
-5.8089));
#52832=CARTESIAN_POINT('Ctrl Pts',(-0.675451834043792,0.338642319424662,
-5.8089));
#52833=CARTESIAN_POINT('Ctrl Pts',(-0.66026439737455,0.371047946919152,
-5.8089));
#52834=CARTESIAN_POINT('Ctrl Pts',(-0.648020670392897,0.397172543475675,
-5.8089));
#52835=CARTESIAN_POINT('Ctrl Pts',(-0.634291186315133,0.422580902638274,
-5.8089));
#52836=CARTESIAN_POINT('Ctrl Pts',(-0.619119721284794,0.447135948712967,
-5.8089));
#52837=CARTESIAN_POINT('Ctrl Pts',(-0.610224791501901,0.46153241011029,
-5.8089));
#52838=CARTESIAN_POINT('Ctrl Pts',(-0.600833791321736,0.475635447480755,
-5.8089));
#52839=CARTESIAN_POINT('Ctrl Pts',(-0.590967220284706,0.489427201169085,
-5.8089));
#52840=CARTESIAN_POINT('Ctrl Pts',(-0.585636455339572,0.496878685257906,
-5.8089));
#52841=CARTESIAN_POINT('Ctrl Pts',(-0.580166827791742,0.504239280109289,
-5.8089));
#52842=CARTESIAN_POINT('Ctrl Pts',(-0.57456130958788,0.511505986352523,
-5.8089));
#52843=CARTESIAN_POINT('Ctrl Pts',(-0.570041164021464,0.517365671186865,
-5.8089));
#52844=CARTESIAN_POINT('Ctrl Pts',(-0.565432977871958,0.523163672746738,
-5.8089));
#52845=CARTESIAN_POINT('Ctrl Pts',(-0.560747049034941,0.528888278685951,
-5.8089));
#52846=CARTESIAN_POINT('Ctrl Pts',(-0.537735453820515,0.55700059520144,
-5.8089));
#52847=CARTESIAN_POINT('Ctrl Pts',(-0.512802538579046,0.58341098831171,
-5.8089));
#52848=CARTESIAN_POINT('Ctrl Pts',(-0.48618644515188,0.607969808368677,
-5.8089));
#52849=CARTESIAN_POINT('Ctrl Pts',(-0.459352739467097,0.632729420487471,
-5.8089));
#52850=CARTESIAN_POINT('Ctrl Pts',(-0.430807455342091,0.655608007637476,
-5.8089));
#52851=CARTESIAN_POINT('Ctrl Pts',(-0.400750465327347,0.676424420620533,
-5.8089));
#52852=CARTESIAN_POINT('Ctrl Pts',(-0.381778290006706,0.689563881240766,
-5.8089));
#52853=CARTESIAN_POINT('Ctrl Pts',(-0.362202973049296,0.701881127216335,
-5.8089));
#52854=CARTESIAN_POINT('Ctrl Pts',(-0.342067962509752,0.713322310757506,
-5.8089));
#52855=CARTESIAN_POINT('Ctrl Pts',(-0.392914465807693,-0.550975791759097,
-5.8089));
#52856=CARTESIAN_POINT('Ctrl Pts',(-0.316486804163133,-0.605362341937418,
-5.80448710597186));
#52857=CARTESIAN_POINT('Ctrl Pts',(-0.123459254944096,-0.689898673908607,
-5.79478837508506));
#52858=CARTESIAN_POINT('Ctrl Pts',(0.204815806457288,-0.674943835808658,
-5.77980380733964));
#52859=CARTESIAN_POINT('Ctrl Pts',(0.502426729513632,-0.495039039708356,
-5.76394629676369));
#52860=CARTESIAN_POINT('Ctrl Pts',(0.677901792498161,-0.194797654574707,
-5.74808878618775));
#52861=CARTESIAN_POINT('Ctrl Pts',(0.688585132880224,0.152798855491627,
-5.7322312756118));
#52862=CARTESIAN_POINT('Ctrl Pts',(0.531879433776216,0.463250529001845,
-5.71637376503586));
#52863=CARTESIAN_POINT('Ctrl Pts',(0.245878610535506,0.661090510301056,
-5.70051625445991));
#52864=CARTESIAN_POINT('Ctrl Pts',(-0.0998931488246837,0.698225042897434,
-5.68465874388397));
#52865=CARTESIAN_POINT('Ctrl Pts',(-0.421381756118886,0.565627364000294,
-5.66880123330803));
#52866=CARTESIAN_POINT('Ctrl Pts',(-0.630785750431968,0.307429753987566,
-5.65364232588638));
#52867=CARTESIAN_POINT('Ctrl Pts',(-0.676646139866951,0.0974912420182623,
-5.64376925532336));
#52868=CARTESIAN_POINT('Ctrl Pts',(-0.676733793626987,-1.34876458775003E-5,
-5.639182021619));
#52869=CARTESIAN_POINT('Origin',(-1.87869726832665E-16,-4.25270154953079E-17,
-5.8089));
#52870=CARTESIAN_POINT('',(-0.7911,-9.68818082805472E-17,-5.8089));
#52871=CARTESIAN_POINT('Origin',(0.,0.,-5.8089));
#52872=CARTESIAN_POINT('Origin',(0.,0.,-5.8089));
#52873=CARTESIAN_POINT('',(0.392888236737269,-0.550964357679769,-5.8089));
#52874=CARTESIAN_POINT('Ctrl Pts',(0.342095882030763,0.713340734875808,
-5.8089));
#52875=CARTESIAN_POINT('Ctrl Pts',(0.360978708681145,0.702635258820052,
-5.8089));
#52876=CARTESIAN_POINT('Ctrl Pts',(0.379389322783699,0.69116424080316,-5.8089));
#52877=CARTESIAN_POINT('Ctrl Pts',(0.397274912114345,0.678942925746265,
-5.8089));
#52878=CARTESIAN_POINT('Ctrl Pts',(0.423819765578583,0.660804691029575,
-5.8089));
#52879=CARTESIAN_POINT('Ctrl Pts',(0.449209359364097,0.641014492048834,
-5.8089));
#52880=CARTESIAN_POINT('Ctrl Pts',(0.47331366889555,0.619707152111731,-5.8089));
#52881=CARTESIAN_POINT('Ctrl Pts',(0.482766815899108,0.611350911232175,
-5.8089));
#52882=CARTESIAN_POINT('Ctrl Pts',(0.492022026358695,0.602761124068153,
-5.8089));
#52883=CARTESIAN_POINT('Ctrl Pts',(0.501070383515418,0.593945229113476,
-5.8089));
#52884=CARTESIAN_POINT('Ctrl Pts',(0.507461516366784,0.587718291462461,
-5.8089));
#52885=CARTESIAN_POINT('Ctrl Pts',(0.513748498043816,0.581379258677312,
-5.8089));
#52886=CARTESIAN_POINT('Ctrl Pts',(0.519919868452944,0.574939912035177,
-5.8089));
#52887=CARTESIAN_POINT('Ctrl Pts',(0.545883770341496,0.547848593031625,
-5.8089));
#52888=CARTESIAN_POINT('Ctrl Pts',(0.569847963303607,0.518943292978646,
-5.8089));
#52889=CARTESIAN_POINT('Ctrl Pts',(0.59159745395337,0.488437514575107,-5.8089));
#52890=CARTESIAN_POINT('Ctrl Pts',(0.604843734393337,0.469858316455947,
-5.8089));
#52891=CARTESIAN_POINT('Ctrl Pts',(0.617267589027075,0.450684778561505,
-5.8089));
#52892=CARTESIAN_POINT('Ctrl Pts',(0.628810161645074,0.430960931745118,
-5.8089));
#52893=CARTESIAN_POINT('Ctrl Pts',(0.6331957498372,0.423466877121077,-5.8089));
#52894=CARTESIAN_POINT('Ctrl Pts',(0.637450247091553,0.415899644987057,
-5.8089));
#52895=CARTESIAN_POINT('Ctrl Pts',(0.641567501202037,0.408268535811919,
-5.8089));
#52896=CARTESIAN_POINT('Ctrl Pts',(0.644406436656658,0.403006721550756,
-5.8089));
#52897=CARTESIAN_POINT('Ctrl Pts',(0.647180685228449,0.3977135715039,-5.8089));
#52898=CARTESIAN_POINT('Ctrl Pts',(0.649889438922888,0.39238997845085,-5.8089));
#52899=CARTESIAN_POINT('Ctrl Pts',(0.666049099676394,0.360630923390353,
-5.8089));
#52900=CARTESIAN_POINT('Ctrl Pts',(0.679881889293971,0.327789779259877,
-5.8089));
#52901=CARTESIAN_POINT('Ctrl Pts',(0.69133700537052,0.294133909535164,-5.8089));
#52902=CARTESIAN_POINT('Ctrl Pts',(0.702691657190659,0.260773210274299,
-5.8089));
#52903=CARTESIAN_POINT('Ctrl Pts',(0.711710261928255,0.226610762787482,
-5.8089));
#52904=CARTESIAN_POINT('Ctrl Pts',(0.718293067787738,0.19190153845702,-5.8089));
#52905=CARTESIAN_POINT('Ctrl Pts',(0.720274770820946,0.181452593644697,
-5.8089));
#52906=CARTESIAN_POINT('Ctrl Pts',(0.722035372085814,0.170954128586943,
-5.8089));
#52907=CARTESIAN_POINT('Ctrl Pts',(0.723571223099844,0.160413260727799,
-5.8089));
#52908=CARTESIAN_POINT('Ctrl Pts',(0.724609888773418,0.153284680211231,
-5.8089));
#52909=CARTESIAN_POINT('Ctrl Pts',(0.725545495635983,0.146137630688022,
-5.8089));
#52910=CARTESIAN_POINT('Ctrl Pts',(0.726375786214834,0.138987023116276,
-5.8089));
#52911=CARTESIAN_POINT('Ctrl Pts',(0.730471171823078,0.103716846523315,
-5.8089));
#52912=CARTESIAN_POINT('Ctrl Pts',(0.732021347863029,0.0682782853423011,
-5.8089));
#52913=CARTESIAN_POINT('Ctrl Pts',(0.730953058964537,0.032934252799972,
-5.8089));
#52914=CARTESIAN_POINT('Ctrl Pts',(0.730050923290943,0.00308735216280863,
-5.8089));
#52915=CARTESIAN_POINT('Ctrl Pts',(0.727280342640496,-0.0266927166244539,
-5.8089));
#52916=CARTESIAN_POINT('Ctrl Pts',(0.722676929026824,-0.0562354887167472,
-5.8089));
#52917=CARTESIAN_POINT('Ctrl Pts',(0.720230454191575,-0.0719359350708675,
-5.8089));
#52918=CARTESIAN_POINT('Ctrl Pts',(0.717265866279696,-0.0875692069311204,
-5.8089));
#52919=CARTESIAN_POINT('Ctrl Pts',(0.713785605356316,-0.103108175325424,
-5.8089));
#52920=CARTESIAN_POINT('Ctrl Pts',(0.712112783672321,-0.110577133501022,
-5.8089));
#52921=CARTESIAN_POINT('Ctrl Pts',(0.710320795535734,-0.11802428479304,
-5.8089));
#52922=CARTESIAN_POINT('Ctrl Pts',(0.708409758051769,-0.125446495005051,
-5.8089));
#52923=CARTESIAN_POINT('Ctrl Pts',(0.706492764579635,-0.132891837466731,
-5.8089));
#52924=CARTESIAN_POINT('Ctrl Pts',(0.704458175001798,-0.140303361495487,
-5.8089));
#52925=CARTESIAN_POINT('Ctrl Pts',(0.702308221058893,-0.147673812311276,
-5.8089));
#52926=CARTESIAN_POINT('Ctrl Pts',(0.692801581982461,-0.1802643782476,-5.8089));
#52927=CARTESIAN_POINT('Ctrl Pts',(0.681035781348705,-0.212081758477362,
-5.8089));
#52928=CARTESIAN_POINT('Ctrl Pts',(0.667074534284358,-0.242877043678588,
-5.8089));
#52929=CARTESIAN_POINT('Ctrl Pts',(0.656923567387669,-0.265267731216093,
-5.8089));
#52930=CARTESIAN_POINT('Ctrl Pts',(0.645610925501866,-0.287117873412337,
-5.8089));
#52931=CARTESIAN_POINT('Ctrl Pts',(0.633146702390696,-0.308322081618923,
-5.8089));
#52932=CARTESIAN_POINT('Ctrl Pts',(0.625027380935961,-0.322134718081451,
-5.8089));
#52933=CARTESIAN_POINT('Ctrl Pts',(0.616419131041242,-0.335673062825433,
-5.8089));
#52934=CARTESIAN_POINT('Ctrl Pts',(0.607339031883614,-0.348913919627164,
-5.8089));
#52935=CARTESIAN_POINT('Ctrl Pts',(0.602580680409358,-0.355852682011713,
-5.8089));
#52936=CARTESIAN_POINT('Ctrl Pts',(0.597692725339706,-0.362709713037344,
-5.8089));
#52937=CARTESIAN_POINT('Ctrl Pts',(0.592677481645101,-0.369481424925529,
-5.8089));
#52938=CARTESIAN_POINT('Ctrl Pts',(0.588934360991923,-0.374535483346122,
-5.8089));
#52939=CARTESIAN_POINT('Ctrl Pts',(0.585121098221576,-0.379540835606088,
-5.8089));
#52940=CARTESIAN_POINT('Ctrl Pts',(0.581244810866683,-0.384488631805347,
-5.8089));
#52941=CARTESIAN_POINT('Ctrl Pts',(0.56068130673256,-0.410736434995127,
-5.8089));
#52942=CARTESIAN_POINT('Ctrl Pts',(0.53830293915685,-0.435427816819282,
-5.8089));
#52943=CARTESIAN_POINT('Ctrl Pts',(0.514295529224174,-0.45838419708911,
-5.8089));
#52944=CARTESIAN_POINT('Ctrl Pts',(0.490732143299865,-0.480915992448961,
-5.8089));
#52945=CARTESIAN_POINT('Ctrl Pts',(0.465598395457484,-0.501777006704631,
-5.8089));
#52946=CARTESIAN_POINT('Ctrl Pts',(0.439043415987534,-0.52075707530173,
-5.8089));
#52947=CARTESIAN_POINT('Ctrl Pts',(0.424100596267082,-0.531437397749323,
-5.8089));
#52948=CARTESIAN_POINT('Ctrl Pts',(0.408707354130667,-0.541521326150454,
-5.8089));
#52949=CARTESIAN_POINT('Ctrl Pts',(0.392888236737257,-0.550964357679777,
-5.8089));
#52950=CARTESIAN_POINT('Origin',(0.,0.,-5.8089));
#52951=CARTESIAN_POINT('Origin',(0.,0.,-6.17861797838101));
#52952=CARTESIAN_POINT('Ctrl Pts',(0.392888236737257,-0.550964357679777,
-5.8089));
#52953=CARTESIAN_POINT('Ctrl Pts',(0.484381081792765,-0.485721548291323,
-5.80361416314135));
#52954=CARTESIAN_POINT('Ctrl Pts',(0.634146933675295,-0.308844853941977,
-5.79304248942406));
#52955=CARTESIAN_POINT('Ctrl Pts',(0.70461890056211,0.0317634872067408,
-5.77718497884811));
#52956=CARTESIAN_POINT('Ctrl Pts',(0.603809517943593,0.364559903875637,
-5.76132746827217));
#52957=CARTESIAN_POINT('Ctrl Pts',(0.356217202446025,0.608779534529828,
-5.74546995769622));
#52958=CARTESIAN_POINT('Ctrl Pts',(0.0220327184609351,0.704987657002684,
-5.72961244712028));
#52959=CARTESIAN_POINT('Ctrl Pts',(-0.317508269912238,0.629831081602948,
-5.71375493654434));
#52960=CARTESIAN_POINT('Ctrl Pts',(-0.5798655339509,0.401562243999013,-5.6978974259684));
#52961=CARTESIAN_POINT('Ctrl Pts',(-0.669529242576081,0.160866553025884,
-5.68618510658062));
#52962=CARTESIAN_POINT('Ctrl Pts',(-0.676730232498528,0.024265518019747,
-5.67975862405149));
#52963=CARTESIAN_POINT('Ctrl Pts',(-0.676705286336412,1.73782512660377E-5,
-5.678617978381));
#52964=CARTESIAN_POINT('Ctrl Pts',(0.459308237155092,-0.644108029201221,
-5.87494887079529));
#52965=CARTESIAN_POINT('Ctrl Pts',(0.566268470232396,-0.567835550248648,
-5.86966303393665));
#52966=CARTESIAN_POINT('Ctrl Pts',(0.741353094769514,-0.361056840480996,
-5.85909136021935));
#52967=CARTESIAN_POINT('Ctrl Pts',(0.823738750162087,0.0371332861375223,
-5.8432338496434));
#52968=CARTESIAN_POINT('Ctrl Pts',(0.705886965634953,0.426190837824773,
-5.82737633906747));
#52969=CARTESIAN_POINT('Ctrl Pts',(0.416437755068778,0.711697191911558,
-5.81151882849151));
#52970=CARTESIAN_POINT('Ctrl Pts',(0.0257574753575252,0.824169846985109,
-5.79566131791559));
#52971=CARTESIAN_POINT('Ctrl Pts',(-0.371184856402511,0.736307623254158,
-5.77980380733962));
#52972=CARTESIAN_POINT('Ctrl Pts',(-0.677895114391254,0.469448634886378,
-5.7639462967637));
#52973=CARTESIAN_POINT('Ctrl Pts',(-0.819815247198737,0.0884743817256807,
-5.74808878618774));
#52974=CARTESIAN_POINT('Ctrl Pts',(-0.762445476544219,-0.314009019036856,
-5.73223127561181));
#52975=CARTESIAN_POINT('Ctrl Pts',(-0.519732014137197,-0.640158685018968,
-5.71637376503586));
#52976=CARTESIAN_POINT('Ctrl Pts',(-0.150676284699232,-0.810691924431145,
-5.70051625445991));
#52977=CARTESIAN_POINT('Ctrl Pts',(0.255007502195102,-0.78415290202513,
-5.68465874388398));
#52978=CARTESIAN_POINT('Ctrl Pts',(0.598701232077407,-0.566993385664642,
-5.66880123330802));
#52979=CARTESIAN_POINT('Ctrl Pts',(0.796855997564115,-0.212002740690496,
-5.65294372273209));
#52980=CARTESIAN_POINT('Ctrl Pts',(0.801302136551466,0.194523858387913,
-5.63708621215614));
#52981=CARTESIAN_POINT('Ctrl Pts',(0.610958829750896,0.553763448800768,
-5.6212287015802));
#52982=CARTESIAN_POINT('Ctrl Pts',(0.272096848637962,0.778388045989811,
-5.60537119100425));
#52983=CARTESIAN_POINT('Ctrl Pts',(-0.132909464157486,0.813793414795239,
-5.58951368042832));
#52984=CARTESIAN_POINT('Ctrl Pts',(-0.505606664494294,0.651372817373753,
-5.57365616985236));
#52985=CARTESIAN_POINT('Ctrl Pts',(-0.755395367485779,0.330609264301904,
-5.55779865927643));
#52986=CARTESIAN_POINT('Ctrl Pts',(-0.821554153994998,-0.0705224703046039,
-5.54194114870049));
#52987=CARTESIAN_POINT('Ctrl Pts',(-0.688000409631081,-0.454510817337334,
-5.52608363812453));
#52988=CARTESIAN_POINT('Ctrl Pts',(-0.387199865531956,-0.728011614548961,
-5.5102261275486));
#52989=CARTESIAN_POINT('Ctrl Pts',(0.00772553293681073,-0.824539242780456,
-5.49436861697264));
#52990=CARTESIAN_POINT('Ctrl Pts',(0.400772922845576,-0.720628691547045,
-5.47851110639671));
#52991=CARTESIAN_POINT('Ctrl Pts',(0.696395968486637,-0.441539694515675,
-5.46265359582076));
#52992=CARTESIAN_POINT('Ctrl Pts',(0.822731328477964,-0.05511631247575,
-5.44679608524482));
#52993=CARTESIAN_POINT('Ctrl Pts',(0.74906799690187,0.344705356467844,-5.43093857466887));
#52994=CARTESIAN_POINT('Ctrl Pts',(0.493312876561327,0.660732209429935,
-5.41508106409294));
#52995=CARTESIAN_POINT('Ctrl Pts',(0.117637769670523,0.816140920372838,
-5.39922355351699));
#52996=CARTESIAN_POINT('Ctrl Pts',(-0.286634036043552,0.773153009527251,
-5.38336604294105));
#52997=CARTESIAN_POINT('Ctrl Pts',(-0.621227648910197,0.542218456887407,
-5.3675085323651));
#52998=CARTESIAN_POINT('Ctrl Pts',(-0.804806328168754,0.179475404719749,
-5.35165102178917));
#52999=CARTESIAN_POINT('Ctrl Pts',(-0.792743724511181,-0.226896527095366,
-5.33579351121321));
#53000=CARTESIAN_POINT('Ctrl Pts',(-0.587972149938848,-0.578111924852009,
-5.31993600063728));
#53001=CARTESIAN_POINT('Ctrl Pts',(-0.240269758713106,-0.788793439252471,
-5.30407849006133));
#53002=CARTESIAN_POINT('Ctrl Pts',(0.165840080609549,-0.807726262061115,
-5.28822097948539));
#53003=CARTESIAN_POINT('Ctrl Pts',(0.531635666684229,-0.630307991912695,
-5.27236346890943));
#53004=CARTESIAN_POINT('Ctrl Pts',(0.76819533570202,-0.299667437279164,
-5.25650595833351));
#53005=CARTESIAN_POINT('Ctrl Pts',(0.818013529477059,0.103819614487269,
-5.24064844775755));
#53006=CARTESIAN_POINT('Ctrl Pts',(0.668979886793761,0.482069038442842,
-5.22479093718162));
#53007=CARTESIAN_POINT('Ctrl Pts',(0.357323164847127,0.743131753206276,
-5.20893342660566));
#53008=CARTESIAN_POINT('Ctrl Pts',(-0.041195650425007,0.823545727416433,
-5.19307591602973));
#53009=CARTESIAN_POINT('Ctrl Pts',(-0.429700168321956,0.703763036897992,
-5.17721840545378));
#53010=CARTESIAN_POINT('Ctrl Pts',(-0.713748385047573,0.412901791715392,
-5.16136089487784));
#53011=CARTESIAN_POINT('Ctrl Pts',(-0.824290697504572,0.0216677817790976,
-5.1455033843019));
#53012=CARTESIAN_POINT('Ctrl Pts',(-0.734455249609499,-0.37483347379983,
-5.12964587372595));
#53013=CARTESIAN_POINT('Ctrl Pts',(-0.466080242259121,-0.68021603519432,
-5.11378836315001));
#53014=CARTESIAN_POINT('Ctrl Pts',(-0.0844052603112262,-0.82024410926967,
-5.09793085257406));
#53015=CARTESIAN_POINT('Ctrl Pts',(0.317787892076171,-0.760878112715554,
-5.08207334199813));
#53016=CARTESIAN_POINT('Ctrl Pts',(0.642729625426568,-0.516549392951754,
-5.06621583142217));
#53017=CARTESIAN_POINT('Ctrl Pts',(0.811429485315579,-0.146652095519609,
-5.05035832084624));
#53018=CARTESIAN_POINT('Ctrl Pts',(0.782878031507377,0.258895026106984,
-5.03450081027029));
#53019=CARTESIAN_POINT('Ctrl Pts',(0.564015869283808,0.601507062265964,
-5.01864329969435));
#53020=CARTESIAN_POINT('Ctrl Pts',(0.208046449836234,0.797898064586159,
-5.0027857891184));
#53021=CARTESIAN_POINT('Ctrl Pts',(-0.198497217014094,0.800327121618067,
-4.98692827854246));
#53022=CARTESIAN_POINT('Ctrl Pts',(-0.556787970296653,0.608203751133396,
-4.97107076796652));
#53023=CARTESIAN_POINT('Ctrl Pts',(-0.779728504515992,0.26823144111952,
-4.95521325739057));
#53024=CARTESIAN_POINT('Ctrl Pts',(-0.813123952407679,-0.136945554074297,
-4.93935574681463));
#53025=CARTESIAN_POINT('Ctrl Pts',(-0.648856176675305,-0.508832299240237,
-4.92349823623868));
#53026=CARTESIAN_POINT('Ctrl Pts',(-0.326857217191358,-0.75702642379888,
-4.90764072566275));
#53027=CARTESIAN_POINT('Ctrl Pts',(0.0745978338559104,-0.821194136574177,
-4.8917832150868));
#53028=CARTESIAN_POINT('Ctrl Pts',(0.45791881288172,-0.68573683550528,-4.87592570451086));
#53029=CARTESIAN_POINT('Ctrl Pts',(0.729923788431936,-0.383582989509403,
-4.86006819393491));
#53030=CARTESIAN_POINT('Ctrl Pts',(0.824490762562902,0.0118164803661736,
-4.84421068335898));
#53031=CARTESIAN_POINT('Ctrl Pts',(0.718631342299906,0.404343468630367,
-4.82835317278302));
#53032=CARTESIAN_POINT('Ctrl Pts',(0.438079014152841,0.698578144604221,
-4.81249566220709));
#53033=CARTESIAN_POINT('Ctrl Pts',(0.0510335617003136,0.822994667260962,
-4.79663815163113));
#53034=CARTESIAN_POINT('Ctrl Pts',(-0.348417697134908,0.747348483027167,
-4.7807806410552));
#53035=CARTESIAN_POINT('Ctrl Pts',(-0.663171702889056,0.490028508606418,
-4.76492313047925));
#53036=CARTESIAN_POINT('Ctrl Pts',(-0.816714547391389,0.113586948365908,
-4.74906561990331));
#53037=CARTESIAN_POINT('Ctrl Pts',(-0.771721326463556,-0.290466591953583,
-4.73320810932737));
#53038=CARTESIAN_POINT('Ctrl Pts',(-0.539129493200493,-0.623910279063567,
-4.71735059875143));
#53039=CARTESIAN_POINT('Ctrl Pts',(-0.175480060095158,-0.805686908959553,
-4.70149308817548));
#53040=CARTESIAN_POINT('Ctrl Pts',(0.230827019802462,-0.791608194556446,
-4.68563557759954));
#53041=CARTESIAN_POINT('Ctrl Pts',(0.581022097712454,-0.585096546502899,
-4.66977806702359));
#53042=CARTESIAN_POINT('Ctrl Pts',(0.789975855045685,-0.236353115495945,
-4.65392055644765));
#53043=CARTESIAN_POINT('Ctrl Pts',(0.806893485991124,0.169845662367026,
-4.63806304587171));
#53044=CARTESIAN_POINT('Ctrl Pts',(0.627662464458674,0.53475646557051,-4.62220553529576));
#53045=CARTESIAN_POINT('Ctrl Pts',(0.295852262709778,0.769672713177038,
-4.60634802471982));
#53046=CARTESIAN_POINT('Ctrl Pts',(-0.107877001059769,0.81748834817516,
-4.59049051414388));
#53047=CARTESIAN_POINT('Ctrl Pts',(-0.485382322315716,0.666579813633147,
-4.57463300356793));
#53048=CARTESIAN_POINT('Ctrl Pts',(-0.744895504445808,0.353631636333951,
-4.558775492992));
#53049=CARTESIAN_POINT('Ctrl Pts',(-0.823331193733816,-0.0452812564385095,
-4.54291798241604));
#53050=CARTESIAN_POINT('Ctrl Pts',(-0.701622369529403,-0.433186677237131,
-4.5270604718401));
#53051=CARTESIAN_POINT('Ctrl Pts',(-0.409355367918847,-0.715788257458745,
-4.51120296126416));
#53052=CARTESIAN_POINT('Ctrl Pts',(-0.0175777057367246,-0.824388058514212,
-4.49534545068821));
#53053=CARTESIAN_POINT('Ctrl Pts',(0.378472940864992,-0.732586431619373,
-4.47948794011228));
#53054=CARTESIAN_POINT('Ctrl Pts',(0.682520171106463,-0.462699538353568,
-4.46363042953632));
#53055=CARTESIAN_POINT('Ctrl Pts',(0.820652799017158,-0.0803344896361682,
-4.44777291896039));
#53056=CARTESIAN_POINT('Ctrl Pts',(0.759292007444244,0.321559161261329,
-4.43191540838444));
#53057=CARTESIAN_POINT('Ctrl Pts',(0.513354060790599,0.645284631019212,
-4.4160578978085));
#53058=CARTESIAN_POINT('Ctrl Pts',(0.142624293386979,0.812147128108981,
-4.40020038723255));
#53059=CARTESIAN_POINT('Ctrl Pts',(-0.262776175223388,0.781583858901121,
-4.38434287665661));
#53060=CARTESIAN_POINT('Ctrl Pts',(-0.604298085426446,0.561024483164266,
-4.36848536608067));
#53061=CARTESIAN_POINT('Ctrl Pts',(-0.798920488805789,0.204085029647251,
-4.35262785550472));
#53062=CARTESIAN_POINT('Ctrl Pts',(-0.799332404633924,-0.202465685146767,
-4.33677034492878));
#53063=CARTESIAN_POINT('Ctrl Pts',(-0.605433699825102,-0.559798786954642,
-4.32091283435284));
#53064=CARTESIAN_POINT('Ctrl Pts',(-0.264359430400681,-0.781049766863819,
-4.3050553237769));
#53065=CARTESIAN_POINT('Ctrl Pts',(0.140978272727411,-0.812434473282982,
-4.28919781320095));
#53066=CARTESIAN_POINT('Ctrl Pts',(0.512045407677382,-0.646323562340337,
-4.27334030262501));
#53067=CARTESIAN_POINT('Ctrl Pts',(0.758638843846605,-0.323097123736636,
-4.25748279204906));
#53068=CARTESIAN_POINT('Ctrl Pts',(0.820813903214692,0.0786713610487585,
-4.24162528147312));
#53069=CARTESIAN_POINT('Ctrl Pts',(0.683456380097103,0.461315535468256,
-4.22576777089718));
#53070=CARTESIAN_POINT('Ctrl Pts',(0.379956670543603,0.731817993266919,
-4.20991026032123));
#53071=CARTESIAN_POINT('Ctrl Pts',(-0.0159071369001762,0.824421985245081,
-4.19405274974529));
#53072=CARTESIAN_POINT('Ctrl Pts',(-0.407904060397163,0.716616301985455,
-4.17819523916935));
#53073=CARTESIAN_POINT('Ctrl Pts',(-0.700743123313723,0.434607549276735,
-4.1623377285934));
#53074=CARTESIAN_POINT('Ctrl Pts',(-0.823237745783721,0.0469495545957191,
-4.14648021801746));
#53075=CARTESIAN_POINT('Ctrl Pts',(-0.745610571129455,-0.352121460549918,
-4.13062270744151));
#53076=CARTESIAN_POINT('Ctrl Pts',(-0.486732077262139,-0.665594870566085,
-4.11476519686557));
#53077=CARTESIAN_POINT('Ctrl Pts',(-0.109533330808494,-0.817268068752106,
-4.09890768628963));
#53078=CARTESIAN_POINT('Ctrl Pts',(0.294291997235545,-0.770270645372725,
-4.08305017571368));
#53079=CARTESIAN_POINT('Ctrl Pts',(0.62657754996231,-0.536027257369465,
-4.06719266513774));
#53080=CARTESIAN_POINT('Ctrl Pts',(0.806547655567773,-0.171480395549841,
-4.05133515456181));
#53081=CARTESIAN_POINT('Ctrl Pts',(0.790453177005112,0.234751830072363,
-4.03547764398585));
#53082=CARTESIAN_POINT('Ctrl Pts',(0.582206539318293,0.583917967127932,
-4.01962013340992));
#53083=CARTESIAN_POINT('Ctrl Pts',(0.232430653801666,0.791138823426793,
-4.00376262283397));
#53084=CARTESIAN_POINT('Ctrl Pts',(-0.173847062909884,0.806040846035366,
-3.98790511225803));
#53085=CARTESIAN_POINT('Ctrl Pts',(-0.537864099966638,0.625001485379737,
-3.97204760168208));
#53086=CARTESIAN_POINT('Ctrl Pts',(-0.771131143057216,0.292029804929349,
-3.95619009110614));
#53087=CARTESIAN_POINT('Ctrl Pts',(-0.816943042166037,-0.111931731945415,
-3.94033258053019));
#53088=CARTESIAN_POINT('Ctrl Pts',(-0.664163330790826,-0.488683657177766,
-3.92447506995425));
#53089=CARTESIAN_POINT('Ctrl Pts',(-0.349931402212712,-0.746640918049129,
-3.90861755937831));
#53090=CARTESIAN_POINT('Ctrl Pts',(0.0493657477302857,-0.823096391506383,
-3.89276004880236));
#53091=CARTESIAN_POINT('Ctrl Pts',(0.436662522079763,-0.699464429810938,
-3.87690253822642));
#53092=CARTESIAN_POINT('Ctrl Pts',(0.71781050878804,-0.405798866722488,
-3.86104502765048));
#53093=CARTESIAN_POINT('Ctrl Pts',(0.824465124961427,-0.0134871969711484,
-3.84518751707454));
#53094=CARTESIAN_POINT('Ctrl Pts',(0.730699579014463,0.382103090785572,
-3.82933000649859));
#53095=CARTESIAN_POINT('Ctrl Pts',(0.459307443835841,0.684807504921484,
-3.81347249592265));
#53096=CARTESIAN_POINT('Ctrl Pts',(0.0762617413083615,0.821041286155828,
-3.7976149853467));
#53097=CARTESIAN_POINT('Ctrl Pts',(-0.325322514389958,0.757687210127501,
-3.78175747477077));
#53098=CARTESIAN_POINT('Ctrl Pts',(-0.647823751169212,0.510146091017909,
-3.76589996419481));
#53099=CARTESIAN_POINT('Ctrl Pts',(-0.812844777683873,0.138592980168027,
-3.75004245361888));
#53100=CARTESIAN_POINT('Ctrl Pts',(-0.780270445474654,-0.266650855386938,
-3.73418494304293));
#53101=CARTESIAN_POINT('Ctrl Pts',(-0.558019285895612,-0.607074232139984,
-3.71832743246699));
#53102=CARTESIAN_POINT('Ctrl Pts',(-0.200118585348163,-0.799923245416739,
-3.70246992189104));
#53103=CARTESIAN_POINT('Ctrl Pts',(0.206429169033917,-0.798318009900671,
-3.6866124113151));
#53104=CARTESIAN_POINT('Ctrl Pts',(0.56279582263738,-0.602648744113612,
-3.67075490073916));
#53105=CARTESIAN_POINT('Ctrl Pts',(0.782351801539573,-0.26048091175283,
-3.65489739016321));
#53106=CARTESIAN_POINT('Ctrl Pts',(0.811724993865988,0.145007520815514,
-3.63903987958727));
#53107=CARTESIAN_POINT('Ctrl Pts',(0.64377503698658,0.515245910719075,-3.62318236901133));
#53108=CARTESIAN_POINT('Ctrl Pts',(0.319329076364232,0.760232587928305,
-3.60732485843538));
#53109=CARTESIAN_POINT('Ctrl Pts',(-0.0827429515313146,0.820413463280368,
-3.59146734785944));
#53110=CARTESIAN_POINT('Ctrl Pts',(-0.464700901513617,0.681159099544468,
-3.57560983728349));
#53111=CARTESIAN_POINT('Ctrl Pts',(-0.733694182404323,0.376320997907176,
-3.55975232670756));
#53112=CARTESIAN_POINT('Ctrl Pts',(-0.824332912529633,-0.0199974018365713,
-3.54389481613161));
#53113=CARTESIAN_POINT('Ctrl Pts',(-0.714583620204558,-0.411454610492029,
-3.52803730555567));
#53114=CARTESIAN_POINT('Ctrl Pts',(-0.431125385349447,-0.702890851318391,
-3.51217979497972));
#53115=CARTESIAN_POINT('Ctrl Pts',(-0.0428643916996818,-0.823460558062143,
-3.49632228440378));
#53116=CARTESIAN_POINT('Ctrl Pts',(0.35581655553398,-0.743854303992209,
-3.48046477382783));
#53117=CARTESIAN_POINT('Ctrl Pts',(0.66800165280848,-0.483423663679116,
-3.4646072632519));
#53118=CARTESIAN_POINT('Ctrl Pts',(0.817801470828383,-0.105477016789133,
-3.44874975267595));
#53119=CARTESIAN_POINT('Ctrl Pts',(0.768801001967315,0.29811015771666,-3.43289224210001));
#53120=CARTESIAN_POINT('Ctrl Pts',(0.532911825764281,0.629229395944262,
-3.41703473152406));
#53121=CARTESIAN_POINT('Ctrl Pts',(0.167476509546501,0.807388546803781,
-3.40117722094812));
#53122=CARTESIAN_POINT('Ctrl Pts',(-0.238670861285152,0.789278700291097,
-3.38531971037218));
#53123=CARTESIAN_POINT('Ctrl Pts',(-0.586799461808706,0.579302199530446,
-3.36946219979623));
#53124=CARTESIAN_POINT('Ctrl Pts',(-0.792282315766162,0.228502470192357,
-3.35360468922029));
#53125=CARTESIAN_POINT('Ctrl Pts',(-0.805168363183897,-0.177844183732743,
-3.33774717864434));
#53126=CARTESIAN_POINT('Ctrl Pts',(-0.622325120183137,-0.540958493369726,
-3.3218896680684));
#53127=CARTESIAN_POINT('Ctrl Pts',(-0.288200158038096,-0.772570589439319,
-3.30603215749246));
#53128=CARTESIAN_POINT('Ctrl Pts',(0.115983707325935,-0.816377624873889,
-3.29017464691651));
#53129=CARTESIAN_POINT('Ctrl Pts',(0.491972961757609,-0.661730497755124,
-3.27431713634057));
#53130=CARTESIAN_POINT('Ctrl Pts',(0.748367951048111,-0.346222553574797,
-3.25845962576463));
#53131=CARTESIAN_POINT('Ctrl Pts',(0.822841326514434,0.0534490237494227,
-3.24260211518868));
#53132=CARTESIAN_POINT('Ctrl Pts',(0.697289270866175,0.440127617282441,
-3.22674460461274));
#53133=CARTESIAN_POINT('Ctrl Pts',(0.402232375679288,0.71981508925223,-3.2108870940368));
#53134=CARTESIAN_POINT('Ctrl Pts',(0.00939635618139049,0.824521894949015,
-3.19502958346085));
#53135=CARTESIAN_POINT('Ctrl Pts',(-0.385723834195541,0.72879473824479,
-3.17917207288491));
#53136=CARTESIAN_POINT('Ctrl Pts',(-0.687077980330429,0.455904042211581,
-3.16331456230897));
#53137=CARTESIAN_POINT('Ctrl Pts',(-0.821409561122009,0.0721871155896124,
-3.14745705173302));
#53138=CARTESIAN_POINT('Ctrl Pts',(-0.75606376027179,-0.329077858816847,
-3.13159954115708));
#53139=CARTESIAN_POINT('Ctrl Pts',(-0.506925562606628,-0.650346923369176,
-3.11574203058114));
#53140=CARTESIAN_POINT('Ctrl Pts',(-0.134558255104558,-0.813522416865705,
-3.09988452000519));
#53141=CARTESIAN_POINT('Ctrl Pts',(0.270518971211785,-0.778937823561237,
-3.08402700942925));
#53142=CARTESIAN_POINT('Ctrl Pts',(0.609835434064138,-0.555000351458992,
-3.06816949885331));
#53143=CARTESIAN_POINT('Ctrl Pts',(0.800906309733423,-0.196147214583821,
-3.05231198827736));
#53144=CARTESIAN_POINT('Ctrl Pts',(0.797283962390398,0.210387571103583,
-3.03645447770142));
#53145=CARTESIAN_POINT('Ctrl Pts',(0.599848952558207,0.565779003564664,
-3.02059696712548));
#53146=CARTESIAN_POINT('Ctrl Pts',(0.256595980656287,0.783634576490111,
-3.00473945654953));
#53147=CARTESIAN_POINT('Ctrl Pts',(-0.149033199147652,0.810995531622473,
-2.98888194597359));
#53148=CARTESIAN_POINT('Ctrl Pts',(-0.51843372957618,0.641210663352952,
-2.97302443539765));
#53149=CARTESIAN_POINT('Ctrl Pts',(-0.761807616809609,0.315553167834938,
-2.9571669248217));
#53150=CARTESIAN_POINT('Ctrl Pts',(-0.819992826629131,-0.0868125050702396,
-2.94130941424576));
#53151=CARTESIAN_POINT('Ctrl Pts',(-0.678845050401212,-0.468074827677772,
-2.92545190366981));
#53152=CARTESIAN_POINT('Ctrl Pts',(-0.372676061102124,-0.735552309656633,
-2.90959439309387));
#53153=CARTESIAN_POINT('Ctrl Pts',(0.0240871744823412,-0.824223546609326,
-2.89373688251793));
#53154=CARTESIAN_POINT('Ctrl Pts',(0.414995031508496,-0.71253334699722,
-2.87787937194199));
#53155=CARTESIAN_POINT('Ctrl Pts',(0.705021275746043,-0.427632608093937,
-2.86202186136604));
#53156=CARTESIAN_POINT('Ctrl Pts',(0.823663098611094,-0.0387781735796382,
-2.8461643507901));
#53157=CARTESIAN_POINT('Ctrl Pts',(0.742079724850744,0.359502891122233,
-2.83030684021416));
#53158=CARTESIAN_POINT('Ctrl Pts',(0.480103349303,0.670391990366713,-2.81444932963821));
#53159=CARTESIAN_POINT('Ctrl Pts',(0.101418106165091,0.818314740489066,
-2.79859181906227));
#53160=CARTESIAN_POINT('Ctrl Pts',(-0.301920979402475,0.767312432426616,
-2.78273430848632));
#53161=CARTESIAN_POINT('Ctrl Pts',(-0.631865751727002,0.529783275079793,
-2.76687679791039));
#53162=CARTESIAN_POINT('Ctrl Pts',(-0.80820956196675,0.163468500651699,
-2.75101928733443));
#53163=CARTESIAN_POINT('Ctrl Pts',(-0.788084793327346,-0.242584016963188,
-2.7351617767585));
#53164=CARTESIAN_POINT('Ctrl Pts',(-0.57638359863761,-0.589666510818917,
-2.71930426618255));
#53165=CARTESIAN_POINT('Ctrl Pts',(-0.224568661370999,-0.793406303913598,
-2.70344675560661));
#53166=CARTESIAN_POINT('Ctrl Pts',(0.181836926435539,-0.804276058915269,
-2.68758924503066));
#53167=CARTESIAN_POINT('Ctrl Pts',(0.544039569602812,-0.619633434754925,
-2.67173173445472));
#53168=CARTESIAN_POINT('Ctrl Pts',(0.773991016887443,-0.284363416313251,
-2.65587422387878));
#53169=CARTESIAN_POINT('Ctrl Pts',(0.815792110218004,0.12003282745089,-2.64001671330283));
#53170=CARTESIAN_POINT('Ctrl Pts',(0.659281374416868,0.495250155080043,
-2.62415920272689));
#53171=CARTESIAN_POINT('Ctrl Pts',(0.342505181723618,0.75007656092713,-2.60830169215095));
#53172=CARTESIAN_POINT('Ctrl Pts',(-0.0575309839749372,0.822566005037088,
-2.592444181575));
#53173=CARTESIAN_POINT('Ctrl Pts',(-0.443581877542379,0.695096946242594,
-2.57658667099907));
#53174=CARTESIAN_POINT('Ctrl Pts',(-0.721801949503084,0.398655982588181,
-2.56072916042311));
#53175=CARTESIAN_POINT('Ctrl Pts',(-0.824558367079424,0.00530528407468725,
-2.54487164984718));
#53176=CARTESIAN_POINT('Ctrl Pts',(-0.72687195620322,-0.389335081960394,
-2.52901413927123));
#53177=CARTESIAN_POINT('Ctrl Pts',(-0.452489417264832,-0.689331541439337,
-2.51315662869529));
#53178=CARTESIAN_POINT('Ctrl Pts',(-0.0681107127879656,-0.821757614849608,
-2.49729911811934));
#53179=CARTESIAN_POINT('Ctrl Pts',(0.332825102093949,-0.75442169784276,
-2.4814416075434));
#53180=CARTESIAN_POINT('Ctrl Pts',(0.652854085504351,-0.503692554838839,
-2.46558409696745));
#53181=CARTESIAN_POINT('Ctrl Pts',(0.814180028972541,-0.130520217522318,
-2.44972658639152));
#53182=CARTESIAN_POINT('Ctrl Pts',(0.777586025966992,0.274380427473716,
-2.43386907581557));
#53183=CARTESIAN_POINT('Ctrl Pts',(0.551967754173711,0.61258162322439,-2.41801156523963));
#53184=CARTESIAN_POINT('Ctrl Pts',(0.192171015120368,0.801869657555022,
-2.40215405466368));
#53185=CARTESIAN_POINT('Ctrl Pts',(-0.214340793908872,0.796230287559016,
-2.38629654408774));
#53186=CARTESIAN_POINT('Ctrl Pts',(-0.568748256297336,0.597034394083407,
-2.3704390335118));
#53187=CARTESIAN_POINT('Ctrl Pts',(-0.784898060136431,0.252704732749246,
-2.35458152293585));
#53188=CARTESIAN_POINT('Ctrl Pts',(-0.810246104510137,-0.153055208620778,
-2.33872401235991));
#53189=CARTESIAN_POINT('Ctrl Pts',(-0.638630504568503,-0.521608785771845,
-2.32286650178397));
#53190=CARTESIAN_POINT('Ctrl Pts',(-0.311769491103034,-0.763363891716889,
-2.30700899120802));
#53191=CARTESIAN_POINT('Ctrl Pts',(0.0908799214823766,-0.819552003616096,
-2.29115148063208));
#53192=CARTESIAN_POINT('Ctrl Pts',(0.471437230902318,-0.67651428963397,
-2.27529397005613));
#53193=CARTESIAN_POINT('Ctrl Pts',(0.737392329280969,-0.369021949858524,
-2.2594364594802));
#53194=CARTESIAN_POINT('Ctrl Pts',(0.824093890176505,0.0281763541565548,
-2.24357894890425));
#53195=CARTESIAN_POINT('Ctrl Pts',(0.710465532836513,0.418525236289438,
-2.22772143832831));
#53196=CARTESIAN_POINT('Ctrl Pts',(0.424129303494443,0.707134344150474,
-2.21186392775236));
#53197=CARTESIAN_POINT('Ctrl Pts',(0.0346910008289892,0.823845362444482,
-2.19600641717642));
#53198=CARTESIAN_POINT('Ctrl Pts',(-0.363180376565469,0.740286877391164,
-2.18014890660048));
#53199=CARTESIAN_POINT('Ctrl Pts',(-0.672765824396101,0.476771215872387,
-2.16429139602453));
#53200=CARTESIAN_POINT('Ctrl Pts',(-0.818807865098622,0.0973566988575322,
-2.14843388544859));
#53201=CARTESIAN_POINT('Ctrl Pts',(-0.765804973395835,-0.305724368479202,
-2.13257637487265));
#53202=CARTESIAN_POINT('Ctrl Pts',(-0.52664168233383,-0.634486552409421,
-2.1167188642967));
#53203=CARTESIAN_POINT('Ctrl Pts',(-0.15945646753355,-0.809010680845144,
-2.10086135372076));
#53204=CARTESIAN_POINT('Ctrl Pts',(0.246491200773431,-0.786871485505144,
-2.08500384314482));
#53205=CARTESIAN_POINT('Ctrl Pts',(0.592519043578318,-0.57345080848913,
-2.06914633256887));
#53206=CARTESIAN_POINT('Ctrl Pts',(0.794510760199069,-0.220629324179034,
-2.05328882199293));
#53207=CARTESIAN_POINT('Ctrl Pts',(0.803363955195986,0.185825192726024,
-2.03743131141698));
#53208=CARTESIAN_POINT('Ctrl Pts',(0.616926495358278,0.547107252816805,
-2.02157380084104));
#53209=CARTESIAN_POINT('Ctrl Pts',(0.280519674206675,0.775392390433891,
-2.0057162902651));
#53210=CARTESIAN_POINT('Ctrl Pts',(-0.124078992640135,0.815186512612425,
-1.98985877968915));
#53211=CARTESIAN_POINT('Ctrl Pts',(-0.498515156467999,0.656816021067916,
-1.97400126911321));
#53212=CARTESIAN_POINT('Ctrl Pts',(-0.751766705624085,0.338779378172446,
-1.95814375853727));
#53213=CARTESIAN_POINT('Ctrl Pts',(-0.822270433852137,-0.0616115279182409,
-1.94228624796132));
#53214=CARTESIAN_POINT('Ctrl Pts',(-0.692887509910239,-0.447025217823546,
-1.92642873738538));
#53215=CARTESIAN_POINT('Ctrl Pts',(-0.39506977549183,-0.723771040628618,
-1.91057122680944));
#53216=CARTESIAN_POINT('Ctrl Pts',(-0.00121408136393792,-0.824574540454796,
-1.89471371623349));
#53217=CARTESIAN_POINT('Ctrl Pts',(0.392936745179409,-0.72493128022428,
-1.87885620565755));
#53218=CARTESIAN_POINT('Ctrl Pts',(0.691568132770651,-0.449063653055908,
-1.86299869508161));
#53219=CARTESIAN_POINT('Ctrl Pts',(0.822085438770328,-0.0640326332552135,
-1.84714118450567));
#53220=CARTESIAN_POINT('Ctrl Pts',(0.752761063264271,0.336564151972617,
-1.83128367392972));
#53221=CARTESIAN_POINT('Ctrl Pts',(0.500447147303881,0.655345175854074,
-1.81542616335378));
#53222=CARTESIAN_POINT('Ctrl Pts',(0.126478966828661,0.814817597815459,
-1.79956865277783));
#53223=CARTESIAN_POINT('Ctrl Pts',(-0.278235129112421,0.776215085970115,
-1.78371114220189));
#53224=CARTESIAN_POINT('Ctrl Pts',(-0.615312732015794,0.54892156869544,
-1.76785363162595));
#53225=CARTESIAN_POINT('Ctrl Pts',(-0.802813265166102,0.1881900848428,-1.75199612105));
#53226=CARTESIAN_POINT('Ctrl Pts',(-0.795157011345605,-0.218288740130424,
-1.73613861047406));
#53227=CARTESIAN_POINT('Ctrl Pts',(-0.594205137977248,-0.571703507739143,
-1.72028109989812));
#53228=CARTESIAN_POINT('Ctrl Pts',(-0.248807263825392,-0.786142221374429,
-1.70442358932217));
#53229=CARTESIAN_POINT('Ctrl Pts',(0.157073450222133,-0.809476730978177,
-1.68856607874623));
#53230=CARTESIAN_POINT('Ctrl Pts',(0.52477100114339,-0.636034624150891,
-1.67270856817029));
#53231=CARTESIAN_POINT('Ctrl Pts',(0.76490137433819,-0.307978139314054,
-1.65685105759434));
#53232=CARTESIAN_POINT('Ctrl Pts',(0.819091005093328,0.0949451006371796,
-1.6409935470184));
#53233=CARTESIAN_POINT('Ctrl Pts',(0.674166874620773,0.474788028412531,
-1.62513603644245));
#53234=CARTESIAN_POINT('Ctrl Pts',(0.365358754132285,0.739214195980236,
-1.60927852586651));
#53235=CARTESIAN_POINT('Ctrl Pts',(-0.0322648401929043,0.823943946423011,
-1.59342101529057));
#53236=CARTESIAN_POINT('Ctrl Pts',(-0.422045137929226,0.708380228627325,
-1.57756350471462));
#53237=CARTESIAN_POINT('Ctrl Pts',(-0.709230004512728,0.420615557794379,
-1.56170599413868));
#53238=CARTESIAN_POINT('Ctrl Pts',(-0.824007345075392,0.030602974064658,
-1.54584848356274));
#53239=CARTESIAN_POINT('Ctrl Pts',(-0.738475805749304,-0.366848921332357,
-1.52999097298679));
#53240=CARTESIAN_POINT('Ctrl Pts',(-0.473427345416823,-0.675123096458254,
-1.51413346241085));
#53241=CARTESIAN_POINT('Ctrl Pts',(-0.0932928948490484,-0.819280832517449,
-1.49827595183491));
#53242=CARTESIAN_POINT('Ctrl Pts',(0.309520231316071,-0.764278661985173,
-1.48241844125897));
#53243=CARTESIAN_POINT('Ctrl Pts',(0.637091733473383,-0.523487124865244,
-1.46656093068302));
#53244=CARTESIAN_POINT('Ctrl Pts',(0.809791883717243,-0.155440508959154,
-1.45070342010708));
#53245=CARTESIAN_POINT('Ctrl Pts',(0.785638806693365,0.250392316529934,
-1.43484590953113));
#53246=CARTESIAN_POINT('Ctrl Pts',(0.57050390128361,0.595356989864048,-1.41898839895519));
#53247=CARTESIAN_POINT('Ctrl Pts',(0.216684555593979,0.795595657433373,
-1.40313088837925));
#53248=CARTESIAN_POINT('Ctrl Pts',(-0.189808884422145,0.802432074479965,
-1.3872733778033));
#53249=CARTESIAN_POINT('Ctrl Pts',(-0.55016146749232,0.61420436863189,-1.37141586722736));
#53250=CARTESIAN_POINT('Ctrl Pts',(-0.776774675580029,0.276669026342562,
-1.35555835665142));
#53251=CARTESIAN_POINT('Ctrl Pts',(-0.81456084696559,-0.128122103286285,
-1.33970084607547));
#53252=CARTESIAN_POINT('Ctrl Pts',(-0.654334498399659,-0.501767885544569,
-1.32384333549953));
#53253=CARTESIAN_POINT('Ctrl Pts',(-0.335045234642093,-0.753438343531457,
-1.30798582492359));
#53254=CARTESIAN_POINT('Ctrl Pts',(0.0656905551256053,-0.821954620235868,
-1.29212831434764));
#53255=CARTESIAN_POINT('Ctrl Pts',(0.450457553358707,-0.690661016260428,
-1.2762708037717));
#53256=CARTESIAN_POINT('Ctrl Pts',(0.72572231415428,-0.391473842674518,
-1.26041329319576));
#53257=CARTESIAN_POINT('Ctrl Pts',(0.824570414676984,0.00287715123474536,
-1.24455578261981));
#53258=CARTESIAN_POINT('Ctrl Pts',(0.722972758082991,0.396528735187848,
-1.22869827204387));
#53259=CARTESIAN_POINT('Ctrl Pts',(0.445626833919317,0.693787699264584,
-1.21284076146793));
#53260=CARTESIAN_POINT('Ctrl Pts',(0.0599529773843778,0.822393024813896,
-1.19698325089198));
#53261=CARTESIAN_POINT('Ctrl Pts',(-0.340294916405972,0.751081897417354,
-1.18112574031604));
#53262=CARTESIAN_POINT('Ctrl Pts',(-0.657820133093386,0.497189419896282,
-1.1652682297401));
#53263=CARTESIAN_POINT('Ctrl Pts',(-0.815435107698969,0.122434602509957,
-1.14941071916415));
#53264=CARTESIAN_POINT('Ctrl Pts',(-0.774825037320025,-0.282082981233933,
-1.13355320858821));
#53265=CARTESIAN_POINT('Ctrl Pts',(-0.545861870014327,-0.618028693204662,
-1.11769569801227));
#53266=CARTESIAN_POINT('Ctrl Pts',(-0.184204521752573,-0.803737109337193,
-1.10183818743632));
#53267=CARTESIAN_POINT('Ctrl Pts',(0.222231312578776,-0.794064160171781,
-1.08598067686038));
#53268=CARTESIAN_POINT('Ctrl Pts',(0.574644685138513,-0.591361253889582,
-1.07012316628444));
#53269=CARTESIAN_POINT('Ctrl Pts',(0.787367029575686,-0.24490366983155,
-1.05426565570849));
#53270=CARTESIAN_POINT('Ctrl Pts',(0.80868742996682,0.161087825031754,-1.03840814513255));
#53271=CARTESIAN_POINT('Ctrl Pts',(0.63342308600479,0.527920297844257,-1.02255063455661));
#53272=CARTESIAN_POINT('Ctrl Pts',(0.30417920580247,0.766420026824182,-1.00669312398066));
#53273=CARTESIAN_POINT('Ctrl Pts',(-0.0990079424591542,0.818609842409561,
-0.990835613404719));
#53274=CARTESIAN_POINT('Ctrl Pts',(-0.478127137719371,0.671802863149659,
-0.974978102828773));
#53275=CARTESIAN_POINT('Ctrl Pts',(-0.741017864904195,0.361686564102989,
-0.959120592252833));
#53276=CARTESIAN_POINT('Ctrl Pts',(-0.823773719040125,-0.0363525319421145,
-0.943263081676887));
#53277=CARTESIAN_POINT('Ctrl Pts',(-0.706277485705126,-0.42555464977585,
-0.927405571100945));
#53278=CARTESIAN_POINT('Ctrl Pts',(-0.41709145749421,-0.711308205242394,
-0.911548060525001));
#53279=CARTESIAN_POINT('Ctrl Pts',(-0.0265141939245934,-0.824149042516177,
-0.895690549949058));
#53280=CARTESIAN_POINT('Ctrl Pts',(0.37050843511164,-0.736646554509639,
-0.879833039373114));
#53281=CARTESIAN_POINT('Ctrl Pts',(0.677463748522479,-0.470071820254814,
-0.863975528797172));
#53282=CARTESIAN_POINT('Ctrl Pts',(0.819733631102158,-0.0892267941812924,
-0.848118018221227));
#53283=CARTESIAN_POINT('Ctrl Pts',(0.762733535768966,0.313308474467536,
-0.832260507645284));
#53284=CARTESIAN_POINT('Ctrl Pts',(0.520319680332095,0.63968123078523,-0.81640299706934));
#53285=CARTESIAN_POINT('Ctrl Pts',(0.151420723792317,0.810553151351601,
-0.800545486493398));
#53286=CARTESIAN_POINT('Ctrl Pts',(-0.254287268196057,0.784386787237767,
-0.784687975917453));
#53287=CARTESIAN_POINT('Ctrl Pts',(-0.598180279812305,0.567542949567232,
-0.768830465341511));
#53288=CARTESIAN_POINT('Ctrl Pts',(-0.796660968908797,0.212734452727095,
-0.752972954765567));
#53289=CARTESIAN_POINT('Ctrl Pts',(-0.801480439708001,-0.193787903454448,
-0.737115444189623));
#53290=CARTESIAN_POINT('Ctrl Pts',(-0.611467121588348,-0.553202138441512,
-0.72125793361368));
#53291=CARTESIAN_POINT('Ctrl Pts',(-0.272811567515137,-0.77813783829713,
-0.705400423037737));
#53292=CARTESIAN_POINT('Ctrl Pts',(0.132162059857106,-0.813915128679966,
-0.689542912461794));
#53293=CARTESIAN_POINT('Ctrl Pts',(0.505008262234922,-0.651836867501574,
-0.67368540188585));
#53294=CARTESIAN_POINT('Ctrl Pts',(0.755091433497301,-0.331302843058724,
-0.657827891309907));
#53295=CARTESIAN_POINT('Ctrl Pts',(0.821618571962899,0.0697679651806149,
-0.641970380733963));
#53296=CARTESIAN_POINT('Ctrl Pts',(0.688417520104387,0.453878799651551,
-0.62611287015802));
#53297=CARTESIAN_POINT('Ctrl Pts',(0.387868272659935,0.727655722044151,
-0.610255359582077));
#53298=CARTESIAN_POINT('Ctrl Pts',(-0.00696831300448354,0.824545989847542,
-0.594397849006133));
#53299=CARTESIAN_POINT('Ctrl Pts',(-0.400110963559091,0.720996437993744,
-0.578540338430189));
#53300=CARTESIAN_POINT('Ctrl Pts',(-0.695990186280356,0.442179044461741,
-0.562682827854247));
#53301=CARTESIAN_POINT('Ctrl Pts',(-0.822680365408402,0.0558718456073918,
-0.546825317278302));
#53302=CARTESIAN_POINT('Ctrl Pts',(-0.749384241638951,-0.344017303551129,
-0.530967806702359));
#53303=CARTESIAN_POINT('Ctrl Pts',(-0.493919452814545,-0.660278896294274,
-0.515110296126415));
#53304=CARTESIAN_POINT('Ctrl Pts',(-0.118387224128064,-0.816032543421702,
-0.499252785550473));
#53305=CARTESIAN_POINT('Ctrl Pts',(0.285923889110438,-0.773415914235931,
-0.483395274974528));
#53306=CARTESIAN_POINT('Ctrl Pts',(0.620729439934895,-0.542788733454466,
-0.467537764398586));
#53307=CARTESIAN_POINT('Ctrl Pts',(0.804641167316146,-0.180214423962784,
-0.451680253822641));
#53308=CARTESIAN_POINT('Ctrl Pts',(0.79295176095903,0.226168414191993,-0.435822743246698));
#53309=CARTESIAN_POINT('Ctrl Pts',(0.588502811795286,0.577571716099595,
-0.419965232670754));
#53310=CARTESIAN_POINT('Ctrl Pts',(0.240994046933947,0.788572454570089,
-0.404107722094812));
#53311=CARTESIAN_POINT('Ctrl Pts',(-0.165098234358834,0.80787822094225,
-0.388250211518868));
#53312=CARTESIAN_POINT('Ctrl Pts',(-0.531056598084034,0.630795954351229,
-0.372392700942924));
#53313=CARTESIAN_POINT('Ctrl Pts',(-0.767919812300705,0.300372784224499,
-0.356535190366982));
#53314=CARTESIAN_POINT('Ctrl Pts',(-0.818108526410274,-0.10306834719425,
-0.340677679791037));
#53315=CARTESIAN_POINT('Ctrl Pts',(-0.669422315370429,-0.481454476105894,
-0.324820169215095));
#53316=CARTESIAN_POINT('Ctrl Pts',(-0.358005466355305,-0.742803292658146,
-0.308962658639151));
#53317=CARTESIAN_POINT('Ctrl Pts',(0.0404393213179984,-0.823583210249897,
-0.293105148063208));
#53318=CARTESIAN_POINT('Ctrl Pts',(0.42905370000224,-0.704157359680949,
-0.277247637487263));
#53319=CARTESIAN_POINT('Ctrl Pts',(0.713368866712798,-0.413557081834078,
-0.261390126911321));
#53320=CARTESIAN_POINT('Ctrl Pts',(0.824270506897614,-0.022424775748895,
-0.245532616335377));
#53321=CARTESIAN_POINT('Ctrl Pts',(0.734799060031862,0.374158856504314,
-0.229675105759433));
#53322=CARTESIAN_POINT('Ctrl Pts',(0.466704935323213,0.679787666910914,
-0.213817595183491));
#53323=CARTESIAN_POINT('Ctrl Pts',(0.0851580820844976,0.820166359232661,
-0.197960084607547));
#53324=CARTESIAN_POINT('Ctrl Pts',(-0.317088194075989,0.761169418782602,
-0.182102574031603));
#53325=CARTESIAN_POINT('Ctrl Pts',(-0.642256564426576,0.517139844854084,
-0.16624506345566));
#53326=CARTESIAN_POINT('Ctrl Pts',(-0.811291370158351,0.147396393859673,
-0.150387552879717));
#53327=CARTESIAN_POINT('Ctrl Pts',(-0.783121507604153,-0.258174361913263,
-0.134530042303774));
#53328=CARTESIAN_POINT('Ctrl Pts',(-0.564556177128614,-0.600991981115412,
-0.11867253172783));
#53329=CARTESIAN_POINT('Ctrl Pts',(-0.208802571875496,-0.797700379488531,
-0.102815021151887));
#53330=CARTESIAN_POINT('Ctrl Pts',(0.197811256787455,-0.800523053928257,
-0.0869575105759431));
#53331=CARTESIAN_POINT('Ctrl Pts',(0.436668678781749,-0.672619994853352,
-0.0763858368586473));
#53332=CARTESIAN_POINT('Ctrl Pts',(0.533647856309019,-0.584002718706676,
-0.0710999999999995));
#53333=CARTESIAN_POINT('Ctrl Pts',(0.437168237015814,-0.613060138694073,
-5.8529325805302));
#53334=CARTESIAN_POINT('Ctrl Pts',(0.538972674085852,-0.540464216262873,
-5.84764674367155));
#53335=CARTESIAN_POINT('Ctrl Pts',(0.705617707738108,-0.34365284496799,
-5.83707506995425));
#53336=CARTESIAN_POINT('Ctrl Pts',(0.78403213362876,0.035343353160595,-5.82121755937831));
#53337=CARTESIAN_POINT('Ctrl Pts',(0.671861149737833,0.405647193175061,
-5.80536004880237));
#53338=CARTESIAN_POINT('Ctrl Pts',(0.39636423752786,0.677391306117648,-5.78950253822642));
#53339=CARTESIAN_POINT('Ctrl Pts',(0.0245158897253287,0.784442450324301,
-5.77364502765049));
#53340=CARTESIAN_POINT('Ctrl Pts',(-0.353292660905754,0.700815442703755,
-5.75778751707453));
#53341=CARTESIAN_POINT('Ctrl Pts',(-0.645218587577802,0.446819837923923,
-5.74193000649859));
#53342=CARTESIAN_POINT('Ctrl Pts',(-0.780297754981346,0.0842096578098633,
-5.72607249592265));
#53343=CARTESIAN_POINT('Ctrl Pts',(-0.725693375032965,-0.298872866094613,
-5.71021498534671));
#53344=CARTESIAN_POINT('Ctrl Pts',(-0.494679411256276,-0.609301164450066,
-5.69435747477076));
#53345=CARTESIAN_POINT('Ctrl Pts',(-0.143413247169386,-0.771614203049557,
-5.67849996419482));
#53346=CARTESIAN_POINT('Ctrl Pts',(0.242715394896773,-0.746354439128878,
-5.66264245361887));
#53347=CARTESIAN_POINT('Ctrl Pts',(0.569842081970103,-0.539662646474474,
-5.64678494304293));
#53348=CARTESIAN_POINT('Ctrl Pts',(0.758445208316514,-0.201783588651147,
-5.63092743246699));
#53349=CARTESIAN_POINT('Ctrl Pts',(0.762677030403281,0.185147239587262,
-5.61506992189104));
#53350=CARTESIAN_POINT('Ctrl Pts',(0.581508827592089,0.527070431254392,
-5.5992124113151));
#53351=CARTESIAN_POINT('Ctrl Pts',(0.258980984868453,0.740867466012043,
-5.58335490073916));
#53352=CARTESIAN_POINT('Ctrl Pts',(-0.126502839331452,0.774566192508729,
-5.56749739016321));
#53353=CARTESIAN_POINT('Ctrl Pts',(-0.481234944771481,0.619974742833006,
-5.55163987958727));
#53354=CARTESIAN_POINT('Ctrl Pts',(-0.718983101847058,0.314672930995483,
-5.53578236901132));
#53355=CARTESIAN_POINT('Ctrl Pts',(-0.781952841385118,-0.0671230810142253,
-5.51992485843539));
#53356=CARTESIAN_POINT('Ctrl Pts',(-0.654836778037186,-0.432602066861879,
-5.50406734785944));
#53357=CARTESIAN_POINT('Ctrl Pts',(-0.368535699764102,-0.692919325877319,
-5.4882098372835));
#53358=CARTESIAN_POINT('Ctrl Pts',(0.00735313965826202,-0.784794040162126,
-5.47235232670755));
#53359=CARTESIAN_POINT('Ctrl Pts',(0.381454496024887,-0.685892281353231,
-5.45649481613161));
#53360=CARTESIAN_POINT('Ctrl Pts',(0.662827646405622,-0.420256190090367,
-5.44063730555566));
#53361=CARTESIAN_POINT('Ctrl Pts',(0.783073272615713,-0.052459545043391,
-5.42477979497973));
#53362=CARTESIAN_POINT('Ctrl Pts',(0.712960729027783,0.328089550299248,
-5.40892228440377));
#53363=CARTESIAN_POINT('Ctrl Pts',(0.469533753366363,0.628882984823358,
-5.39306477382785));
#53364=CARTESIAN_POINT('Ctrl Pts',(0.111967285176232,0.776800541452915,
-5.37720726325188));
#53365=CARTESIAN_POINT('Ctrl Pts',(-0.272817437331468,0.735884773615265,
-5.36134975267595));
#53366=CARTESIAN_POINT('Ctrl Pts',(-0.591282659639843,0.516081941711108,
-5.34549224210001));
#53367=CARTESIAN_POINT('Ctrl Pts',(-0.766012309737663,0.170824165390574,
-5.32963473152406));
#53368=CARTESIAN_POINT('Ctrl Pts',(-0.754531158849833,-0.21595945099891,
-5.31377722094812));
#53369=CARTESIAN_POINT('Ctrl Pts',(-0.559630172964593,-0.550245239560189,
-5.29791971037218));
#53370=CARTESIAN_POINT('Ctrl Pts',(-0.2286880537467,-0.750771288892008,
-5.28206219979623));
#53371=CARTESIAN_POINT('Ctrl Pts',(0.157846103774871,-0.768791494277949,
-5.2662046892203));
#53372=CARTESIAN_POINT('Ctrl Pts',(0.506009272941894,-0.5999253035569,-5.25034717864434));
#53373=CARTESIAN_POINT('Ctrl Pts',(0.73116607416563,-0.28522259051528,-5.2344896680684));
#53374=CARTESIAN_POINT('Ctrl Pts',(0.778582885322433,0.0988152054798314,
-5.21863215749246));
#53375=CARTESIAN_POINT('Ctrl Pts',(0.636733100020407,0.458831901124396,
-5.20277464691652));
#53376=CARTESIAN_POINT('Ctrl Pts',(0.340099143417682,0.707310629637068,
-5.18691713634057));
#53377=CARTESIAN_POINT('Ctrl Pts',(-0.039209899610264,0.783848415143884,
-5.17105962576463));
#53378=CARTESIAN_POINT('Ctrl Pts',(-0.408987363680301,0.669839600576782,
-5.15520211518868));
#53379=CARTESIAN_POINT('Ctrl Pts',(-0.679343625746411,0.392998717947966,
-5.13934460461275));
#53380=CARTESIAN_POINT('Ctrl Pts',(-0.784557475495335,0.0206233313364565,
-5.12348709403679));
#53381=CARTESIAN_POINT('Ctrl Pts',(-0.699052358885477,-0.35676540427524,
-5.10762958346086));
#53382=CARTESIAN_POINT('Ctrl Pts',(-0.443613811671148,-0.647427633211327,
-5.09177207288491));
#53383=CARTESIAN_POINT('Ctrl Pts',(-0.0803366799465044,-0.780705944646382,
-5.07591456230896));
#53384=CARTESIAN_POINT('Ctrl Pts',(0.30246958640326,-0.724201562724126,
-5.06005705173303));
#53385=CARTESIAN_POINT('Ctrl Pts',(0.611748178012079,-0.491650201718588,
-5.04419954115708));
#53386=CARTESIAN_POINT('Ctrl Pts',(0.772316211342588,-0.139583035675748,
-5.02834203058114));
#53387=CARTESIAN_POINT('Ctrl Pts',(0.745141021098056,0.24641552878821,-5.0124845200052));
#53388=CARTESIAN_POINT('Ctrl Pts',(0.536828655090044,0.572512662938769,
-4.99662700942925));
#53389=CARTESIAN_POINT('Ctrl Pts',(0.19801800258504,0.759437044660883,-4.98076949885331));
#53390=CARTESIAN_POINT('Ctrl Pts',(-0.188929070708771,0.761749014040809,
-4.96491198827737));
#53391=CARTESIAN_POINT('Ctrl Pts',(-0.529949161969875,0.578886551820349,
-4.94905447770142));
#53392=CARTESIAN_POINT('Ctrl Pts',(-0.742143310517495,0.255301901295619,
-4.93319696712548));
#53393=CARTESIAN_POINT('Ctrl Pts',(-0.77392900016589,-0.130344377911946,
-4.91733945654953));
#53394=CARTESIAN_POINT('Ctrl Pts',(-0.617579411575381,-0.484305094490272,
-4.90148194597358));
#53395=CARTESIAN_POINT('Ctrl Pts',(-0.311101743527395,-0.720535536476336,
-4.88562443539765));
#53396=CARTESIAN_POINT('Ctrl Pts',(0.0710020001251872,-0.781610177856742,
-4.8697669248217));
#53397=CARTESIAN_POINT('Ctrl Pts',(0.43584578705537,-0.652682314803389,
-4.85390941424576));
#53398=CARTESIAN_POINT('Ctrl Pts',(0.69473932738756,-0.365093167742298,
-4.83805190366982));
#53399=CARTESIAN_POINT('Ctrl Pts',(0.784747896832823,0.0112468914587877,
-4.82219439309387));
#53400=CARTESIAN_POINT('Ctrl Pts',(0.68399121018045,0.384852931061866,-4.80633688251793));
#53401=CARTESIAN_POINT('Ctrl Pts',(0.416962324640737,0.664904635253221,
-4.79047937194199));
#53402=CARTESIAN_POINT('Ctrl Pts',(0.048573594794104,0.783323917699316,
-4.77462186136604));
#53403=CARTESIAN_POINT('Ctrl Pts',(-0.331622945290539,0.71132410075004,
-4.75876435079011));
#53404=CARTESIAN_POINT('Ctrl Pts',(-0.631204887564187,0.466407701551024,
-4.74290684021414));
#53405=CARTESIAN_POINT('Ctrl Pts',(-0.777346517971772,0.108111725303905,
-4.72704932963822));
#53406=CARTESIAN_POINT('Ctrl Pts',(-0.734522101861767,-0.276465252839481,
-4.71119181906226));
#53407=CARTESIAN_POINT('Ctrl Pts',(-0.513141875106644,-0.593835979175278,
-4.69533430848633));
#53408=CARTESIAN_POINT('Ctrl Pts',(-0.167021408060069,-0.766850443959353,
-4.67947679791038));
#53409=CARTESIAN_POINT('Ctrl Pts',(0.219700482463985,-0.753450364759431,
-4.66361928733444));
#53410=CARTESIAN_POINT('Ctrl Pts',(0.553015133578838,-0.556893182023092,
-4.64776177675849));
#53411=CARTESIAN_POINT('Ctrl Pts',(0.751896708786371,-0.224960204185648,
-4.63190426618255));
#53412=CARTESIAN_POINT('Ctrl Pts',(0.767998860449733,0.161658604778522,
-4.61604675560661));
#53413=CARTESIAN_POINT('Ctrl Pts',(0.59740729826221,0.508979640196021,-4.60018924503066));
#53414=CARTESIAN_POINT('Ctrl Pts',(0.281591318516465,0.732572237726208,
-4.58433173445472));
#53415=CARTESIAN_POINT('Ctrl Pts',(-0.102677014154933,0.778083019295018,
-4.56847422387877));
#53416=CARTESIAN_POINT('Ctrl Pts',(-0.461985475025898,0.634448717404426,
-4.55261671330284));
#53417=CARTESIAN_POINT('Ctrl Pts',(-0.708989362909296,0.336585557373601,
-4.53675920272689));
#53418=CARTESIAN_POINT('Ctrl Pts',(-0.783644222612109,-0.0430985674667928,
-4.52090169215095));
#53419=CARTESIAN_POINT('Ctrl Pts',(-0.667802119635095,-0.412305812670522,
-4.50504418157501));
#53420=CARTESIAN_POINT('Ctrl Pts',(-0.389623242148861,-0.681285170342373,
-4.48918667099906));
#53421=CARTESIAN_POINT('Ctrl Pts',(-0.0167304089195194,-0.784650143419608,
-4.47332916042312));
#53422=CARTESIAN_POINT('Ctrl Pts',(0.360229438385337,-0.697273623387268,
-4.45747164984717));
#53423=CARTESIAN_POINT('Ctrl Pts',(0.649620703034755,-0.440396067579693,
-4.44161413927123));
#53424=CARTESIAN_POINT('Ctrl Pts',(0.78109493435295,-0.0764621323217238,
-4.42575662869529));
#53425=CARTESIAN_POINT('Ctrl Pts',(0.72269191236498,0.306059069385753,-4.40989911811935));
#53426=CARTESIAN_POINT('Ctrl Pts',(0.488608893911385,0.614180024863817,
-4.39404160754339));
#53427=CARTESIAN_POINT('Ctrl Pts',(0.135749385384003,0.772999261654816,
-4.37818409696746));
#53428=CARTESIAN_POINT('Ctrl Pts',(-0.250109595167953,0.74390923139584,
-4.36232658639151));
#53429=CARTESIAN_POINT('Ctrl Pts',(-0.57516915062141,0.53398146252887,-4.34646907581558));
#53430=CARTESIAN_POINT('Ctrl Pts',(-0.760410185043356,0.194247534433146,
-4.33061156523962));
#53431=CARTESIAN_POINT('Ctrl Pts',(-0.760802245324052,-0.192706247072863,
-4.31475405466368));
#53432=CARTESIAN_POINT('Ctrl Pts',(-0.576250025085295,-0.532814848460723,
-4.29889654408774));
#53433=CARTESIAN_POINT('Ctrl Pts',(-0.251616532815955,-0.743400884156524,
-4.28303903351179));
#53434=CARTESIAN_POINT('Ctrl Pts',(0.13418270773351,-0.773272755951178,
-4.26718152293586));
#53435=CARTESIAN_POINT('Ctrl Pts',(0.487363321704981,-0.615168876657226,
-4.25132401235991));
#53436=CARTESIAN_POINT('Ctrl Pts',(0.722070233162724,-0.30752289757245,
-4.23546650178397));
#53437=CARTESIAN_POINT('Ctrl Pts',(0.781248272857062,0.0748791713955384,
-4.21960899120802));
#53438=CARTESIAN_POINT('Ctrl Pts',(0.65051178401439,0.439078777680545,-4.20375148063208));
#53439=CARTESIAN_POINT('Ctrl Pts',(0.361641647954727,0.696542226010465,
-4.18789397005614));
#53440=CARTESIAN_POINT('Ctrl Pts',(-0.0151403663859606,0.78468243478284,
-4.17203645948019));
#53441=CARTESIAN_POINT('Ctrl Pts',(-0.388241891893626,0.682073300701532,
-4.15617894890425));
#53442=CARTESIAN_POINT('Ctrl Pts',(-0.666965255658098,0.413658194522911,
-4.14032143832831));
#53443=CARTESIAN_POINT('Ctrl Pts',(-0.783555279126468,0.0446864487743974,
-4.12446392775236));
#53444=CARTESIAN_POINT('Ctrl Pts',(-0.709669961287797,-0.335148176478406,
-4.10860641717643));
#53445=CARTESIAN_POINT('Ctrl Pts',(-0.463270167836958,-0.63351125147336,
-4.09274890660047));
#53446=CARTESIAN_POINT('Ctrl Pts',(-0.104253503966341,-0.777873357984297,
-4.07689139602453));
#53447=CARTESIAN_POINT('Ctrl Pts',(0.280106262400609,-0.733141347841593,
-4.06103388544859));
#53448=CARTESIAN_POINT('Ctrl Pts',(0.596374679817071,-0.510189176114225,
-4.04517637487265));
#53449=CARTESIAN_POINT('Ctrl Pts',(0.767669700064063,-0.163214539041649,
-4.0293188642967));
#53450=CARTESIAN_POINT('Ctrl Pts',(0.752351022431571,0.223436105401952,
-4.01346135372076));
#53451=CARTESIAN_POINT('Ctrl Pts',(0.554142481635739,0.555771413620393,
-3.99760384314482));
#53452=CARTESIAN_POINT('Ctrl Pts',(0.22122681661509,0.75300361869076,-3.98174633256887));
#53453=CARTESIAN_POINT('Ctrl Pts',(-0.165467126114326,0.76718732023313,
-3.96588882199293));
#53454=CARTESIAN_POINT('Ctrl Pts',(-0.511937477526917,0.59487458615611,
-3.95003131141698));
#53455=CARTESIAN_POINT('Ctrl Pts',(-0.733960367021422,0.277953114378677,
-3.93417380084104));
#53456=CARTESIAN_POINT('Ctrl Pts',(-0.77756399863012,-0.106536295155054,
-3.9183162902651));
#53457=CARTESIAN_POINT('Ctrl Pts',(-0.632148716101378,-0.465127675893839,
-3.90245877968915));
#53458=CARTESIAN_POINT('Ctrl Pts',(-0.333063685357226,-0.710650642473002,
-3.88660126911321));
#53459=CARTESIAN_POINT('Ctrl Pts',(0.0469861743344437,-0.783420738538645,
-3.87074375853727));
#53460=CARTESIAN_POINT('Ctrl Pts',(0.415614111627677,-0.665748198921305,
-3.85488624796133));
#53461=CARTESIAN_POINT('Ctrl Pts',(0.683209943244133,-0.386238174710081,
-3.83902873738538));
#53462=CARTESIAN_POINT('Ctrl Pts',(0.784723495038708,-0.0128370746379034,
-3.82317122680944));
#53463=CARTESIAN_POINT('Ctrl Pts',(0.695477722595448,0.363684604464468,
-3.8073137162335));
#53464=CARTESIAN_POINT('Ctrl Pts',(0.437167481936875,0.651797780671273,
-3.79145620565755));
#53465=CARTESIAN_POINT('Ctrl Pts',(0.0725857023728426,0.781464695275524,
-3.77559869508161));
#53466=CARTESIAN_POINT('Ctrl Pts',(-0.309641017888792,0.721164470971649,
-3.75974118450566));
#53467=CARTESIAN_POINT('Ctrl Pts',(-0.616596751997694,0.485555557662479,
-3.74388367392972));
#53468=CARTESIAN_POINT('Ctrl Pts',(-0.773663282480133,0.131912393250565,
-3.72802616335378));
#53469=CARTESIAN_POINT('Ctrl Pts',(-0.74265912833721,-0.253797504417287,
-3.71216865277783));
#53470=CARTESIAN_POINT('Ctrl Pts',(-0.531121124556358,-0.577811478945351,
-3.69631114220189));
#53471=CARTESIAN_POINT('Ctrl Pts',(-0.190472284347944,-0.761364605853399,
-3.68045363162595));
#53472=CARTESIAN_POINT('Ctrl Pts',(0.196478679446638,-0.759836747383233,
-3.66459612105));
#53473=CARTESIAN_POINT('Ctrl Pts',(0.535667418259626,-0.573599312382862,
-3.64873861047406));
#53474=CARTESIAN_POINT('Ctrl Pts',(0.744640156953499,-0.247924970108488,
-3.63288109989812));
#53475=CARTESIAN_POINT('Ctrl Pts',(0.772597475516741,0.138017734281446,
-3.61702358932217));
#53476=CARTESIAN_POINT('Ctrl Pts',(0.612743197677913,0.490409551141159,
-3.60116607874623));
#53477=CARTESIAN_POINT('Ctrl Pts',(0.303936481101913,0.723587154119262,
-3.58530856817028));
#53478=CARTESIAN_POINT('Ctrl Pts',(-0.0787544993106969,0.78086713529854,
-3.56945105759435));
#53479=CARTESIAN_POINT('Ctrl Pts',(-0.442300959183037,0.648325239102095,
-3.55359354701839));
#53480=CARTESIAN_POINT('Ctrl Pts',(-0.698327977345097,0.358181225370803,
-3.53773603644246));
#53481=CARTESIAN_POINT('Ctrl Pts',(-0.784597655632743,-0.0190334685916752,
-3.52187852586651));
#53482=CARTESIAN_POINT('Ctrl Pts',(-0.680138600126441,-0.391621295091407,
-3.50602101529057));
#53483=CARTESIAN_POINT('Ctrl Pts',(-0.410343881079456,-0.669009456892558,
-3.49016350471463));
#53484=CARTESIAN_POINT('Ctrl Pts',(-0.0407982026757765,-0.783767351201523,
-3.47430599413868));
#53485=CARTESIAN_POINT('Ctrl Pts',(0.338665157079046,-0.707998351362241,
-3.45844848356274));
#53486=CARTESIAN_POINT('Ctrl Pts',(0.635802019773763,-0.460121229463095,
-3.4425909729868));
#53487=CARTESIAN_POINT('Ctrl Pts',(0.778381048520723,-0.10039271614418,
-3.42673346241085));
#53488=CARTESIAN_POINT('Ctrl Pts',(0.731742545545852,0.283740376381475,
-3.41087595183491));
#53489=CARTESIAN_POINT('Ctrl Pts',(0.507223917422551,0.59889869906817,-3.39501844125896));
#53490=CARTESIAN_POINT('Ctrl Pts',(0.159403652051826,0.768470057883562,
-3.37916093068303));
#53491=CARTESIAN_POINT('Ctrl Pts',(-0.227166227850259,0.751233158929577,
-3.36330342010708));
#53492=CARTESIAN_POINT('Ctrl Pts',(-0.558514011831493,0.551378139518531,
-3.34744590953114));
#53493=CARTESIAN_POINT('Ctrl Pts',(-0.754091991355572,0.217487982942537,
-3.33158839895519));
#53494=CARTESIAN_POINT('Ctrl Pts',(-0.766356893606415,-0.169271574025148,
-3.31573088837925));
#53495=CARTESIAN_POINT('Ctrl Pts',(-0.592327229588209,-0.514882712119356,
-3.2998733778033));
#53496=CARTESIAN_POINT('Ctrl Pts',(-0.274308067666229,-0.735330427878682,
-3.28401586722736));
#53497=CARTESIAN_POINT('Ctrl Pts',(0.110392953473453,-0.777025836104844,
-3.26815835665142));
#53498=CARTESIAN_POINT('Ctrl Pts',(0.468258426374354,-0.629833152732085,
-3.25230084607548));
#53499=CARTESIAN_POINT('Ctrl Pts',(0.712294427431246,-0.329533614069066,
-3.23644333549953));
#53500=CARTESIAN_POINT('Ctrl Pts',(0.78317796842517,0.050872624509148,-3.22058582492359));
#53501=CARTESIAN_POINT('Ctrl Pts',(0.663677888998276,0.418912179108962,
-3.20472831434765));
#53502=CARTESIAN_POINT('Ctrl Pts',(0.382843598964291,0.685117897068157,
-3.1888708037717));
#53503=CARTESIAN_POINT('Ctrl Pts',(0.00894342433664182,0.784777528546888,
-3.17301329319576));
#53504=CARTESIAN_POINT('Ctrl Pts',(-0.367130817454304,0.693664700721004,
-3.15715578261982));
#53505=CARTESIAN_POINT('Ctrl Pts',(-0.653958812526187,0.433928134223127,
-3.14129827204387));
#53506=CARTESIAN_POINT('Ctrl Pts',(-0.781815218311425,0.0687074855287506,
-3.12544076146793));
#53507=CARTESIAN_POINT('Ctrl Pts',(-0.719619276146273,-0.313215343732932,
-3.10958325089198));
#53508=CARTESIAN_POINT('Ctrl Pts',(-0.482490268138086,-0.618998299919365,
-3.09372574031604));
#53509=CARTESIAN_POINT('Ctrl Pts',(-0.128072153733491,-0.774308257471849,
-3.07786822974009));
#53510=CARTESIAN_POINT('Ctrl Pts',(0.257479165748238,-0.74139074269687,
-3.06201071916415));
#53511=CARTESIAN_POINT('Ctrl Pts',(0.58043958286246,-0.528247711587546,
-3.04615320858821));
#53512=CARTESIAN_POINT('Ctrl Pts',(0.762300283595343,-0.186692345267518,
-3.03029569801227));
#53513=CARTESIAN_POINT('Ctrl Pts',(0.758852543986716,0.200246274961393,
-3.01443818743632));
#53514=CARTESIAN_POINT('Ctrl Pts',(0.570934478967572,0.538506801142803,
-2.99858067686038));
#53515=CARTESIAN_POINT('Ctrl Pts',(0.244227304051109,0.745861098400332,
-2.98272316628443));
#53516=CARTESIAN_POINT('Ctrl Pts',(-0.141849363146094,0.771903175486456,
-2.96686565570849));
#53517=CARTESIAN_POINT('Ctrl Pts',(-0.493443707807536,0.610302434352163,
-2.95100814513255));
#53518=CARTESIAN_POINT('Ctrl Pts',(-0.72508626200279,0.300342582405237,
-2.93515063455661));
#53519=CARTESIAN_POINT('Ctrl Pts',(-0.780466774563917,-0.0826278884688641,
-2.91929312398066));
#53520=CARTESIAN_POINT('Ctrl Pts',(-0.646122733894283,-0.445512252240051,
-2.90343561340472));
#53521=CARTESIAN_POINT('Ctrl Pts',(-0.354711985178273,-0.700096537430314,
-2.88757810282877));
#53522=CARTESIAN_POINT('Ctrl Pts',(0.0229261022366121,-0.784493561469602,
-2.87172059225283));
#53523=CARTESIAN_POINT('Ctrl Pts',(0.394991057461987,-0.678187156083102,
-2.85586308167689));
#53524=CARTESIAN_POINT('Ctrl Pts',(0.671037188633014,-0.407019465901235,
-2.84000557110095));
#53525=CARTESIAN_POINT('Ctrl Pts',(0.783960128703746,-0.0369089522180315,
-2.824148060525));
#53526=CARTESIAN_POINT('Ctrl Pts',(0.706309312124615,0.342173800512369,
-2.80829054994906));
#53527=CARTESIAN_POINT('Ctrl Pts',(0.456960963949165,0.638077136071867,
-2.79243303937312));
#53528=CARTESIAN_POINT('Ctrl Pts',(0.0965294568812757,0.778869577082859,
-2.77657552879717));
#53529=CARTESIAN_POINT('Ctrl Pts',(-0.287367505318435,0.730325729409888,
-2.76071801822123));
#53530=CARTESIAN_POINT('Ctrl Pts',(-0.601407974792955,0.504246172029558,
-2.74486050764528));
#53531=CARTESIAN_POINT('Ctrl Pts',(-0.769251497714866,0.155588840905967,
-2.72900299706934));
#53532=CARTESIAN_POINT('Ctrl Pts',(-0.750096801772698,-0.230890757981771,
-2.7131454864934));
#53533=CARTESIAN_POINT('Ctrl Pts',(-0.548600223723299,-0.561242860695591,
-2.69728797591745));
#53534=CARTESIAN_POINT('Ctrl Pts',(-0.213743795209606,-0.755161799987539,
-2.68143046534151));
#53535=CARTESIAN_POINT('Ctrl Pts',(0.173071854854098,-0.76550760101281,
-2.66557295476557));
#53536=CARTESIAN_POINT('Ctrl Pts',(0.51781527146833,-0.589765291268659,
-2.64971544418963));
#53537=CARTESIAN_POINT('Ctrl Pts',(0.736682386570194,-0.270656268111916,
-2.63385793361368));
#53538=CARTESIAN_POINT('Ctrl Pts',(0.776468544967536,0.114246894167955,
-2.61800042303774));
#53539=CARTESIAN_POINT('Ctrl Pts',(0.627502084300454,0.471377649395485,
-2.60214291246179));
#53540=CARTESIAN_POINT('Ctrl Pts',(0.325995430411447,0.713920677317781,
-2.58628540188585));
#53541=CARTESIAN_POINT('Ctrl Pts',(-0.0547578223153314,0.782915918248127,
-2.57042789130991));
#53542=CARTESIAN_POINT('Ctrl Pts',(-0.422199933923428,0.661591240832344,
-2.55457038073396));
#53543=CARTESIAN_POINT('Ctrl Pts',(-0.687008984844947,0.379439598478257,
-2.53871287015802));
#53544=CARTESIAN_POINT('Ctrl Pts',(-0.784812242613961,0.00504955386858817,
-2.52285535958208));
#53545=CARTESIAN_POINT('Ctrl Pts',(-0.691834602396433,-0.370567992516886,
-2.50699784900614));
#53546=CARTESIAN_POINT('Ctrl Pts',(-0.430678104183853,-0.656103745399787,
-2.49114033843019));
#53547=CARTESIAN_POINT('Ctrl Pts',(-0.0648275772623532,-0.782146494831576,
-2.47528282785425));
#53548=CARTESIAN_POINT('Ctrl Pts',(0.316781958926394,-0.718056365928039,
-2.4594253172783));
#53549=CARTESIAN_POINT('Ctrl Pts',(0.621384609508185,-0.479413100798661,
-2.44356780670236));
#53550=CARTESIAN_POINT('Ctrl Pts',(0.774934170752148,-0.124228761370738,
-2.42771029612641));
#53551=CARTESIAN_POINT('Ctrl Pts',(0.740104105699592,0.261154488526679,
-2.41185278555047));
#53552=CARTESIAN_POINT('Ctrl Pts',(0.525361294359332,0.583053397674786,
-2.39599527497453));
#53553=CARTESIAN_POINT('Ctrl Pts',(0.1829078102454,0.763217195234921,-2.38013776439859));
#53554=CARTESIAN_POINT('Ctrl Pts',(-0.20400894086746,0.757849659363361,
-2.36428025382264));
#53555=CARTESIAN_POINT('Ctrl Pts',(-0.541332927211076,0.568255590441586,
-2.3484227432467));
#53556=CARTESIAN_POINT('Ctrl Pts',(-0.747063678440222,0.240523625671967,
-2.33256523267075));
#53557=CARTESIAN_POINT('Ctrl Pts',(-0.771189872952408,-0.14567750000146,
-2.31670772209481));
#53558=CARTESIAN_POINT('Ctrl Pts',(-0.607846646766021,-0.496465717010077,
-2.30085021151887));
#53559=CARTESIAN_POINT('Ctrl Pts',(-0.296741289956032,-0.726567519908682,
-2.28499270094293));
#53560=CARTESIAN_POINT('Ctrl Pts',(0.0864992435160036,-0.780047200509165,
-2.26913519036698));
#53561=CARTESIAN_POINT('Ctrl Pts',(0.448712577796839,-0.64390432261163,
-2.25327767979104));
#53562=CARTESIAN_POINT('Ctrl Pts',(0.701847862728175,-0.351234012781961,
-2.23742016921509));
#53563=CARTESIAN_POINT('Ctrl Pts',(0.784370154855984,0.0268181714929559,
-2.22156265863915));
#53564=CARTESIAN_POINT('Ctrl Pts',(0.67621901661164,0.398351096049469,-2.2057051480632));
#53565=CARTESIAN_POINT('Ctrl Pts',(0.403685030827794,0.67304840096132,-2.18984763748727));
#53566=CARTESIAN_POINT('Ctrl Pts',(0.0330187931456675,0.78413360688739,
-2.17399012691132));
#53567=CARTESIAN_POINT('Ctrl Pts',(-0.345674020403545,0.704602885155229,
-2.15813261633538));
#53568=CARTESIAN_POINT('Ctrl Pts',(-0.640336544359476,0.453789449093728,
-2.14227510575943));
#53569=CARTESIAN_POINT('Ctrl Pts',(-0.779338931644242,0.092663821282302,
-2.12641759518349));
#53570=CARTESIAN_POINT('Ctrl Pts',(-0.728890934312499,-0.290987559919799,
-2.11056008460755));
#53571=CARTESIAN_POINT('Ctrl Pts',(-0.501256013240592,-0.60390244521874,
-2.0947025740316));
#53572=CARTESIAN_POINT('Ctrl Pts',(-0.151770199516093,-0.77001400032069,
-2.07884506345566));
#53573=CARTESIAN_POINT('Ctrl Pts',(0.23460960410698,-0.748941978935479,
-2.06298755287972));
#53574=CARTESIAN_POINT('Ctrl Pts',(0.563957893034617,-0.545808802636034,
-2.04713004230377));
#53575=CARTESIAN_POINT('Ctrl Pts',(0.7562130182504,-0.209994345589698,-2.03127253172783));
#53576=CARTESIAN_POINT('Ctrl Pts',(0.764639463359969,0.176867875046899,
-2.01541502115189));
#53577=CARTESIAN_POINT('Ctrl Pts',(0.587188834266557,0.520735083380895,
-1.99955751057594));
#53578=CARTESIAN_POINT('Ctrl Pts',(0.266997805614742,0.738016209813808,
-1.9837));
#53579=CARTESIAN_POINT('Ctrl Pts',(-0.118098022363289,0.775892138937434,
-1.96784248942406));
#53580=CARTESIAN_POINT('Ctrl Pts',(-0.474485268169029,0.625155568192103,
-1.95198497884811));
#53581=CARTESIAN_POINT('Ctrl Pts',(-0.715529352098025,0.322449221486431,
-1.93612746827217));
#53582=CARTESIAN_POINT('Ctrl Pts',(-0.782634594458599,-0.0586416721082485,
-1.92026995769623));
#53583=CARTESIAN_POINT('Ctrl Pts',(-0.659488305792038,-0.425477295134033,
-1.90441244712028));
#53584=CARTESIAN_POINT('Ctrl Pts',(-0.376026257050732,-0.688883160020217,
-1.88855493654434));
#53585=CARTESIAN_POINT('Ctrl Pts',(-0.00115555909198516,-0.784827636385346,
-1.8726974259684));
#53586=CARTESIAN_POINT('Ctrl Pts',(0.373996045036767,-0.6899874726746,-1.85683991539245));
#53587=CARTESIAN_POINT('Ctrl Pts',(0.658232526488693,-0.427417471827413,
-1.84098240481651));
#53588=CARTESIAN_POINT('Ctrl Pts',(0.782458516680696,-0.0609460730881939,
-1.82512489424057));
#53589=CARTESIAN_POINT('Ctrl Pts',(0.716475778792257,0.320340775667187,
-1.80926738366462));
#53590=CARTESIAN_POINT('Ctrl Pts',(0.476324131397102,0.623755622018608,
-1.79340987308868));
#53591=CARTESIAN_POINT('Ctrl Pts',(0.120382310777934,0.77554100691246,-1.77755236251274));
#53592=CARTESIAN_POINT('Ctrl Pts',(-0.264823382274487,0.738799249019466,
-1.76169485193679));
#53593=CARTESIAN_POINT('Ctrl Pts',(-0.585652859036139,0.522461943928764,
-1.74583734136085));
#53594=CARTESIAN_POINT('Ctrl Pts',(-0.764115318199852,0.179118772448241,
-1.72997983078491));
#53595=CARTESIAN_POINT('Ctrl Pts',(-0.756828118201908,-0.207766584536555,
-1.71412232020896));
#53596=CARTESIAN_POINT('Ctrl Pts',(-0.565562712753049,-0.544145726891646,
-1.69826480963302));
#53597=CARTESIAN_POINT('Ctrl Pts',(-0.236814026147216,-0.748247867468375,
-1.68240729905707));
#53598=CARTESIAN_POINT('Ctrl Pts',(0.149502050607495,-0.77045758547449,
-1.66654978848113));
#53599=CARTESIAN_POINT('Ctrl Pts',(0.499475504353768,-0.605375895375407,
-1.65069227790519));
#53600=CARTESIAN_POINT('Ctrl Pts',(0.728030891371734,-0.293132692409946,
-1.63483476732925));
#53601=CARTESIAN_POINT('Ctrl Pts',(0.779608423463245,0.0903684691481552,
-1.6189772567533));
#53602=CARTESIAN_POINT('Ctrl Pts',(0.641670059866376,0.451901857068663,
-1.60311974617736));
#53603=CARTESIAN_POINT('Ctrl Pts',(0.347747393801637,0.703581910125037,
-1.58726223560141));
#53604=CARTESIAN_POINT('Ctrl Pts',(-0.0307095805468093,0.784227438829875,
-1.57140472502547));
#53605=CARTESIAN_POINT('Ctrl Pts',(-0.401701328137329,0.674234230163178,
-1.55554721444953));
#53606=CARTESIAN_POINT('Ctrl Pts',(-0.675043044365986,0.400340657945363,
-1.53968970387359));
#53607=CARTESIAN_POINT('Ctrl Pts',(-0.78428778148182,0.0291278212255782,
-1.52383219329764));
#53608=CARTESIAN_POINT('Ctrl Pts',(-0.702879112462439,-0.349165730585115,
-1.5079746827217));
#53609=CARTESIAN_POINT('Ctrl Pts',(-0.450606762972262,-0.642580189015103,
-1.49211717214575));
#53610=CARTESIAN_POINT('Ctrl Pts',(-0.0887959045103961,-0.779789100650431,
-1.47625966156981));
#53611=CARTESIAN_POINT('Ctrl Pts',(0.294600451068075,-0.727438195575069,
-1.46040215099386));
#53612=CARTESIAN_POINT('Ctrl Pts',(0.606382048937353,-0.498253514666544,
-1.44454464041793));
#53613=CARTESIAN_POINT('Ctrl Pts',(0.770757546929961,-0.147947821888442,
-1.42868712984198));
#53614=CARTESIAN_POINT('Ctrl Pts',(0.747768718847025,0.238322674676382,
-1.41282961926604));
#53615=CARTESIAN_POINT('Ctrl Pts',(0.543003944975163,0.566659042010658,
-1.39697210869009));
#53616=CARTESIAN_POINT('Ctrl Pts',(0.206239726385727,0.757245620265555,
-1.38111459811415));
#53617=CARTESIAN_POINT('Ctrl Pts',(-0.180659541154162,0.763752502019466,
-1.3652570875382));
#53618=CARTESIAN_POINT('Ctrl Pts',(-0.52364207597792,0.584597922008419,
-1.34939957696226));
#53619=CARTESIAN_POINT('Ctrl Pts',(-0.739331864773827,0.263332770237737,
-1.33354206638632));
#53620=CARTESIAN_POINT('Ctrl Pts',(-0.775296632204346,-0.121946243253436,
-1.31768455581038));
#53621=CARTESIAN_POINT('Ctrl Pts',(-0.622793662172921,-0.477581206192484,
-1.30182704523443));
#53622=CARTESIAN_POINT('Ctrl Pts',(-0.318895074593618,-0.71712041217006,
-1.28596953465849));
#53623=CARTESIAN_POINT('Ctrl Pts',(0.062524078276333,-0.782334003982136,
-1.27011202408255));
#53624=CARTESIAN_POINT('Ctrl Pts',(0.428744182059569,-0.657369135646856,
-1.2542545135066));
#53625=CARTESIAN_POINT('Ctrl Pts',(0.690740376456031,-0.372603658710436,
-1.23839700293066));
#53626=CARTESIAN_POINT('Ctrl Pts',(0.784823709482088,0.00273846413186627,
-1.22253949235471));
#53627=CARTESIAN_POINT('Ctrl Pts',(0.688123357027629,0.377414890623108,
-1.20668198177877));
#53628=CARTESIAN_POINT('Ctrl Pts',(0.424146317423146,0.660345103387168,
-1.19082447120283));
#53629=CARTESIAN_POINT('Ctrl Pts',(0.0570630685600556,0.78275127617752,
-1.17496696062689));
#53630=CARTESIAN_POINT('Ctrl Pts',(-0.32389170634536,0.714877553649376,
-1.15910945005094));
#53631=CARTESIAN_POINT('Ctrl Pts',(-0.626111279081718,0.473223435976791,
-1.143251939475));
#53632=CARTESIAN_POINT('Ctrl Pts',(-0.776128751013863,0.116532896645915,
-1.12739442889905));
#53633=CARTESIAN_POINT('Ctrl Pts',(-0.737476204779087,-0.268485756671859,
-1.11153691832311));
#53634=CARTESIAN_POINT('Ctrl Pts',(-0.519549731671247,-0.588237902953695,
-1.09567940774717));
#53635=CARTESIAN_POINT('Ctrl Pts',(-0.17532532515354,-0.764994630380392,
-1.07982189717122));
#53636=CARTESIAN_POINT('Ctrl Pts',(0.211519113464033,-0.755787945650376,
-1.06396438659528));
#53637=CARTESIAN_POINT('Ctrl Pts',(0.546945130939781,-0.562855912194491,
-1.04810687601934));
#53638=CARTESIAN_POINT('Ctrl Pts',(0.74941363633275,-0.233098596798759,
-1.03224936544339));
#53639=CARTESIAN_POINT('Ctrl Pts',(0.769706331079953,0.153322920812463,
-1.01639185486745));
#53640=CARTESIAN_POINT('Ctrl Pts',(0.602890241004603,0.502472995744484,
-1.00053434429151));
#53641=CARTESIAN_POINT('Ctrl Pts',(0.289516878602456,0.729476340367059,
-0.984676833715564));
#53642=CARTESIAN_POINT('Ctrl Pts',(-0.0942354701137554,0.77915045422785,
-0.96881932313962));
#53643=CARTESIAN_POINT('Ctrl Pts',(-0.455080011542695,0.639420000661008,
-0.952961812563677));
#53644=CARTESIAN_POINT('Ctrl Pts',(-0.705298636932576,0.344252214069966,
-0.937104301987735));
#53645=CARTESIAN_POINT('Ctrl Pts',(-0.784065416904622,-0.0346002336004862,
-0.92124679141179));
#53646=CARTESIAN_POINT('Ctrl Pts',(-0.672232845598666,-0.405041671250436,
-0.905389280835848));
#53647=CARTESIAN_POINT('Ctrl Pts',(-0.39698642958483,-0.677021069743413,
-0.889531770259904));
#53648=CARTESIAN_POINT('Ctrl Pts',(-0.0252361322446689,-0.784422648691607,
-0.87367425968396));
#53649=CARTESIAN_POINT('Ctrl Pts',(0.352648845099092,-0.70113803648162,
-0.857816749108016));
#53650=CARTESIAN_POINT('Ctrl Pts',(0.644808014805302,-0.447412983935282,
-0.841959238532074));
#53651=CARTESIAN_POINT('Ctrl Pts',(0.780220073019283,-0.0849258017849115,
-0.82610172795613));
#53652=CARTESIAN_POINT('Ctrl Pts',(0.725967548960737,0.298206089822066,
-0.810244217380186));
#53653=CARTESIAN_POINT('Ctrl Pts',(0.495238750222128,0.608846724906565,
-0.794386706804243));
#53654=CARTESIAN_POINT('Ctrl Pts',(0.144121802121297,0.771482119238247,
-0.778529196228299));
#53655=CARTESIAN_POINT('Ctrl Pts',(-0.242029878282588,0.746577050390341,
-0.762671685652355));
#53656=CARTESIAN_POINT('Ctrl Pts',(-0.569346241127547,0.540185719789925,
-0.746814175076413));
#53657=CARTESIAN_POINT('Ctrl Pts',(-0.758259580612683,0.202480030027912,
-0.730956664500469));
#53658=CARTESIAN_POINT('Ctrl Pts',(-0.762846738826278,-0.184446759833668,
-0.715099153924525));
#53659=CARTESIAN_POINT('Ctrl Pts',(-0.58199261827663,-0.526536177695834,
-0.699241643348582));
#53660=CARTESIAN_POINT('Ctrl Pts',(-0.259661252205769,-0.740629319061807,
-0.683384132772639));
#53661=CARTESIAN_POINT('Ctrl Pts',(0.12579146210391,-0.774682039428296,
-0.667526622196696));
#53662=CARTESIAN_POINT('Ctrl Pts',(0.480665387250857,-0.620416424387693,
-0.651669111620751));
#53663=CARTESIAN_POINT('Ctrl Pts',(0.718693818365588,-0.315333077228062,
-0.63581160104481));
#53664=CARTESIAN_POINT('Ctrl Pts',(0.782014154218595,0.0664049452435352,
-0.619954090468865));
#53665=CARTESIAN_POINT('Ctrl Pts',(0.655233782565965,0.432000514276696,
-0.604096579892922));
#53666=CARTESIAN_POINT('Ctrl Pts',(0.369171887713958,0.692580588431942,
-0.588239069316979));
#53667=CARTESIAN_POINT('Ctrl Pts',(-0.00663241994093424,0.784800462000848,
-0.572381558741035));
#53668=CARTESIAN_POINT('Ctrl Pts',(-0.380824445111711,0.686242301345836,
-0.556524048165091));
#53669=CARTESIAN_POINT('Ctrl Pts',(-0.66244142408827,0.420864721499445,
-0.540666537589149));
#53670=CARTESIAN_POINT('Ctrl Pts',(-0.78302476611513,0.0531786592687593,
-0.524809027013205));
#53671=CARTESIAN_POINT('Ctrl Pts',(-0.713261729843775,-0.327434663545121,
-0.508951516437261));
#53672=CARTESIAN_POINT('Ctrl Pts',(-0.470111090870426,-0.628451522706413,
-0.493094005861318));
#53673=CARTESIAN_POINT('Ctrl Pts',(-0.112680613737367,-0.776697388587739,
-0.477236495285375));
#53674=CARTESIAN_POINT('Ctrl Pts',(0.27214152155714,-0.736135005548202,
-0.46137898470943));
#53675=CARTESIAN_POINT('Ctrl Pts',(0.590808465794012,-0.516624729280032,
-0.445521474133488));
#53676=CARTESIAN_POINT('Ctrl Pts',(0.765855110121114,-0.171527561745056,
-0.429663963557544));
#53677=CARTESIAN_POINT('Ctrl Pts',(0.754729167332557,0.215266435266626,
-0.4138064529816));
#53678=CARTESIAN_POINT('Ctrl Pts',(0.560135255367789,0.549731070449319,
-0.397948942405656));
#53679=CARTESIAN_POINT('Ctrl Pts',(0.229377429157334,0.750560956317521,
-0.382091431829714));
#53680=CARTESIAN_POINT('Ctrl Pts',(-0.157140016682746,0.768936128296654,
-0.36623392125377));
#53681=CARTESIAN_POINT('Ctrl Pts',(-0.505458117141541,0.600389744778999,
-0.350376410677827));
#53682=CARTESIAN_POINT('Ctrl Pts',(-0.730903831797943,0.285893937675275,
-0.334518900101885));
#53683=CARTESIAN_POINT('Ctrl Pts',(-0.778673303125677,-0.0981001514671905,
-0.31866138952594));
#53684=CARTESIAN_POINT('Ctrl Pts',(-0.637154202245931,-0.45824696248919,
-0.302803878949997));
#53685=CARTESIAN_POINT('Ctrl Pts',(-0.34074855599798,-0.706998001847843,
-0.286946368374054));
#53686=CARTESIAN_POINT('Ctrl Pts',(0.0384900277778693,-0.783884091195167,
-0.27108885779811));
#53687=CARTESIAN_POINT('Ctrl Pts',(0.408372057023997,-0.670214915848524,
-0.255231347222166));
#53688=CARTESIAN_POINT('Ctrl Pts',(0.678982401305158,-0.393622421166732,
-0.239373836646223));
#53689=CARTESIAN_POINT('Ctrl Pts',(0.784538258134674,-0.0213438359833095,
-0.223516326070279));
#53690=CARTESIAN_POINT('Ctrl Pts',(0.69937959664011,0.356123305506083,-0.207658815494336));
#53691=CARTESIAN_POINT('Ctrl Pts',(0.444208392702825,0.647019913531816,
-0.191801304918393));
#53692=CARTESIAN_POINT('Ctrl Pts',(0.0810532135089025,0.780631942388513,
-0.17594379434245));
#53693=CARTESIAN_POINT('Ctrl Pts',(-0.301803615892741,0.724478826986905,
-0.160086283766505));
#53694=CARTESIAN_POINT('Ctrl Pts',(-0.611297919935612,0.492212192112627,
-0.144228773190563));
#53695=CARTESIAN_POINT('Ctrl Pts',(-0.772184753739812,0.140291456659345,
-0.128371262614619));
#53696=CARTESIAN_POINT('Ctrl Pts',(-0.745372760934995,-0.24572960271599,
-0.112513752038676));
#53697=CARTESIAN_POINT('Ctrl Pts',(-0.537342918516762,-0.572022410205874,
-0.0966562414627321));
#53698=CARTESIAN_POINT('Ctrl Pts',(-0.19873767733096,-0.75924888856303,
-0.0807987308867897));
#53699=CARTESIAN_POINT('Ctrl Pts',(0.188276175770941,-0.761935501840704,
-0.0649412203108454));
#53700=CARTESIAN_POINT('Ctrl Pts',(0.415619971558626,-0.640197744227128,
-0.0543695465935496));
#53701=CARTESIAN_POINT('Ctrl Pts',(0.507924469142728,-0.555852079925216,
-0.0490837097349018));
#53702=CARTESIAN_POINT('Ctrl Pts',(0.415028236876536,-0.582012248186925,
-5.8309162902651));
#53703=CARTESIAN_POINT('Ctrl Pts',(0.511676877939308,-0.513092882277098,
-5.82563045340645));
#53704=CARTESIAN_POINT('Ctrl Pts',(0.669882320706702,-0.326248849454983,
-5.81505877968916));
#53705=CARTESIAN_POINT('Ctrl Pts',(0.744325517095435,0.0335534201836676,
-5.79920126911321));
#53706=CARTESIAN_POINT('Ctrl Pts',(0.637835333840713,0.385103548525349,
-5.78334375853727));
#53707=CARTESIAN_POINT('Ctrl Pts',(0.376290719986943,0.643085420323738,
-5.76748624796132));
#53708=CARTESIAN_POINT('Ctrl Pts',(0.0232743040931315,0.744715053663492,
-5.75162873738539));
#53709=CARTESIAN_POINT('Ctrl Pts',(-0.335400465408995,0.665323262153351,
-5.73577122680943));
#53710=CARTESIAN_POINT('Ctrl Pts',(-0.612542060764352,0.424191040961468,
-5.7199137162335));
#53711=CARTESIAN_POINT('Ctrl Pts',(-0.740780262763952,0.0799449338940462,
-5.70405620565754));
#53712=CARTESIAN_POINT('Ctrl Pts',(-0.688941273521715,-0.283736713152371,
-5.68819869508162));
#53713=CARTESIAN_POINT('Ctrl Pts',(-0.469626808375355,-0.578443643881164,
-5.67234118450566));
#53714=CARTESIAN_POINT('Ctrl Pts',(-0.136150209639541,-0.732536481667968,
-5.65648367392972));
#53715=CARTESIAN_POINT('Ctrl Pts',(0.230423287598442,-0.708555976232628,
-5.64062616335378));
#53716=CARTESIAN_POINT('Ctrl Pts',(0.540982931862801,-0.512331907284304,
-5.62476865277783));
#53717=CARTESIAN_POINT('Ctrl Pts',(0.72003441906891,-0.1915644366118,-5.60891114220189));
#53718=CARTESIAN_POINT('Ctrl Pts',(0.724051924255098,0.175770620786611,
-5.59305363162594));
#53719=CARTESIAN_POINT('Ctrl Pts',(0.552058825433282,0.500377413708016,
-5.57719612105001));
#53720=CARTESIAN_POINT('Ctrl Pts',(0.245865121098944,0.703346886034275,
-5.56133861047405));
#53721=CARTESIAN_POINT('Ctrl Pts',(-0.120096214505419,0.73533897022222,
-5.54548109989812));
#53722=CARTESIAN_POINT('Ctrl Pts',(-0.456863225048667,0.588576668292261,
-5.52962358932217));
#53723=CARTESIAN_POINT('Ctrl Pts',(-0.682570836208337,0.298736597689061,
-5.51376607874623));
#53724=CARTESIAN_POINT('Ctrl Pts',(-0.742351528775239,-0.0637236917238471,
-5.49790856817029));
#53725=CARTESIAN_POINT('Ctrl Pts',(-0.621673146443291,-0.410693316386423,
-5.48205105759435));
#53726=CARTESIAN_POINT('Ctrl Pts',(-0.349871533996248,-0.657827037205679,
-5.4661935470184));
#53727=CARTESIAN_POINT('Ctrl Pts',(0.00698074637971318,-0.745048837543795,
-5.45033603644245));
#53728=CARTESIAN_POINT('Ctrl Pts',(0.362136069204197,-0.651155871159418,
-5.43447852586652));
#53729=CARTESIAN_POINT('Ctrl Pts',(0.629259324324606,-0.398972685665058,
-5.41862101529057));
#53730=CARTESIAN_POINT('Ctrl Pts',(0.743415216753462,-0.049802777611032,
-5.40276350471463));
#53731=CARTESIAN_POINT('Ctrl Pts',(0.676853461153697,0.311473744130651,
-5.38690599413868));
#53732=CARTESIAN_POINT('Ctrl Pts',(0.445754630171398,0.597033760216781,
-5.37104848356274));
#53733=CARTESIAN_POINT('Ctrl Pts',(0.106296800681942,0.737460162532991,
-5.3551909729868));
#53734=CARTESIAN_POINT('Ctrl Pts',(-0.259000838619383,0.69861653770328,
-5.33933346241085));
#53735=CARTESIAN_POINT('Ctrl Pts',(-0.561337670369488,0.489945426534807,
-5.32347595183491));
#53736=CARTESIAN_POINT('Ctrl Pts',(-0.727218291306573,0.1621729260614,-5.30761844125897));
#53737=CARTESIAN_POINT('Ctrl Pts',(-0.716318593188485,-0.205022374902455,
-5.29176093068302));
#53738=CARTESIAN_POINT('Ctrl Pts',(-0.53128819599034,-0.522378554268369,
-5.27590342010708));
#53739=CARTESIAN_POINT('Ctrl Pts',(-0.217106348780294,-0.712749138531546,
-5.26004590953113));
#53740=CARTESIAN_POINT('Ctrl Pts',(0.149852126940193,-0.729856726494781,
-5.24418839895519));
#53741=CARTESIAN_POINT('Ctrl Pts',(0.48038287919956,-0.569542615201107,
-5.22833088837924));
#53742=CARTESIAN_POINT('Ctrl Pts',(0.69413681262924,-0.270777743751394,
-5.21247337780331));
#53743=CARTESIAN_POINT('Ctrl Pts',(0.739152241167806,0.093810796472393,
-5.19661586722736));
#53744=CARTESIAN_POINT('Ctrl Pts',(0.604486313247053,0.43559476380595,-5.18075835665142));
#53745=CARTESIAN_POINT('Ctrl Pts',(0.322875121988236,0.671489506067859,
-5.16490084607547));
#53746=CARTESIAN_POINT('Ctrl Pts',(-0.0372241487955211,0.744151102871337,
-5.14904333549953));
#53747=CARTESIAN_POINT('Ctrl Pts',(-0.388274559038646,0.635916164255573,
-5.13318582492358));
#53748=CARTESIAN_POINT('Ctrl Pts',(-0.64493886644525,0.37309564418054,-5.11732831434765));
#53749=CARTESIAN_POINT('Ctrl Pts',(-0.744824253486097,0.0195788808938151,
-5.1014708037717));
#53750=CARTESIAN_POINT('Ctrl Pts',(-0.663649468161454,-0.338697334750651,
-5.08561329319576));
#53751=CARTESIAN_POINT('Ctrl Pts',(-0.421147381083175,-0.614639231228336,
-5.06975578261981));
#53752=CARTESIAN_POINT('Ctrl Pts',(-0.0762680995817819,-0.741167780023092,
-5.05389827204387));
#53753=CARTESIAN_POINT('Ctrl Pts',(0.287151280730348,-0.687525012732699,
-5.03804076146793));
#53754=CARTESIAN_POINT('Ctrl Pts',(0.58076673059759,-0.46675101048542,-5.02218325089198));
#53755=CARTESIAN_POINT('Ctrl Pts',(0.733202937369596,-0.132513975831888,
-5.00632574031604));
#53756=CARTESIAN_POINT('Ctrl Pts',(0.707404010688734,0.233936031469435,
-4.9904682297401));
#53757=CARTESIAN_POINT('Ctrl Pts',(0.50964144089628,0.543518263611574,-4.97461071916415));
#53758=CARTESIAN_POINT('Ctrl Pts',(0.187989555333847,0.720976024735606,
-4.95875320858821));
#53759=CARTESIAN_POINT('Ctrl Pts',(-0.17936092440345,0.723170906463552,
-4.94289569801227));
#53760=CARTESIAN_POINT('Ctrl Pts',(-0.503110353643096,0.549569352507302,
-4.92703818743633));
#53761=CARTESIAN_POINT('Ctrl Pts',(-0.704558116518999,0.242372361471718,
-4.91118067686037));
#53762=CARTESIAN_POINT('Ctrl Pts',(-0.734734047924101,-0.123743201749595,
-4.89532316628444));
#53763=CARTESIAN_POINT('Ctrl Pts',(-0.586302646475458,-0.459777889740308,
-4.87946565570849));
#53764=CARTESIAN_POINT('Ctrl Pts',(-0.295346269863432,-0.684044649153792,
-4.86360814513255));
#53765=CARTESIAN_POINT('Ctrl Pts',(0.0674061663944642,-0.742026219139309,
-4.84775063455661));
#53766=CARTESIAN_POINT('Ctrl Pts',(0.413772761229021,-0.619627794101497,
-4.83189312398067));
#53767=CARTESIAN_POINT('Ctrl Pts',(0.659554866343183,-0.346603345975194,
-4.81603561340471));
#53768=CARTESIAN_POINT('Ctrl Pts',(0.745005031102745,0.0106773025514018,
-4.80017810282878));
#53769=CARTESIAN_POINT('Ctrl Pts',(0.649351078060994,0.365362393493366,
-4.78432059225283));
#53770=CARTESIAN_POINT('Ctrl Pts',(0.395845635128632,0.631231125902221,
-4.76846308167689));
#53771=CARTESIAN_POINT('Ctrl Pts',(0.0461136278878946,0.743653168137669,
-4.75260557110094));
#53772=CARTESIAN_POINT('Ctrl Pts',(-0.31482819344617,0.675299718472914,
-4.736748060525));
#53773=CARTESIAN_POINT('Ctrl Pts',(-0.599238072239317,0.44278689449563,
-4.72089054994906));
#53774=CARTESIAN_POINT('Ctrl Pts',(-0.737978488552156,0.102636502241902,
-4.70503303937312));
#53775=CARTESIAN_POINT('Ctrl Pts',(-0.697322877259977,-0.26246391372538,
-4.68917552879717));
#53776=CARTESIAN_POINT('Ctrl Pts',(-0.487154257012797,-0.563761679286988,
-4.67331801822123));
#53777=CARTESIAN_POINT('Ctrl Pts',(-0.15856275602498,-0.728013978959154,
-4.65746050764529));
#53778=CARTESIAN_POINT('Ctrl Pts',(0.208573945125506,-0.715292534962416,
-4.64160299706934));
#53779=CARTESIAN_POINT('Ctrl Pts',(0.525008169445223,-0.528689817543286,
-4.6257454864934));
#53780=CARTESIAN_POINT('Ctrl Pts',(0.713817562527057,-0.213567292875351,
-4.60988797591745));
#53781=CARTESIAN_POINT('Ctrl Pts',(0.729104234908342,0.153471547190018,
-4.59403046534152));
#53782=CARTESIAN_POINT('Ctrl Pts',(0.567152132065747,0.483202814821534,
-4.57817295476556));
#53783=CARTESIAN_POINT('Ctrl Pts',(0.267330374323152,0.695471762275377,
-4.56231544418963));
#53784=CARTESIAN_POINT('Ctrl Pts',(-0.0974770272500981,0.738677690414879,
-4.54645793361368));
#53785=CARTESIAN_POINT('Ctrl Pts',(-0.43858862773608,0.602317621175703,
-4.53060042303774));
#53786=CARTESIAN_POINT('Ctrl Pts',(-0.673083221372783,0.319539478413253,
-4.5147429124618));
#53787=CARTESIAN_POINT('Ctrl Pts',(-0.743957251490401,-0.0409158784950773,
-4.49888540188585));
#53788=CARTESIAN_POINT('Ctrl Pts',(-0.633981869740789,-0.391424948103911,
-4.48302789130991));
#53789=CARTESIAN_POINT('Ctrl Pts',(-0.369891116378875,-0.646782083226002,
-4.46717038073397));
#53790=CARTESIAN_POINT('Ctrl Pts',(-0.0158831121023146,-0.744912228325002,
-4.45131287015802));
#53791=CARTESIAN_POINT('Ctrl Pts',(0.341985935905684,-0.661960815155165,
-4.43545535958208));
#53792=CARTESIAN_POINT('Ctrl Pts',(0.616721234963047,-0.418092596805816,
-4.41959784900613));
#53793=CARTESIAN_POINT('Ctrl Pts',(0.741537069688743,-0.0725897750072806,
-4.40374033843019));
#53794=CARTESIAN_POINT('Ctrl Pts',(0.686091817285715,0.290558977510177,
-4.38788282785425));
#53795=CARTESIAN_POINT('Ctrl Pts',(0.463863727032172,0.58307541870842,-4.3720253172783));
#53796=CARTESIAN_POINT('Ctrl Pts',(0.128874477381027,0.733851395200652,
-4.35616780670236));
#53797=CARTESIAN_POINT('Ctrl Pts',(-0.237443015112518,0.706234603890558,
-4.34031029612642));
#53798=CARTESIAN_POINT('Ctrl Pts',(-0.546040215816375,0.506938441893474,
-4.32445278555047));
#53799=CARTESIAN_POINT('Ctrl Pts',(-0.721899881280921,0.18441003921904,
-4.30859527497453));
#53800=CARTESIAN_POINT('Ctrl Pts',(-0.72227208601418,-0.182946808998957,
-4.29273776439859));
#53801=CARTESIAN_POINT('Ctrl Pts',(-0.547066350345486,-0.505830909966805,
-4.27688025382264));
#53802=CARTESIAN_POINT('Ctrl Pts',(-0.23887363523123,-0.705752001449229,
-4.2610227432467));
#53803=CARTESIAN_POINT('Ctrl Pts',(0.127387142739609,-0.734111038619373,
-4.24516523267076));
#53804=CARTESIAN_POINT('Ctrl Pts',(0.46268123573258,-0.584014190974114,
-4.22930772209481));
#53805=CARTESIAN_POINT('Ctrl Pts',(0.685501622478843,-0.291948671408264,
-4.21345021151887));
#53806=CARTESIAN_POINT('Ctrl Pts',(0.741682642499434,0.0710869817423186,
-4.19759270094293));
#53807=CARTESIAN_POINT('Ctrl Pts',(0.617567187931678,0.416842019892833,
-4.18173519036698));
#53808=CARTESIAN_POINT('Ctrl Pts',(0.34332662536585,0.661266458754013,-4.16587767979104));
#53809=CARTESIAN_POINT('Ctrl Pts',(-0.014373595871744,0.744942884320598,
-4.15002016921509));
#53810=CARTESIAN_POINT('Ctrl Pts',(-0.36857972339009,0.647530299417611,
-4.13416265863915));
#53811=CARTESIAN_POINT('Ctrl Pts',(-0.633187388002473,0.392708839769087,
-4.11830514806321));
#53812=CARTESIAN_POINT('Ctrl Pts',(-0.743872812469215,0.0424233429530765,
-4.10244763748726));
#53813=CARTESIAN_POINT('Ctrl Pts',(-0.67372935144614,-0.318174892406895,
-4.08659012691132));
#53814=CARTESIAN_POINT('Ctrl Pts',(-0.439808258411777,-0.601427632380634,
-4.07073261633538));
#53815=CARTESIAN_POINT('Ctrl Pts',(-0.0989736771241871,-0.738478647216488,
-4.05487510575944));
#53816=CARTESIAN_POINT('Ctrl Pts',(0.265920527565673,-0.69601205031046,
-4.03901759518349));
#53817=CARTESIAN_POINT('Ctrl Pts',(0.566171809671833,-0.484351094858986,
-4.02316008460755));
#53818=CARTESIAN_POINT('Ctrl Pts',(0.728791744560353,-0.154948682533456,
-4.00730257403161));
#53819=CARTESIAN_POINT('Ctrl Pts',(0.714248867858033,0.212120380731541,
-3.99144506345566));
#53820=CARTESIAN_POINT('Ctrl Pts',(0.526078423953184,0.527624860112855,
-3.97558755287972));
#53821=CARTESIAN_POINT('Ctrl Pts',(0.210022979428513,0.714868413954726,
-3.95973004230377));
#53822=CARTESIAN_POINT('Ctrl Pts',(-0.157087189318767,0.728333794430896,
-3.94387253172783));
#53823=CARTESIAN_POINT('Ctrl Pts',(-0.486010855087196,0.564747686932481,
-3.92801502115189));
#53824=CARTESIAN_POINT('Ctrl Pts',(-0.696789590985629,0.263876423828005,
-3.91215751057594));
#53825=CARTESIAN_POINT('Ctrl Pts',(-0.738184955094202,-0.101140858364692,
-3.8963));
#53826=CARTESIAN_POINT('Ctrl Pts',(-0.600134101411932,-0.441571694609913,
-3.88044248942406));
#53827=CARTESIAN_POINT('Ctrl Pts',(-0.316195968501739,-0.674660366896873,
-3.86458497884811));
#53828=CARTESIAN_POINT('Ctrl Pts',(0.0446066009386007,-0.743745085570909,
-3.84872746827217));
#53829=CARTESIAN_POINT('Ctrl Pts',(0.394565701175593,-0.632031968031671,
-3.83286995769623));
#53830=CARTESIAN_POINT('Ctrl Pts',(0.648609377700225,-0.366677482697674,
-3.81701244712028));
#53831=CARTESIAN_POINT('Ctrl Pts',(0.744981865115991,-0.0121869523046585,
-3.80115493654434));
#53832=CARTESIAN_POINT('Ctrl Pts',(0.660255866176431,0.345266118143364,
-3.7852974259684));
#53833=CARTESIAN_POINT('Ctrl Pts',(0.415027520037911,0.618788056421063,
-3.76943991539245));
#53834=CARTESIAN_POINT('Ctrl Pts',(0.0689096634373234,0.741888104395219,
-3.75358240481651));
#53835=CARTESIAN_POINT('Ctrl Pts',(-0.293959521387625,0.684641731815797,
-3.73772489424057));
#53836=CARTESIAN_POINT('Ctrl Pts',(-0.585369752826176,0.460965024307049,
-3.72186738366462));
#53837=CARTESIAN_POINT('Ctrl Pts',(-0.734481787276393,0.125231806333102,
-3.70600987308868));
#53838=CARTESIAN_POINT('Ctrl Pts',(-0.705047811199764,-0.240944153447636,
-3.69015236251273));
#53839=CARTESIAN_POINT('Ctrl Pts',(-0.504222963217104,-0.548548725750719,
-3.67429485193679));
#53840=CARTESIAN_POINT('Ctrl Pts',(-0.180825983347723,-0.722805966290058,
-3.65843734136085));
#53841=CARTESIAN_POINT('Ctrl Pts',(0.186528189859359,-0.721355484865796,
-3.64257983078491));
#53842=CARTESIAN_POINT('Ctrl Pts',(0.508539013881873,-0.544549880652111,
-3.62672232020896));
#53843=CARTESIAN_POINT('Ctrl Pts',(0.706928512367425,-0.235369028464147,
-3.61086480963302));
#53844=CARTESIAN_POINT('Ctrl Pts',(0.733469957167495,0.131027947747378,
-3.59500729905708));
#53845=CARTESIAN_POINT('Ctrl Pts',(0.581711358369246,0.465573191563243,
-3.57914978848113));
#53846=CARTESIAN_POINT('Ctrl Pts',(0.288543885839595,0.686941720310219,
-3.56329227790519));
#53847=CARTESIAN_POINT('Ctrl Pts',(-0.0747660470900795,0.741320807316712,
-3.54743476732925));
#53848=CARTESIAN_POINT('Ctrl Pts',(-0.419901016852458,0.615491378659723,
-3.5315772567533));
#53849=CARTESIAN_POINT('Ctrl Pts',(-0.662961772285872,0.340041452834431,
-3.51571974617736));
#53850=CARTESIAN_POINT('Ctrl Pts',(-0.744862398735852,-0.0180695353467789,
-3.49986223560141));
#53851=CARTESIAN_POINT('Ctrl Pts',(-0.645693580048323,-0.371787979690786,
-3.48400472502547));
#53852=CARTESIAN_POINT('Ctrl Pts',(-0.389562376809465,-0.635128062466725,
-3.46814721444952));
#53853=CARTESIAN_POINT('Ctrl Pts',(-0.0387320136518709,-0.744074144340904,
-3.45228970387359));
#53854=CARTESIAN_POINT('Ctrl Pts',(0.321513758624112,-0.672142398732272,
-3.43643219329764));
#53855=CARTESIAN_POINT('Ctrl Pts',(0.603602386739046,-0.436818795247073,
-3.4205746827217));
#53856=CARTESIAN_POINT('Ctrl Pts',(0.738960626213063,-0.0953084154992266,
-3.40471717214575));
#53857=CARTESIAN_POINT('Ctrl Pts',(0.69468408912439,0.26937059504629,-3.38885966156981));
#53858=CARTESIAN_POINT('Ctrl Pts',(0.481536009080821,0.568568002192077,
-3.37300215099387));
#53859=CARTESIAN_POINT('Ctrl Pts',(0.151330794557152,0.729551568963344,
-3.35714464041793));
#53860=CARTESIAN_POINT('Ctrl Pts',(-0.215661594415367,0.713187617568055,
-3.34128712984198));
#53861=CARTESIAN_POINT('Ctrl Pts',(-0.530228561854279,0.523454079506617,
-3.32542961926604));
#53862=CARTESIAN_POINT('Ctrl Pts',(-0.715901666944983,0.206473495692717,
-3.30957210869009));
#53863=CARTESIAN_POINT('Ctrl Pts',(-0.727545424028934,-0.160698964317554,
-3.29371459811415));
#53864=CARTESIAN_POINT('Ctrl Pts',(-0.56232933899328,-0.488806930868986,
-3.27785708753821));
#53865=CARTESIAN_POINT('Ctrl Pts',(-0.260415977294363,-0.698090266318044,
-3.26199957696227));
#53866=CARTESIAN_POINT('Ctrl Pts',(0.104802199620971,-0.737674047335801,
-3.24614206638632));
#53867=CARTESIAN_POINT('Ctrl Pts',(0.4445438909911,-0.597935807709044,-3.23028455581038));
#53868=CARTESIAN_POINT('Ctrl Pts',(0.67622090381438,-0.312844674563337,
-3.21442704523443));
#53869=CARTESIAN_POINT('Ctrl Pts',(0.743514610335906,0.0482962252688744,
-3.19856953465849));
#53870=CARTESIAN_POINT('Ctrl Pts',(0.630066507130376,0.397696740935482,
-3.18271202408254));
#53871=CARTESIAN_POINT('Ctrl Pts',(0.363454822249294,0.650420704884086,
-3.16685451350661));
#53872=CARTESIAN_POINT('Ctrl Pts',(0.00849049249189266,0.745033162144761,
-3.15099700293066));
#53873=CARTESIAN_POINT('Ctrl Pts',(-0.348537800713067,0.65853466319722,
-3.13513949235472));
#53874=CARTESIAN_POINT('Ctrl Pts',(-0.620839644721946,0.411952226234673,
-3.11928198177877));
#53875=CARTESIAN_POINT('Ctrl Pts',(-0.742220875500842,0.0652278554678893,
-3.10342447120283));
#53876=CARTESIAN_POINT('Ctrl Pts',(-0.683174792020755,-0.297352828649017,
-3.08756696062688));
#53877=CARTESIAN_POINT('Ctrl Pts',(-0.458054973669544,-0.587649676469553,
-3.07170945005094));
#53878=CARTESIAN_POINT('Ctrl Pts',(-0.121586052362424,-0.735094098077993,
-3.055851939475));
#53879=CARTESIAN_POINT('Ctrl Pts',(0.244439360284691,-0.703843661832503,
-3.03999442889905));
#53880=CARTESIAN_POINT('Ctrl Pts',(0.551043731660782,-0.5014950717161,-3.02413691832311));
#53881=CARTESIAN_POINT('Ctrl Pts',(0.723694257457264,-0.177237475951216,
-3.00827940774717));
#53882=CARTESIAN_POINT('Ctrl Pts',(0.720421125583033,0.190104978819204,
-2.99242189717122));
#53883=CARTESIAN_POINT('Ctrl Pts',(0.542020005376938,0.511234598720941,
-2.97656438659528));
#53884=CARTESIAN_POINT('Ctrl Pts',(0.23185862744593,0.708087620310554,-2.96070687601934));
#53885=CARTESIAN_POINT('Ctrl Pts',(-0.134665527144535,0.732810819350438,
-2.9448493654434));
#53886=CARTESIAN_POINT('Ctrl Pts',(-0.468453686038892,0.579394205351375,
-2.92899185486745));
#53887=CARTESIAN_POINT('Ctrl Pts',(-0.688364907195973,0.285131996975536,
-2.91313434429151));
#53888=CARTESIAN_POINT('Ctrl Pts',(-0.740940722498702,-0.0784432718674888,
-2.89727683371556));
#53889=CARTESIAN_POINT('Ctrl Pts',(-0.613400417387355,-0.42294967680233,
-2.88141932313962));
#53890=CARTESIAN_POINT('Ctrl Pts',(-0.336747909254422,-0.664640765203995,
-2.86556181256368));
#53891=CARTESIAN_POINT('Ctrl Pts',(0.0217650299908832,-0.744763576329879,
-2.84970430198774));
#53892=CARTESIAN_POINT('Ctrl Pts',(0.374987083415478,-0.643840965168983,
-2.83384679141179));
#53893=CARTESIAN_POINT('Ctrl Pts',(0.637053101519986,-0.386406323708533,
-2.81798928083585));
#53894=CARTESIAN_POINT('Ctrl Pts',(0.744257158796397,-0.0350397308564244,
-2.80213177025991));
#53895=CARTESIAN_POINT('Ctrl Pts',(0.670538899398487,0.324844709902505,
-2.78627425968396));
#53896=CARTESIAN_POINT('Ctrl Pts',(0.43381857859533,0.605762281777021,-2.77041674910802));
#53897=CARTESIAN_POINT('Ctrl Pts',(0.0916408075974612,0.739424413676653,
-2.75455923853207));
#53898=CARTESIAN_POINT('Ctrl Pts',(-0.272814031234396,0.693339026393159,
-2.73870172795613));
#53899=CARTESIAN_POINT('Ctrl Pts',(-0.570950197858908,0.478709068979323,
-2.72284421738019));
#53900=CARTESIAN_POINT('Ctrl Pts',(-0.730293433462981,0.147709181160235,
-2.70698670680424));
#53901=CARTESIAN_POINT('Ctrl Pts',(-0.71210881021805,-0.219197499000354,
-2.6911291962283));
#53902=CARTESIAN_POINT('Ctrl Pts',(-0.520816848808986,-0.532819210572265,
-2.67527168565235));
#53903=CARTESIAN_POINT('Ctrl Pts',(-0.202918929048214,-0.716917296061479,
-2.65941417507642));
#53904=CARTESIAN_POINT('Ctrl Pts',(0.164306783272657,-0.726739143110351,
-2.64355666450047));
#53905=CARTESIAN_POINT('Ctrl Pts',(0.491590973333846,-0.559897147782392,
-2.62769915392453));
#53906=CARTESIAN_POINT('Ctrl Pts',(0.699373756252946,-0.256949119910581,
-2.61184164334858));
#53907=CARTESIAN_POINT('Ctrl Pts',(0.737144979717066,0.10846096088502,-2.59598413277264));
#53908=CARTESIAN_POINT('Ctrl Pts',(0.595722794184041,0.447505143710925,
-2.5801266221967));
#53909=CARTESIAN_POINT('Ctrl Pts',(0.309485679099278,0.677764793708433,
-2.56426911162075));
#53910=CARTESIAN_POINT('Ctrl Pts',(-0.0519846606557266,0.743265831459165,
-2.54841160104481));
#53911=CARTESIAN_POINT('Ctrl Pts',(-0.400817990304477,0.628085535422093,
-2.53255409046887));
#53912=CARTESIAN_POINT('Ctrl Pts',(-0.65221602018681,0.360223214368335,
-2.51669657989292));
#53913=CARTESIAN_POINT('Ctrl Pts',(-0.745066118148496,0.00479382366248841,
-2.50083906931698));
#53914=CARTESIAN_POINT('Ctrl Pts',(-0.656797248589648,-0.351800903073378,
-2.48498155874103));
#53915=CARTESIAN_POINT('Ctrl Pts',(-0.408866791102873,-0.622875949360237,
-2.4691240481651));
#53916=CARTESIAN_POINT('Ctrl Pts',(-0.0615444417367415,-0.742535374813543,
-2.45326653758914));
#53917=CARTESIAN_POINT('Ctrl Pts',(0.30073881575884,-0.681691034013317,
-2.43740902701321));
#53918=CARTESIAN_POINT('Ctrl Pts',(0.589915133512018,-0.455133646758482,
-2.42155151643726));
#53919=CARTESIAN_POINT('Ctrl Pts',(0.735688312531754,-0.117937305219158,
-2.40569400586132));
#53920=CARTESIAN_POINT('Ctrl Pts',(0.702622185432192,0.247928549579643,
-2.38983649528537));
#53921=CARTESIAN_POINT('Ctrl Pts',(0.498754834544953,0.553525172125181,
-2.37397898470943));
#53922=CARTESIAN_POINT('Ctrl Pts',(0.173644605370432,0.72456473291482,-2.35812147413349));
#53923=CARTESIAN_POINT('Ctrl Pts',(-0.193677087826048,0.719469031167705,
-2.34226396355754));
#53924=CARTESIAN_POINT('Ctrl Pts',(-0.513917598124815,0.539476786799764,
-2.3264064529816));
#53925=CARTESIAN_POINT('Ctrl Pts',(-0.709229296744016,0.228342518594689,
-2.31054894240566));
#53926=CARTESIAN_POINT('Ctrl Pts',(-0.732133641394678,-0.138299791382143,
-2.29469143182972));
#53927=CARTESIAN_POINT('Ctrl Pts',(-0.577062788963539,-0.471322648248307,
-2.27883392125377));
#53928=CARTESIAN_POINT('Ctrl Pts',(-0.28171308880903,-0.689771148100477,
-2.26297641067783));
#53929=CARTESIAN_POINT('Ctrl Pts',(0.0821185655496305,-0.740542397402233,
-2.24711890010188));
#53930=CARTESIAN_POINT('Ctrl Pts',(0.425987924691361,-0.611294355589289,
-2.23126138952594));
#53931=CARTESIAN_POINT('Ctrl Pts',(0.66630339617538,-0.333446075705398,
-2.21540387895));
#53932=CARTESIAN_POINT('Ctrl Pts',(0.744646419535463,0.025459988829357,
-2.19954636837405));
#53933=CARTESIAN_POINT('Ctrl Pts',(0.641972500386766,0.3781769558095,-2.18368885779811));
#53934=CARTESIAN_POINT('Ctrl Pts',(0.383240758161146,0.638962457772165,
-2.16783134722217));
#53935=CARTESIAN_POINT('Ctrl Pts',(0.0313465854623456,0.744421851330298,
-2.15197383664622));
#53936=CARTESIAN_POINT('Ctrl Pts',(-0.328167664241619,0.668918892919293,
-2.13611632607028));
#53937=CARTESIAN_POINT('Ctrl Pts',(-0.607907264322853,0.430807682315068,
-2.12025881549434));
#53938=CARTESIAN_POINT('Ctrl Pts',(-0.739869998189859,0.0879709437070718,
-2.10440130491839));
#53939=CARTESIAN_POINT('Ctrl Pts',(-0.691976895229164,-0.276250751360397,
-2.08854379434245));
#53940=CARTESIAN_POINT('Ctrl Pts',(-0.475870344147353,-0.573318338028059,
-2.0726862837665));
#53941=CARTESIAN_POINT('Ctrl Pts',(-0.144083931498636,-0.731017319796236,
-2.05682877319056));
#53942=CARTESIAN_POINT('Ctrl Pts',(0.222728007440529,-0.711012472365815,
-2.04097126261462));
#53943=CARTESIAN_POINT('Ctrl Pts',(0.535396742490916,-0.51816679678294,
-2.02511375203868));
#53944=CARTESIAN_POINT('Ctrl Pts',(0.717915276301731,-0.199359367000361,
-2.00925624146273));
#53945=CARTESIAN_POINT('Ctrl Pts',(0.725914971523952,0.167910557367775,
-1.99339873088679));
#53946=CARTESIAN_POINT('Ctrl Pts',(0.557451173174836,0.494362913944983,
-1.97754122031085));
#53947=CARTESIAN_POINT('Ctrl Pts',(0.253475937022809,0.700640029193726,
-1.9616837097349));
#53948=CARTESIAN_POINT('Ctrl Pts',(-0.112117052086442,0.736597765262441,
-1.94582619915896));
#53949=CARTESIAN_POINT('Ctrl Pts',(-0.450455379870058,0.593495115316291,
-1.92996868858302));
#53950=CARTESIAN_POINT('Ctrl Pts',(-0.679291998571966,0.306119064800417,
-1.91411117800707));
#53951=CARTESIAN_POINT('Ctrl Pts',(-0.74299875506506,-0.0556718162982561,
-1.89825366743113));
#53952=CARTESIAN_POINT('Ctrl Pts',(-0.626089101673838,-0.40392937244452,
-1.88239615685519));
#53953=CARTESIAN_POINT('Ctrl Pts',(-0.356982738609634,-0.653995279411816,
-1.86653864627924));
#53954=CARTESIAN_POINT('Ctrl Pts',(-0.00109703682003259,-0.745080732315894,
-1.8506811357033));
#53955=CARTESIAN_POINT('Ctrl Pts',(0.355055344894126,-0.655043665124921,
-1.83482362512736));
#53956=CARTESIAN_POINT('Ctrl Pts',(0.624896920206737,-0.405771290598917,
-1.81896611455141));
#53957=CARTESIAN_POINT('Ctrl Pts',(0.742831594591062,-0.0578595129211745,
-1.80310860397547));
#53958=CARTESIAN_POINT('Ctrl Pts',(0.680190494320244,0.304117399361759,
-1.78725109339952));
#53959=CARTESIAN_POINT('Ctrl Pts',(0.452201115490324,0.592166068183142,
-1.77139358282358));
#53960=CARTESIAN_POINT('Ctrl Pts',(0.114285654727207,0.73626441600946,-1.75553607224764));
#53961=CARTESIAN_POINT('Ctrl Pts',(-0.251411635436553,0.701383412068814,
-1.73967856167169));
#53962=CARTESIAN_POINT('Ctrl Pts',(-0.555992986056486,0.496002319162088,
-1.72382105109575));
#53963=CARTESIAN_POINT('Ctrl Pts',(-0.7254173712336,0.170047460053681,-1.70796354051981));
#53964=CARTESIAN_POINT('Ctrl Pts',(-0.718499225058212,-0.197244428942686,
-1.69210602994386));
#53965=CARTESIAN_POINT('Ctrl Pts',(-0.53692028752885,-0.51658794604415,
-1.67624851936792));
#53966=CARTESIAN_POINT('Ctrl Pts',(-0.224820788469039,-0.710353513562321,
-1.66039100879198));
#53967=CARTESIAN_POINT('Ctrl Pts',(0.141930650992857,-0.731438439970802,
-1.64453349821603));
#53968=CARTESIAN_POINT('Ctrl Pts',(0.474180007564145,-0.574717166599923,
-1.62867598764009));
#53969=CARTESIAN_POINT('Ctrl Pts',(0.691160408405278,-0.278287245505838,
-1.61281847706415));
#53970=CARTESIAN_POINT('Ctrl Pts',(0.740125841833161,0.0857918376591303,
-1.59696096648821));
#53971=CARTESIAN_POINT('Ctrl Pts',(0.609173245111979,0.429015685724797,
-1.58110345591226));
#53972=CARTESIAN_POINT('Ctrl Pts',(0.330136033470989,0.667949624269838,
-1.56524594533632));
#53973=CARTESIAN_POINT('Ctrl Pts',(-0.0291543209007144,0.744510931236738,
-1.54938843476037));
#53974=CARTESIAN_POINT('Ctrl Pts',(-0.38135751834543,0.640088231699029,
-1.53353092418443));
#53975=CARTESIAN_POINT('Ctrl Pts',(-0.640856084219246,0.380065758096348,
-1.51767341360849));
#53976=CARTESIAN_POINT('Ctrl Pts',(-0.744568217888247,0.0276526683864981,
-1.50181590303254));
#53977=CARTESIAN_POINT('Ctrl Pts',(-0.667282419175575,-0.331482539837873,
-1.4859583924566));
#53978=CARTESIAN_POINT('Ctrl Pts',(-0.4277861805277,-0.610037281571953,
-1.47010088188066));
#53979=CARTESIAN_POINT('Ctrl Pts',(-0.0842989141717446,-0.74029736878341,
-1.45424337130471));
#53980=CARTESIAN_POINT('Ctrl Pts',(0.27968067082008,-0.690597729164966,
-1.43838586072877));
#53981=CARTESIAN_POINT('Ctrl Pts',(0.575672364401323,-0.473019904467842,
-1.42252835015283));
#53982=CARTESIAN_POINT('Ctrl Pts',(0.731723210142681,-0.140455134817732,
-1.40667083957688));
#53983=CARTESIAN_POINT('Ctrl Pts',(0.709898631000685,0.226253032822831,
-1.39081332900094));
#53984=CARTESIAN_POINT('Ctrl Pts',(0.515503988666716,0.537961094157267,
-1.37495581842499));
#53985=CARTESIAN_POINT('Ctrl Pts',(0.195794897177476,0.718895583097738,
-1.35909830784905));
#53986=CARTESIAN_POINT('Ctrl Pts',(-0.17151019788618,0.725072929558965,
-1.34324079727311));
#53987=CARTESIAN_POINT('Ctrl Pts',(-0.497122684463518,0.554991475384949,
-1.32738328669717));
#53988=CARTESIAN_POINT('Ctrl Pts',(-0.701889053967625,0.249996514132912,
-1.31152577612122));
#53989=CARTESIAN_POINT('Ctrl Pts',(-0.736032417443101,-0.115770383220588,
-1.29566826554528));
#53990=CARTESIAN_POINT('Ctrl Pts',(-0.591252825946184,-0.453394526840398,
-1.27981075496934));
#53991=CARTESIAN_POINT('Ctrl Pts',(-0.302744914545142,-0.680802480808663,
-1.26395324439339));
#53992=CARTESIAN_POINT('Ctrl Pts',(0.0593576014270612,-0.742713387728404,
-1.24809573381745));
#53993=CARTESIAN_POINT('Ctrl Pts',(0.407030810760431,-0.624077255033285,
-1.2322382232415));
#53994=CARTESIAN_POINT('Ctrl Pts',(0.655758438757783,-0.353733474746353,
-1.21638071266556));
#53995=CARTESIAN_POINT('Ctrl Pts',(0.745077004287191,0.00259977702898679,
-1.20052320208962));
#53996=CARTESIAN_POINT('Ctrl Pts',(0.653273955972268,0.358301046058368,
-1.18466569151367));
#53997=CARTESIAN_POINT('Ctrl Pts',(0.402665800926975,0.626902507509751,
-1.16880818093773));
#53998=CARTESIAN_POINT('Ctrl Pts',(0.0541731597357335,0.743109527541145,
-1.15295067036179));
#53999=CARTESIAN_POINT('Ctrl Pts',(-0.307488496284748,0.678673209881398,
-1.13709315978584));
#54000=CARTESIAN_POINT('Ctrl Pts',(-0.594402425070052,0.449257452057301,
-1.1212356492099));
#54001=CARTESIAN_POINT('Ctrl Pts',(-0.736822394328756,0.110631190781873,
-1.10537813863396));
#54002=CARTESIAN_POINT('Ctrl Pts',(-0.700127372238149,-0.254888532109785,
-1.08952062805801));
#54003=CARTESIAN_POINT('Ctrl Pts',(-0.493237593328167,-0.558447112702729,
-1.07366311748207));
#54004=CARTESIAN_POINT('Ctrl Pts',(-0.166446128554507,-0.72625215142359,
-1.05780560690613));
#54005=CARTESIAN_POINT('Ctrl Pts',(0.200806914349289,-0.717511731128971,
-1.04194809633018));
#54006=CARTESIAN_POINT('Ctrl Pts',(0.519245576741049,-0.534350570499398,
-1.02609058575424));
#54007=CARTESIAN_POINT('Ctrl Pts',(0.711460243089813,-0.221293523765969,
-1.0102330751783));
#54008=CARTESIAN_POINT('Ctrl Pts',(0.730725232193086,0.145558016593173,
-0.994375564602353));
#54009=CARTESIAN_POINT('Ctrl Pts',(0.572357396004417,0.477025693644712,
-0.978518054026409));
#54010=CARTESIAN_POINT('Ctrl Pts',(0.274854551402442,0.692532653909937,
-0.962660543450467));
#54011=CARTESIAN_POINT('Ctrl Pts',(-0.0894629977683567,0.73969106604614,
-0.946803032874522));
#54012=CARTESIAN_POINT('Ctrl Pts',(-0.432032885366019,0.607037138172358,
-0.930945522298579));
#54013=CARTESIAN_POINT('Ctrl Pts',(-0.669579408960958,0.326817864036942,
-0.915088011722637));
#54014=CARTESIAN_POINT('Ctrl Pts',(-0.744357114769118,-0.0328479352588572,
-0.899230501146692));
#54015=CARTESIAN_POINT('Ctrl Pts',(-0.638188205492206,-0.384528692725023,
-0.88337299057075));
#54016=CARTESIAN_POINT('Ctrl Pts',(-0.376881401675451,-0.64273393424443,
-0.867515479994806));
#54017=CARTESIAN_POINT('Ctrl Pts',(-0.0239580705647442,-0.744696254867037,
-0.851657969418863));
#54018=CARTESIAN_POINT('Ctrl Pts',(0.334789255086544,-0.665629518453601,
-0.835800458842918));
#54019=CARTESIAN_POINT('Ctrl Pts',(0.612152281088124,-0.424754147615751,
-0.819942948266977));
#54020=CARTESIAN_POINT('Ctrl Pts',(0.740706514936408,-0.0806248093885304,
-0.804085437691032));
#54021=CARTESIAN_POINT('Ctrl Pts',(0.68920156215251,0.283103705176595,-0.788227927115088));
#54022=CARTESIAN_POINT('Ctrl Pts',(0.470157820112161,0.5780122190279,-0.772370416539146));
#54023=CARTESIAN_POINT('Ctrl Pts',(0.136822880450277,0.732411087124892,
-0.756512905963202));
#54024=CARTESIAN_POINT('Ctrl Pts',(-0.229772488369119,0.708767313542914,
-0.740655395387258));
#54025=CARTESIAN_POINT('Ctrl Pts',(-0.54051220244279,0.512828490012617,
-0.724797884811315));
#54026=CARTESIAN_POINT('Ctrl Pts',(-0.719858192316569,0.192225607328728,
-0.708940374235372));
#54027=CARTESIAN_POINT('Ctrl Pts',(-0.724213037944555,-0.175105616212887,
-0.693082863659428));
#54028=CARTESIAN_POINT('Ctrl Pts',(-0.552518114964911,-0.499870216950158,
-0.677225353083484));
#54029=CARTESIAN_POINT('Ctrl Pts',(-0.246510936896401,-0.703120799826482,
-0.661367842507542));
#54030=CARTESIAN_POINT('Ctrl Pts',(0.119420864350713,-0.735448950176627,
-0.645510331931598));
#54031=CARTESIAN_POINT('Ctrl Pts',(0.456322512266791,-0.588995981273811,
-0.629652821355655));
#54032=CARTESIAN_POINT('Ctrl Pts',(0.682296203233876,-0.299363311397401,
-0.613795310779712));
#54033=CARTESIAN_POINT('Ctrl Pts',(0.742409736474291,0.0630419253064556,
-0.597937800203768));
#54034=CARTESIAN_POINT('Ctrl Pts',(0.622050045027544,0.41012222890184,-0.582080289627824));
#54035=CARTESIAN_POINT('Ctrl Pts',(0.350475502767979,0.657505454819733,
-0.566222779051882));
#54036=CARTESIAN_POINT('Ctrl Pts',(-0.00629652687738437,0.745054934154154,
-0.550365268475936));
#54037=CARTESIAN_POINT('Ctrl Pts',(-0.361537926664331,0.651488164697928,
-0.534507757899994));
#54038=CARTESIAN_POINT('Ctrl Pts',(-0.628892661896185,0.39955039853715,
-0.51865024732405));
#54039=CARTESIAN_POINT('Ctrl Pts',(-0.743369166821858,0.0504854729301265,
-0.502792736748107));
#54040=CARTESIAN_POINT('Ctrl Pts',(-0.677139218048598,-0.310852023539114,
-0.486935226172163));
#54041=CARTESIAN_POINT('Ctrl Pts',(-0.446302728926307,-0.596624149118552,
-0.47107771559622));
#54042=CARTESIAN_POINT('Ctrl Pts',(-0.10697400334667,-0.737362233753777,
-0.455220205020277));
#54043=CARTESIAN_POINT('Ctrl Pts',(0.258359154003842,-0.698854096860472,
-0.439362694444332));
#54044=CARTESIAN_POINT('Ctrl Pts',(0.560887491653129,-0.490460725105599,
-0.42350518386839));
#54045=CARTESIAN_POINT('Ctrl Pts',(0.727069052926082,-0.162840699527328,
-0.407647673292446));
#54046=CARTESIAN_POINT('Ctrl Pts',(0.716506573706083,0.204364456341259,
-0.391790162716503));
#54047=CARTESIAN_POINT('Ctrl Pts',(0.531767698940294,0.521890424799043,
-0.375932652140559));
#54048=CARTESIAN_POINT('Ctrl Pts',(0.217760811380721,0.712549458064953,
-0.360075141564617));
#54049=CARTESIAN_POINT('Ctrl Pts',(-0.149181799006659,0.729994035651059,
-0.344217630988673));
#54050=CARTESIAN_POINT('Ctrl Pts',(-0.479859636199047,0.569983535206768,
-0.328360120412729));
#54051=CARTESIAN_POINT('Ctrl Pts',(-0.693887851295182,0.27141509112605,
-0.312502609836787));
#54052=CARTESIAN_POINT('Ctrl Pts',(-0.73923807984108,-0.0931319557401305,
-0.296645099260842));
#54053=CARTESIAN_POINT('Ctrl Pts',(-0.604886089121433,-0.435039448872488,
-0.280787588684899));
#54054=CARTESIAN_POINT('Ctrl Pts',(-0.323491645640655,-0.671192711037537,
-0.264930078108956));
#54055=CARTESIAN_POINT('Ctrl Pts',(0.0365407342377404,-0.74418497214044,
-0.249072567533012));
#54056=CARTESIAN_POINT('Ctrl Pts',(0.387690414045755,-0.636272472016097,
-0.233215056957068));
#54057=CARTESIAN_POINT('Ctrl Pts',(0.64459593589752,-0.373687760499387,
-0.217357546381126));
#54058=CARTESIAN_POINT('Ctrl Pts',(0.744806009371733,-0.0202628962177233,
-0.201500035805182));
#54059=CARTESIAN_POINT('Ctrl Pts',(0.663960133248361,0.338087754507852,
-0.185642525229238));
#54060=CARTESIAN_POINT('Ctrl Pts',(0.421711850082436,0.614252160152718,
-0.169785014653295));
#54061=CARTESIAN_POINT('Ctrl Pts',(0.0769483449333087,0.741097525544364,
-0.153927504077352));
#54062=CARTESIAN_POINT('Ctrl Pts',(-0.286519037709493,0.687788235191209,
-0.138069993501407));
#54063=CARTESIAN_POINT('Ctrl Pts',(-0.580339275444648,0.46728453937117,
-0.122212482925465));
#54064=CARTESIAN_POINT('Ctrl Pts',(-0.733078137321275,0.133186519459017,
-0.106354972349522));
#54065=CARTESIAN_POINT('Ctrl Pts',(-0.707624014265837,-0.233284843518718,
-0.0904974617735782));
#54066=CARTESIAN_POINT('Ctrl Pts',(-0.510129659904911,-0.543052839296335,
-0.0746399511976345));
#54067=CARTESIAN_POINT('Ctrl Pts',(-0.188672782786423,-0.720797397637529,
-0.058782440621692));
#54068=CARTESIAN_POINT('Ctrl Pts',(0.178741094754426,-0.723347949753151,
-0.0429249300457477));
#54069=CARTESIAN_POINT('Ctrl Pts',(0.394571264335502,-0.607775493600903,
-0.0323532563284519));
#54070=CARTESIAN_POINT('Ctrl Pts',(0.482201081976437,-0.527701441143757,
-0.0270674194698041));
#54071=CARTESIAN_POINT('Ctrl Pts',(0.392888236737257,-0.550964357679777,
-5.8089));
#54072=CARTESIAN_POINT('Ctrl Pts',(0.484381081792765,-0.485721548291323,
-5.80361416314135));
#54073=CARTESIAN_POINT('Ctrl Pts',(0.634146933675295,-0.308844853941977,
-5.79304248942406));
#54074=CARTESIAN_POINT('Ctrl Pts',(0.70461890056211,0.0317634872067408,
-5.77718497884811));
#54075=CARTESIAN_POINT('Ctrl Pts',(0.603809517943593,0.364559903875637,
-5.76132746827217));
#54076=CARTESIAN_POINT('Ctrl Pts',(0.356217202446025,0.608779534529828,
-5.74546995769622));
#54077=CARTESIAN_POINT('Ctrl Pts',(0.0220327184609351,0.704987657002684,
-5.72961244712028));
#54078=CARTESIAN_POINT('Ctrl Pts',(-0.317508269912238,0.629831081602948,
-5.71375493654434));
#54079=CARTESIAN_POINT('Ctrl Pts',(-0.5798655339509,0.401562243999013,-5.6978974259684));
#54080=CARTESIAN_POINT('Ctrl Pts',(-0.701262770546561,0.0756802099782287,
-5.68203991539245));
#54081=CARTESIAN_POINT('Ctrl Pts',(-0.652189172010462,-0.268600560210128,
-5.66618240481651));
#54082=CARTESIAN_POINT('Ctrl Pts',(-0.444574205494435,-0.547586123312261,
-5.65032489424056));
#54083=CARTESIAN_POINT('Ctrl Pts',(-0.128887172109694,-0.69345876028638,
-5.63446738366463));
#54084=CARTESIAN_POINT('Ctrl Pts',(0.218131180300111,-0.670757513336377,
-5.61860987308867));
#54085=CARTESIAN_POINT('Ctrl Pts',(0.512123781755499,-0.485001168094135,
-5.60275236251274));
#54086=CARTESIAN_POINT('Ctrl Pts',(0.681623629821306,-0.181345284572452,
-5.58689485193679));
#54087=CARTESIAN_POINT('Ctrl Pts',(0.685426818106913,0.166394001985959,
-5.57103734136085));
#54088=CARTESIAN_POINT('Ctrl Pts',(0.522608823274475,0.47368439616164,-5.5551798307849));
#54089=CARTESIAN_POINT('Ctrl Pts',(0.232749257329435,0.665826306056506,
-5.53932232020896));
#54090=CARTESIAN_POINT('Ctrl Pts',(-0.113689589679385,0.69611174793571,
-5.52346480963302));
#54091=CARTESIAN_POINT('Ctrl Pts',(-0.432491505325853,0.557178593751515,
-5.50760729905708));
#54092=CARTESIAN_POINT('Ctrl Pts',(-0.646158570569616,0.28280026438264,
-5.49174978848113));
#54093=CARTESIAN_POINT('Ctrl Pts',(-0.70275021616536,-0.0603243024334685,
-5.47589227790519));
#54094=CARTESIAN_POINT('Ctrl Pts',(-0.588509514849396,-0.388784565910968,
-5.46003476732924));
#54095=CARTESIAN_POINT('Ctrl Pts',(-0.331207368228394,-0.622734748534038,
-5.4441772567533));
#54096=CARTESIAN_POINT('Ctrl Pts',(0.00660835310116418,-0.705303634925465,
-5.42831974617736));
#54097=CARTESIAN_POINT('Ctrl Pts',(0.342817642383509,-0.616419460965605,
-5.41246223560141));
#54098=CARTESIAN_POINT('Ctrl Pts',(0.595691002243588,-0.377689181239748,
-5.39660472502547));
#54099=CARTESIAN_POINT('Ctrl Pts',(0.703757160891212,-0.0471460101786735,
-5.38074721444953));
#54100=CARTESIAN_POINT('Ctrl Pts',(0.64074619327961,0.294857937962055,-5.36488970387358));
#54101=CARTESIAN_POINT('Ctrl Pts',(0.421975506976434,0.565184535610204,
-5.34903219329764));
#54102=CARTESIAN_POINT('Ctrl Pts',(0.100626316187652,0.698119783613068,
-5.3331746827217));
#54103=CARTESIAN_POINT('Ctrl Pts',(-0.245184239907299,0.661348301791295,
-5.31731717214575));
#54104=CARTESIAN_POINT('Ctrl Pts',(-0.531392681099133,0.463808911358507,
-5.30145966156981));
#54105=CARTESIAN_POINT('Ctrl Pts',(-0.688424272875483,0.153521686732225,
-5.28560215099387));
#54106=CARTESIAN_POINT('Ctrl Pts',(-0.678106027527137,-0.194085298805999,
-5.26974464041792));
#54107=CARTESIAN_POINT('Ctrl Pts',(-0.502946219016085,-0.49451186897655,
-5.25388712984198));
#54108=CARTESIAN_POINT('Ctrl Pts',(-0.205524643813888,-0.674726988171084,
-5.23802961926603));
#54109=CARTESIAN_POINT('Ctrl Pts',(0.141858150105515,-0.690921958711615,
-5.2221721086901));
#54110=CARTESIAN_POINT('Ctrl Pts',(0.454756485457226,-0.539159926845312,
-5.20631459811414));
#54111=CARTESIAN_POINT('Ctrl Pts',(0.65710755109285,-0.256332896987509,
-5.19045708753821));
#54112=CARTESIAN_POINT('Ctrl Pts',(0.699721597013181,0.0888063874649557,
-5.17459957696226));
#54113=CARTESIAN_POINT('Ctrl Pts',(0.572239526473699,0.412357626487503,
-5.15874206638632));
#54114=CARTESIAN_POINT('Ctrl Pts',(0.30565110055879,0.635668382498652,-5.14288455581037));
#54115=CARTESIAN_POINT('Ctrl Pts',(-0.035238397980778,0.704453790598787,
-5.12702704523444));
#54116=CARTESIAN_POINT('Ctrl Pts',(-0.367561754396992,0.601992727934364,
-5.11116953465848));
#54117=CARTESIAN_POINT('Ctrl Pts',(-0.610534107144088,0.353192570413113,
-5.09531202408255));
#54118=CARTESIAN_POINT('Ctrl Pts',(-0.705091031476859,0.0185344304511741,
-5.0794545135066));
#54119=CARTESIAN_POINT('Ctrl Pts',(-0.628246577437432,-0.320629265226061,
-5.06359700293066));
#54120=CARTESIAN_POINT('Ctrl Pts',(-0.398680950495202,-0.581850829245344,
-5.04773949235472));
#54121=CARTESIAN_POINT('Ctrl Pts',(-0.0721995192170595,-0.701629615399804,
-5.03188198177877));
#54122=CARTESIAN_POINT('Ctrl Pts',(0.271832975057436,-0.650848462741271,
-5.01602447120283));
#54123=CARTESIAN_POINT('Ctrl Pts',(0.549785283183103,-0.441851819252255,
-5.00016696062688));
#54124=CARTESIAN_POINT('Ctrl Pts',(0.694089663396602,-0.125444915988027,
-4.98430945005094));
#54125=CARTESIAN_POINT('Ctrl Pts',(0.669667000279414,0.221456534150661,
-4.968451939475));
#54126=CARTESIAN_POINT('Ctrl Pts',(0.482454226702515,0.514523864284379,
-4.95259442889905));
#54127=CARTESIAN_POINT('Ctrl Pts',(0.177961108082654,0.682515004810329,
-4.93673691832311));
#54128=CARTESIAN_POINT('Ctrl Pts',(-0.169792778098127,0.684592798886295,
-4.92087940774717));
#54129=CARTESIAN_POINT('Ctrl Pts',(-0.476271545316318,0.520252153194254,
-4.90502189717122));
#54130=CARTESIAN_POINT('Ctrl Pts',(-0.666972922520502,0.229442821647816,
-4.88916438659529));
#54131=CARTESIAN_POINT('Ctrl Pts',(-0.695539095682312,-0.117142025587244,
-4.87330687601934));
#54132=CARTESIAN_POINT('Ctrl Pts',(-0.555025881375534,-0.435250684990344,
-4.85744936544339));
#54133=CARTESIAN_POINT('Ctrl Pts',(-0.279590796199469,-0.647553761831247,
-4.84159185486746));
#54134=CARTESIAN_POINT('Ctrl Pts',(0.0638103326637412,-0.702442260421875,
-4.8257343442915));
#54135=CARTESIAN_POINT('Ctrl Pts',(0.391699735402671,-0.586573273399606,
-4.80987683371557));
#54136=CARTESIAN_POINT('Ctrl Pts',(0.624370405298808,-0.32811352420809,
-4.79401932313962));
#54137=CARTESIAN_POINT('Ctrl Pts',(0.705262165372666,0.0101077136440157,
-4.77816181256367));
#54138=CARTESIAN_POINT('Ctrl Pts',(0.614710945941539,0.345871855924866,
-4.76230430198774));
#54139=CARTESIAN_POINT('Ctrl Pts',(0.374728945616527,0.597557616551221,
-4.74644679141179));
#54140=CARTESIAN_POINT('Ctrl Pts',(0.0436536609816854,0.703982418576024,
-4.73058928083585));
#54141=CARTESIAN_POINT('Ctrl Pts',(-0.298033441601801,0.639275336195787,
-4.71473177025991));
#54142=CARTESIAN_POINT('Ctrl Pts',(-0.567271256914447,0.419166087440235,
-4.69887425968396));
#54143=CARTESIAN_POINT('Ctrl Pts',(-0.69861045913254,0.0971612791798993,
-4.68301674910802));
#54144=CARTESIAN_POINT('Ctrl Pts',(-0.660123652658186,-0.248462574611278,
-4.66715923853208));
#54145=CARTESIAN_POINT('Ctrl Pts',(-0.461166638918949,-0.533687379398699,
-4.65130172795613));
#54146=CARTESIAN_POINT('Ctrl Pts',(-0.15010410398989,-0.689177513958953,
-4.63544421738019));
#54147=CARTESIAN_POINT('Ctrl Pts',(0.197447407787028,-0.677134705165401,
-4.61958670680424));
#54148=CARTESIAN_POINT('Ctrl Pts',(0.497001205311606,-0.500486453063479,
-4.6037291962283));
#54149=CARTESIAN_POINT('Ctrl Pts',(0.675738416267745,-0.202174381565054,
-4.58787168565236));
#54150=CARTESIAN_POINT('Ctrl Pts',(0.690209609366951,0.145284489601514,
-4.57201417507641));
#54151=CARTESIAN_POINT('Ctrl Pts',(0.536896965869284,0.457425989447045,
-4.55615666450047));
#54152=CARTESIAN_POINT('Ctrl Pts',(0.253069430129838,0.658371286824547,
-4.54029915392453));
#54153=CARTESIAN_POINT('Ctrl Pts',(-0.0922770403452622,0.699272361534738,
-4.52444164334858));
#54154=CARTESIAN_POINT('Ctrl Pts',(-0.415191780446262,0.570186524946981,
-4.50858413277264));
#54155=CARTESIAN_POINT('Ctrl Pts',(-0.637177079836271,0.302493399452904,
-4.49272662219669));
#54156=CARTESIAN_POINT('Ctrl Pts',(-0.704270280368694,-0.0387331895233606,
-4.47686911162076));
#54157=CARTESIAN_POINT('Ctrl Pts',(-0.600161619846482,-0.370544083537301,
-4.46101160104481));
#54158=CARTESIAN_POINT('Ctrl Pts',(-0.350158990608888,-0.61227899610963,
-4.44515409046887));
#54159=CARTESIAN_POINT('Ctrl Pts',(-0.0150358152851096,-0.705174313230397,
-4.42929657989292));
#54160=CARTESIAN_POINT('Ctrl Pts',(0.32374243342603,-0.626648006923061,
-4.41343906931699));
#54161=CARTESIAN_POINT('Ctrl Pts',(0.583821766891339,-0.39578912603194,
-4.39758155874103));
#54162=CARTESIAN_POINT('Ctrl Pts',(0.701979205024536,-0.0687174176928368,
-4.3817240481651));
#54163=CARTESIAN_POINT('Ctrl Pts',(0.649491722206451,0.275058885634601,
-4.36586653758914));
#54164=CARTESIAN_POINT('Ctrl Pts',(0.439118560152959,0.551970812553023,
-4.35000902701321));
#54165=CARTESIAN_POINT('Ctrl Pts',(0.121999569378052,0.694703528746487,
-4.33415151643726));
#54166=CARTESIAN_POINT('Ctrl Pts',(-0.224776435057083,0.668559976385276,
-4.31829400586132));
#54167=CARTESIAN_POINT('Ctrl Pts',(-0.516911281011339,0.479895421258078,
-4.30243649528538));
#54168=CARTESIAN_POINT('Ctrl Pts',(-0.683389577518488,0.174572544004934,
-4.28657898470943));
#54169=CARTESIAN_POINT('Ctrl Pts',(-0.683741926704308,-0.173187370925052,
-4.27072147413349));
#54170=CARTESIAN_POINT('Ctrl Pts',(-0.517882675605679,-0.478846971472886,
-4.25486396355754));
#54171=CARTESIAN_POINT('Ctrl Pts',(-0.226130737646503,-0.668103118741933,
-4.23900645298161));
#54172=CARTESIAN_POINT('Ctrl Pts',(0.120591577745708,-0.694949321287569,
-4.22314894240565));
#54173=CARTESIAN_POINT('Ctrl Pts',(0.437999149760179,-0.552859505291001,
-4.20729143182972));
#54174=CARTESIAN_POINT('Ctrl Pts',(0.648933011794961,-0.276374445244078,
-4.19143392125377));
#54175=CARTESIAN_POINT('Ctrl Pts',(0.702117012141806,0.0672947920890993,
-4.17557641067783));
#54176=CARTESIAN_POINT('Ctrl Pts',(0.584622591848963,0.394605262105121,
-4.15971890010188));
#54177=CARTESIAN_POINT('Ctrl Pts',(0.325011602776974,0.625990691497561,
-4.14386138952594));
#54178=CARTESIAN_POINT('Ctrl Pts',(-0.0136068253575281,0.705203333858357,
-4.12800387895));
#54179=CARTESIAN_POINT('Ctrl Pts',(-0.348917554886554,0.612987298133689,
-4.11214636837405));
#54180=CARTESIAN_POINT('Ctrl Pts',(-0.599409520346848,0.371759485015262,
-4.09628885779812));
#54181=CARTESIAN_POINT('Ctrl Pts',(-0.704190345811963,0.0401602371317554,
-4.08043134722216));
#54182=CARTESIAN_POINT('Ctrl Pts',(-0.637788741604482,-0.301201608335383,
-4.06457383664623));
#54183=CARTESIAN_POINT('Ctrl Pts',(-0.416346348986597,-0.569344013287909,
-4.04871632607028));
#54184=CARTESIAN_POINT('Ctrl Pts',(-0.0936938502820333,-0.699083936448678,
-4.03285881549434));
#54185=CARTESIAN_POINT('Ctrl Pts',(0.251734792730736,-0.658882752779327,
-4.01700130491839));
#54186=CARTESIAN_POINT('Ctrl Pts',(0.535968939526595,-0.458513013603747,
-4.00114379434245));
#54187=CARTESIAN_POINT('Ctrl Pts',(0.689913789056643,-0.146682826025263,
-3.98528628376651));
#54188=CARTESIAN_POINT('Ctrl Pts',(0.676146713284492,0.200804656061129,
-3.96942877319056));
#54189=CARTESIAN_POINT('Ctrl Pts',(0.49801436627063,0.499478306605316,-3.95357126261462));
#54190=CARTESIAN_POINT('Ctrl Pts',(0.198819142241936,0.676733209218694,
-3.93771375203867));
#54191=CARTESIAN_POINT('Ctrl Pts',(-0.148707252523208,0.689480268628661,
-3.92185624146274));
#54192=CARTESIAN_POINT('Ctrl Pts',(-0.460084232647476,0.534620787708854,
-3.90599873088679));
#54193=CARTESIAN_POINT('Ctrl Pts',(-0.659618814949835,0.249799733277333,
-3.89014122031085));
#54194=CARTESIAN_POINT('Ctrl Pts',(-0.698805911558285,-0.0957454215743307,
-3.8742837097349));
#54195=CARTESIAN_POINT('Ctrl Pts',(-0.568119486722484,-0.418015713325986,
-3.85842619915896));
#54196=CARTESIAN_POINT('Ctrl Pts',(-0.299328251646252,-0.638670091320746,
-3.84256868858302));
#54197=CARTESIAN_POINT('Ctrl Pts',(0.0422270275427583,-0.704069432603173,
-3.82671117800707));
#54198=CARTESIAN_POINT('Ctrl Pts',(0.373517290723508,-0.598315737142038,
-3.81085366743113));
#54199=CARTESIAN_POINT('Ctrl Pts',(0.614008812156318,-0.347116790685268,
-3.79499615685518));
#54200=CARTESIAN_POINT('Ctrl Pts',(0.705240235193272,-0.0115368299714127,
-3.77913864627925));
#54201=CARTESIAN_POINT('Ctrl Pts',(0.625034009757416,0.326847631822259,
-3.76328113570329));
#54202=CARTESIAN_POINT('Ctrl Pts',(0.392887558138946,0.585778332170854,
-3.74742362512736));
#54203=CARTESIAN_POINT('Ctrl Pts',(0.065233624501804,0.702311513514914,
-3.73156611455141));
#54204=CARTESIAN_POINT('Ctrl Pts',(-0.278278024886458,0.648118992659946,
-3.71570860397547));
#54205=CARTESIAN_POINT('Ctrl Pts',(-0.554142753654658,0.436374490951619,
-3.69985109339953));
#54206=CARTESIAN_POINT('Ctrl Pts',(-0.695300292072653,0.11855121941564,
-3.68399358282358));
#54207=CARTESIAN_POINT('Ctrl Pts',(-0.667436494062319,-0.228090802477984,
-3.66813607224764));
#54208=CARTESIAN_POINT('Ctrl Pts',(-0.47732480187785,-0.519285972556088,
-3.65227856167169));
#54209=CARTESIAN_POINT('Ctrl Pts',(-0.171179682347504,-0.684247326726716,
-3.63642105109576));
#54210=CARTESIAN_POINT('Ctrl Pts',(0.176577700272081,-0.682874222348358,
-3.6205635405198));
#54211=CARTESIAN_POINT('Ctrl Pts',(0.48141060950412,-0.51550044892136,-3.60470602994387));
#54212=CARTESIAN_POINT('Ctrl Pts',(0.66921686778135,-0.222813086819806,
-3.58884851936792));
#54213=CARTESIAN_POINT('Ctrl Pts',(0.694342438818249,0.12403816121331,-3.57299100879198));
#54214=CARTESIAN_POINT('Ctrl Pts',(0.550679519060578,0.440736831985327,
-3.55713349821603));
#54215=CARTESIAN_POINT('Ctrl Pts',(0.273151290577277,0.650296286501176,
-3.54127598764009));
#54216=CARTESIAN_POINT('Ctrl Pts',(-0.0707775948694625,0.701774479334883,
-3.52541847706415));
#54217=CARTESIAN_POINT('Ctrl Pts',(-0.397501074521878,0.582657518217351,
-3.5095609664882));
#54218=CARTESIAN_POINT('Ctrl Pts',(-0.627595567226647,0.321901680298058,
-3.49370345591226));
#54219=CARTESIAN_POINT('Ctrl Pts',(-0.705127141838962,-0.0171056021018824,
-3.47784594533632));
#54220=CARTESIAN_POINT('Ctrl Pts',(-0.611248559970205,-0.351954664290164,
-3.46198843476037));
#54221=CARTESIAN_POINT('Ctrl Pts',(-0.368780872539474,-0.601246668040893,
-3.44613092418443));
#54222=CARTESIAN_POINT('Ctrl Pts',(-0.0366658246279656,-0.704380937480284,
-3.43027341360848));
#54223=CARTESIAN_POINT('Ctrl Pts',(0.304362360169178,-0.636286446102303,
-3.41441590303255));
#54224=CARTESIAN_POINT('Ctrl Pts',(0.571402753704327,-0.413516361031052,
-3.3985583924566));
#54225=CARTESIAN_POINT('Ctrl Pts',(0.699540203905405,-0.0902241148542729,
-3.38270088188066));
#54226=CARTESIAN_POINT('Ctrl Pts',(0.657625632702926,0.255000813711106,
-3.36684337130472));
#54227=CARTESIAN_POINT('Ctrl Pts',(0.455848100739092,0.538237305315985,
-3.35098586072876));
#54228=CARTESIAN_POINT('Ctrl Pts',(0.143257937062477,0.690633080043126,
-3.33512835015283));
#54229=CARTESIAN_POINT('Ctrl Pts',(-0.204156960980475,0.675142076206533,
-3.31927083957688));
#54230=CARTESIAN_POINT('Ctrl Pts',(-0.501943111877064,0.495530019494702,
-3.30341332900094));
#54231=CARTESIAN_POINT('Ctrl Pts',(-0.677711342534395,0.195459008442898,
-3.28755581842499));
#54232=CARTESIAN_POINT('Ctrl Pts',(-0.688733954451453,-0.152126354609959,
-3.27169830784905));
#54233=CARTESIAN_POINT('Ctrl Pts',(-0.532331448398351,-0.462731149618616,
-3.25584079727311));
#54234=CARTESIAN_POINT('Ctrl Pts',(-0.246523886922497,-0.660850104757407,
-3.23998328669717));
#54235=CARTESIAN_POINT('Ctrl Pts',(0.0992114457684886,-0.698322258566757,
-3.22412577612122));
#54236=CARTESIAN_POINT('Ctrl Pts',(0.420829355607847,-0.566038462686005,
-3.20826826554528));
#54237=CARTESIAN_POINT('Ctrl Pts',(0.640147380197513,-0.296155735057606,
-3.19241075496933));
#54238=CARTESIAN_POINT('Ctrl Pts',(0.703851252246643,0.0457198260286,-3.17655324439339));
#54239=CARTESIAN_POINT('Ctrl Pts',(0.596455125262476,0.376481302762003,
-3.16069573381745));
#54240=CARTESIAN_POINT('Ctrl Pts',(0.344066045534297,0.615723512700013,
-3.14483822324151));
#54241=CARTESIAN_POINT('Ctrl Pts',(0.00803756064714361,0.705288795742634,
-3.12898071266556));
#54242=CARTESIAN_POINT('Ctrl Pts',(-0.32994478397183,0.623404625673433,
-3.11312320208962));
#54243=CARTESIAN_POINT('Ctrl Pts',(-0.587720476917705,0.38997631824622,
-3.09726569151367));
#54244=CARTESIAN_POINT('Ctrl Pts',(-0.702626532690257,0.0617482254070272,
-3.08140818093773));
#54245=CARTESIAN_POINT('Ctrl Pts',(-0.646730307895239,-0.281490313565102,
-3.06555067036178));
#54246=CARTESIAN_POINT('Ctrl Pts',(-0.433619679201001,-0.556301053019741,
-3.04969315978585));
#54247=CARTESIAN_POINT('Ctrl Pts',(-0.115099950991358,-0.695879938684137,
-3.0338356492099));
#54248=CARTESIAN_POINT('Ctrl Pts',(0.231399554821144,-0.666296580968136,
-3.01797813863396));
#54249=CARTESIAN_POINT('Ctrl Pts',(0.521647880459103,-0.474742431844655,
-3.00212062805801));
#54250=CARTESIAN_POINT('Ctrl Pts',(0.685088231319183,-0.167782606634913,
-2.98626311748207));
#54251=CARTESIAN_POINT('Ctrl Pts',(0.681989707179352,0.179963682677014,
-2.97040560690613));
#54252=CARTESIAN_POINT('Ctrl Pts',(0.513105531786303,0.48396239629908,-2.95454809633019));
#54253=CARTESIAN_POINT('Ctrl Pts',(0.219489950840751,0.670314142220776,
-2.93869058575424));
#54254=CARTESIAN_POINT('Ctrl Pts',(-0.127481691142976,0.693718463214421,
-2.92283307517829));
#54255=CARTESIAN_POINT('Ctrl Pts',(-0.443463664270248,0.548485976350586,
-2.90697556460236));
#54256=CARTESIAN_POINT('Ctrl Pts',(-0.651643552389154,0.269921411545835,
-2.89111805402641));
#54257=CARTESIAN_POINT('Ctrl Pts',(-0.701414670433489,-0.0742586552661132,
-2.87526054345047));
#54258=CARTESIAN_POINT('Ctrl Pts',(-0.580678100880426,-0.400387101364609,
-2.85940303287452));
#54259=CARTESIAN_POINT('Ctrl Pts',(-0.318783833330571,-0.629184992977676,
-2.84354552229858));
#54260=CARTESIAN_POINT('Ctrl Pts',(0.0206039577451542,-0.705033591190155,
-2.82768801172263));
#54261=CARTESIAN_POINT('Ctrl Pts',(0.35498310936897,-0.609494774254864,
-2.81183050114669));
#54262=CARTESIAN_POINT('Ctrl Pts',(0.603069014406956,-0.365793181515832,
-2.79597299057075));
#54263=CARTESIAN_POINT('Ctrl Pts',(0.704554188889049,-0.0331705094948168,
-2.78011547999481));
#54264=CARTESIAN_POINT('Ctrl Pts',(0.634768486672358,0.307515619292639,
-2.76425796941886));
#54265=CARTESIAN_POINT('Ctrl Pts',(0.410676193241495,0.573447427482177,
-2.74840045884292));
#54266=CARTESIAN_POINT('Ctrl Pts',(0.0867521583136464,0.699979250270445,
-2.73254294826698));
#54267=CARTESIAN_POINT('Ctrl Pts',(-0.258260557150356,0.656352323376431,
-2.71668543769103));
#54268=CARTESIAN_POINT('Ctrl Pts',(-0.54049242092486,0.453171965929088,
-2.70082792711509));
#54269=CARTESIAN_POINT('Ctrl Pts',(-0.691335369211096,0.139829521414503,
-2.68497041653915));
#54270=CARTESIAN_POINT('Ctrl Pts',(-0.674120818663402,-0.207504240018937,
-2.6691129059632));
#54271=CARTESIAN_POINT('Ctrl Pts',(-0.493033473894675,-0.504395560448939,
-2.65325539538726));
#54272=CARTESIAN_POINT('Ctrl Pts',(-0.19209406288682,-0.678672792135419,
-2.63739788481132));
#54273=CARTESIAN_POINT('Ctrl Pts',(0.155541711691216,-0.687970685207893,
-2.62154037423537));
#54274=CARTESIAN_POINT('Ctrl Pts',(0.465366675199364,-0.530029004296125,
-2.60568286365943));
#54275=CARTESIAN_POINT('Ctrl Pts',(0.662065125935696,-0.243241971709246,
-2.58982535308348));
#54276=CARTESIAN_POINT('Ctrl Pts',(0.697821414466598,0.102675027602084,
-2.57396784250754));
#54277=CARTESIAN_POINT('Ctrl Pts',(0.563943504067627,0.423632638026367,
-2.5581103319316));
#54278=CARTESIAN_POINT('Ctrl Pts',(0.292975927787107,0.641608910099083,
-2.54225282135566));
#54279=CARTESIAN_POINT('Ctrl Pts',(-0.0492114989961208,0.703615744670204,
-2.52639531077971));
#54280=CARTESIAN_POINT('Ctrl Pts',(-0.379436046685527,0.594579830011842,
-2.51053780020377));
#54281=CARTESIAN_POINT('Ctrl Pts',(-0.617423055528672,0.341006830258411,
-2.49468028962782));
#54282=CARTESIAN_POINT('Ctrl Pts',(-0.705319993683033,0.00453809345638933,
-2.47882277905188));
#54283=CARTESIAN_POINT('Ctrl Pts',(-0.621759894782861,-0.333033813629871,
-2.46296526847594));
#54284=CARTESIAN_POINT('Ctrl Pts',(-0.387055478021894,-0.589648153320687,
-2.4471077579));
#54285=CARTESIAN_POINT('Ctrl Pts',(-0.0582613062111292,-0.70292425479551,
-2.43125024732405));
#54286=CARTESIAN_POINT('Ctrl Pts',(0.284695672591286,-0.645325702098597,
-2.41539273674811));
#54287=CARTESIAN_POINT('Ctrl Pts',(0.558445657515852,-0.430854192718303,
-2.39953522617216));
#54288=CARTESIAN_POINT('Ctrl Pts',(0.696442454311359,-0.111645849067578,
-2.38367771559622));
#54289=CARTESIAN_POINT('Ctrl Pts',(0.665140265164793,0.234702610632607,
-2.36782020502028));
#54290=CARTESIAN_POINT('Ctrl Pts',(0.472148374730573,0.523996946575577,
-2.35196269444434));
#54291=CARTESIAN_POINT('Ctrl Pts',(0.164381400495464,0.685912270594717,
-2.33610518386839));
#54292=CARTESIAN_POINT('Ctrl Pts',(-0.183345234784635,0.681088402972051,
-2.32024767329245));
#54293=CARTESIAN_POINT('Ctrl Pts',(-0.486502269038555,0.510697983157941,
-2.3043901627165));
#54294=CARTESIAN_POINT('Ctrl Pts',(-0.671394915047807,0.216161411517411,
-2.28853265214056));
#54295=CARTESIAN_POINT('Ctrl Pts',(-0.69307740983695,-0.130922082762827,
-2.27267514156461));
#54296=CARTESIAN_POINT('Ctrl Pts',(-0.546278931161056,-0.446179579486538,
-2.25681763098868));
#54297=CARTESIAN_POINT('Ctrl Pts',(-0.266684887662029,-0.652974776292271,
-2.24096012041273));
#54298=CARTESIAN_POINT('Ctrl Pts',(0.0777378875832581,-0.701037594295302,
-2.22510260983679));
#54299=CARTESIAN_POINT('Ctrl Pts',(0.403263271585882,-0.578684388566949,
-2.20924509926084));
#54300=CARTESIAN_POINT('Ctrl Pts',(0.630758929622586,-0.315658138628835,
-2.1933875886849));
#54301=CARTESIAN_POINT('Ctrl Pts',(0.704922684214943,0.0241018061657587,
-2.17753007810895));
#54302=CARTESIAN_POINT('Ctrl Pts',(0.607725984161892,0.358002815569531,
-2.16167256753301));
#54303=CARTESIAN_POINT('Ctrl Pts',(0.362796485494498,0.604876514583012,
-2.14581505695707));
#54304=CARTESIAN_POINT('Ctrl Pts',(0.0296743777790237,0.704710095773204,
-2.12995754638113));
#54305=CARTESIAN_POINT('Ctrl Pts',(-0.310661308079694,0.633234900683358,
-2.11410003580518));
#54306=CARTESIAN_POINT('Ctrl Pts',(-0.575477984286229,0.407825915536408,
-2.09824252522924));
#54307=CARTESIAN_POINT('Ctrl Pts',(-0.700401064735479,0.0832780661318421,
-2.08238501465329));
#54308=CARTESIAN_POINT('Ctrl Pts',(-0.655062856145828,-0.261513942800995,
-2.06652750407735));
#54309=CARTESIAN_POINT('Ctrl Pts',(-0.450484675054114,-0.542734230837378,
-2.05066999350141));
#54310=CARTESIAN_POINT('Ctrl Pts',(-0.13639766348118,-0.692020639271782,
-2.03481248292547));
#54311=CARTESIAN_POINT('Ctrl Pts',(0.210846410774077,-0.67308296579615,
-2.01895497234952));
#54312=CARTESIAN_POINT('Ctrl Pts',(0.506835591947215,-0.490524790929845,
-2.00309746177358));
#54313=CARTESIAN_POINT('Ctrl Pts',(0.679617534353063,-0.188724388411024,
-1.98723995119763));
#54314=CARTESIAN_POINT('Ctrl Pts',(0.687190479687935,0.158953239688651,
-1.97138244062169));
#54315=CARTESIAN_POINT('Ctrl Pts',(0.527713512083115,0.467990744509071,
-1.95552493004575));
#54316=CARTESIAN_POINT('Ctrl Pts',(0.239954068430876,0.663263848573645,
-1.93966741946981));
#54317=CARTESIAN_POINT('Ctrl Pts',(-0.106136081809596,0.697303391587448,
-1.92380990889386));
#54318=CARTESIAN_POINT('Ctrl Pts',(-0.426425491571088,0.561834662440479,
-1.90795239831792));
#54319=CARTESIAN_POINT('Ctrl Pts',(-0.643054645045905,0.289788908114401,
-1.89209488774197));
#54320=CARTESIAN_POINT('Ctrl Pts',(-0.703362915671523,-0.0527019604882636,
-1.87623737716603));
#54321=CARTESIAN_POINT('Ctrl Pts',(-0.592689897555636,-0.382381449755007,
-1.86037986659008));
#54322=CARTESIAN_POINT('Ctrl Pts',(-0.337939220168536,-0.619107398803415,
-1.84452235601415));
#54323=CARTESIAN_POINT('Ctrl Pts',(-0.00103851454807973,-0.705333828246443,
-1.8286648454382));
#54324=CARTESIAN_POINT('Ctrl Pts',(0.336114644751484,-0.620099857575242,
-1.81280733486226));
#54325=CARTESIAN_POINT('Ctrl Pts',(0.591561313924781,-0.384125109370422,
-1.79694982428632));
#54326=CARTESIAN_POINT('Ctrl Pts',(0.70320467250143,-0.0547729527541542,
-1.78109231371037));
#54327=CARTESIAN_POINT('Ctrl Pts',(0.64390520984823,0.287894023056329,-1.76523480313443));
#54328=CARTESIAN_POINT('Ctrl Pts',(0.428078099583546,0.560576514347677,
-1.74937729255848));
#54329=CARTESIAN_POINT('Ctrl Pts',(0.10818899867648,0.69698782510646,-1.73351978198254));
#54330=CARTESIAN_POINT('Ctrl Pts',(-0.237999888598618,0.663967575118165,
-1.7176622714066));
#54331=CARTESIAN_POINT('Ctrl Pts',(-0.526333113076832,0.469542694395412,
-1.70180476083065));
#54332=CARTESIAN_POINT('Ctrl Pts',(-0.686719424267349,0.160976147659122,
-1.68594725025471));
#54333=CARTESIAN_POINT('Ctrl Pts',(-0.680170331914515,-0.186722273348817,
-1.67008973967877));
#54334=CARTESIAN_POINT('Ctrl Pts',(-0.508277862304651,-0.489030165196652,
-1.65423222910282));
#54335=CARTESIAN_POINT('Ctrl Pts',(-0.212827550790863,-0.672459159656269,
-1.63837471852688));
#54336=CARTESIAN_POINT('Ctrl Pts',(0.134359251378219,-0.692419294467113,
-1.62251720795094));
#54337=CARTESIAN_POINT('Ctrl Pts',(0.448884510774523,-0.54405843782444,
-1.60665969737499));
#54338=CARTESIAN_POINT('Ctrl Pts',(0.65428992543882,-0.263441798601729,
-1.59080218679905));
#54339=CARTESIAN_POINT('Ctrl Pts',(0.700643260203079,0.0812152061701052,
-1.57494467622311));
#54340=CARTESIAN_POINT('Ctrl Pts',(0.576676430357581,0.406129514380929,
-1.55908716564716));
#54341=CARTESIAN_POINT('Ctrl Pts',(0.312524673140342,0.63231733841464,-1.54322965507122));
#54342=CARTESIAN_POINT('Ctrl Pts',(-0.0275990612546199,0.704794423643601,
-1.52737214449527));
#54343=CARTESIAN_POINT('Ctrl Pts',(-0.361013708553533,0.605942233234882,
-1.51151463391933));
#54344=CARTESIAN_POINT('Ctrl Pts',(-0.606669124072505,0.359790858247332,
-1.49565712334339));
#54345=CARTESIAN_POINT('Ctrl Pts',(-0.704848654294675,0.0261775155474184,
-1.47979961276745));
#54346=CARTESIAN_POINT('Ctrl Pts',(-0.631685725888709,-0.313799349090631,
-1.4639421021915));
#54347=CARTESIAN_POINT('Ctrl Pts',(-0.404965598083139,-0.577494374128802,
-1.44808459161556));
#54348=CARTESIAN_POINT('Ctrl Pts',(-0.0798019238330923,-0.700805636916392,
-1.43222708103962));
#54349=CARTESIAN_POINT('Ctrl Pts',(0.264760890572085,-0.65375726275486,
-1.41636957046367));
#54350=CARTESIAN_POINT('Ctrl Pts',(0.544962679865294,-0.447786294269141,
-1.40051205988773));
#54351=CARTESIAN_POINT('Ctrl Pts',(0.692688873355398,-0.13296244774702,
-1.38465454931178));
#54352=CARTESIAN_POINT('Ctrl Pts',(0.672028543154347,0.21418339096928,-1.36879703873584));
#54353=CARTESIAN_POINT('Ctrl Pts',(0.488004032358267,0.509263146303875,
-1.3529395281599));
#54354=CARTESIAN_POINT('Ctrl Pts',(0.185350067969226,0.680545545929922,
-1.33708201758396));
#54355=CARTESIAN_POINT('Ctrl Pts',(-0.162360854618199,0.686393357098464,
-1.32122450700801));
#54356=CARTESIAN_POINT('Ctrl Pts',(-0.470603292949117,0.525385028761478,
-1.30536699643207));
#54357=CARTESIAN_POINT('Ctrl Pts',(-0.664446243161424,0.236660258028087,
-1.28950948585612));
#54358=CARTESIAN_POINT('Ctrl Pts',(-0.696768202681856,-0.109594523187739,
-1.27365197528018));
#54359=CARTESIAN_POINT('Ctrl Pts',(-0.559711989719446,-0.429207847488311,
-1.25779446470423));
#54360=CARTESIAN_POINT('Ctrl Pts',(-0.286594754496667,-0.644484549447267,
-1.2419369541283));
#54361=CARTESIAN_POINT('Ctrl Pts',(0.0561911245777891,-0.703092771474672,
-1.22607944355235));
#54362=CARTESIAN_POINT('Ctrl Pts',(0.385317439461293,-0.590785374419714,
-1.21022193297641));
#54363=CARTESIAN_POINT('Ctrl Pts',(0.620776501059534,-0.33486329078227,
-1.19436442240046));
#54364=CARTESIAN_POINT('Ctrl Pts',(0.705330299092296,0.00246108992610756,
-1.17850691182452));
#54365=CARTESIAN_POINT('Ctrl Pts',(0.618424554916906,0.339187201493628,
-1.16264940124858));
#54366=CARTESIAN_POINT('Ctrl Pts',(0.381185284430804,0.593459911632335,
-1.14679189067263));
#54367=CARTESIAN_POINT('Ctrl Pts',(0.0512832509114107,0.703467778904769,
-1.13093438009669));
#54368=CARTESIAN_POINT('Ctrl Pts',(-0.291085286224135,0.642468866113421,
-1.11507686952075));
#54369=CARTESIAN_POINT('Ctrl Pts',(-0.562693571058386,0.425291468137809,
-1.0992193589448));
#54370=CARTESIAN_POINT('Ctrl Pts',(-0.697516037643649,0.104729484917831,
-1.08336184836886));
#54371=CARTESIAN_POINT('Ctrl Pts',(-0.662778539697212,-0.241291307547711,
-1.06750433779292));
#54372=CARTESIAN_POINT('Ctrl Pts',(-0.466925454985086,-0.528656322451762,
-1.05164682721697));
#54373=CARTESIAN_POINT('Ctrl Pts',(-0.157566931955473,-0.687509672466789,
-1.03578931664103));
#54374=CARTESIAN_POINT('Ctrl Pts',(0.190094715234546,-0.679235516607566,
-1.01993180606508));
#54375=CARTESIAN_POINT('Ctrl Pts',(0.491546022542315,-0.505845228804307,
-1.00407429548914));
#54376=CARTESIAN_POINT('Ctrl Pts',(0.673506849846877,-0.209488450733178,
-0.988216784913199));
#54377=CARTESIAN_POINT('Ctrl Pts',(0.691744133306218,0.137793112373883,
-0.972359274337254));
#54378=CARTESIAN_POINT('Ctrl Pts',(0.541824551004231,0.45157839154494,-0.956501763761313));
#54379=CARTESIAN_POINT('Ctrl Pts',(0.260192224202427,0.655588967452813,
-0.940644253185368));
#54380=CARTESIAN_POINT('Ctrl Pts',(-0.0846905254229573,0.700231677864431,
-0.924786742609425));
#54381=CARTESIAN_POINT('Ctrl Pts',(-0.408985759189344,0.574654275683705,
-0.908929232033481));
#54382=CARTESIAN_POINT('Ctrl Pts',(-0.633860180989338,0.30938351400392,
-0.89307172145754));
#54383=CARTESIAN_POINT('Ctrl Pts',(-0.704648812633615,-0.0310956369172294,
-0.877214210881594));
#54384=CARTESIAN_POINT('Ctrl Pts',(-0.604143565385745,-0.364015714199608,
-0.861356700305653));
#54385=CARTESIAN_POINT('Ctrl Pts',(-0.356776373766072,-0.608446798745448,
-0.845499189729708));
#54386=CARTESIAN_POINT('Ctrl Pts',(-0.0226800088848199,-0.704969861042468,
-0.829641679153765));
#54387=CARTESIAN_POINT('Ctrl Pts',(0.316929665073997,-0.630121000425581,
-0.813784168577821));
#54388=CARTESIAN_POINT('Ctrl Pts',(0.579496547370947,-0.40209531129622,
-0.797926658001879));
#54389=CARTESIAN_POINT('Ctrl Pts',(0.701192956853533,-0.0763238169921492,
-0.782069147425935));
#54390=CARTESIAN_POINT('Ctrl Pts',(0.652435575344282,0.268001320531126,
-0.76621163684999));
#54391=CARTESIAN_POINT('Ctrl Pts',(0.445076890002194,0.547177713149235,
-0.750354126274048));
#54392=CARTESIAN_POINT('Ctrl Pts',(0.129523958779256,0.693340055011537,
-0.734496615698105));
#54393=CARTESIAN_POINT('Ctrl Pts',(-0.217515098455649,0.670957576695487,
-0.718639105122159));
#54394=CARTESIAN_POINT('Ctrl Pts',(-0.511678163758033,0.485471260235309,
-0.702781594546218));
#54395=CARTESIAN_POINT('Ctrl Pts',(-0.681456804020454,0.181971184629545,
-0.686924083970274));
#54396=CARTESIAN_POINT('Ctrl Pts',(-0.685579337062831,-0.165764472592108,
-0.671066573394329));
#54397=CARTESIAN_POINT('Ctrl Pts',(-0.523043611653193,-0.47320425620448,
-0.655209062818387));
#54398=CARTESIAN_POINT('Ctrl Pts',(-0.233360621587032,-0.66561228059116,
-0.639351552242444));
#54399=CARTESIAN_POINT('Ctrl Pts',(0.113050266597516,-0.696215860924957,
-0.6234940416665));
#54400=CARTESIAN_POINT('Ctrl Pts',(0.431979637282727,-0.55757553815993,
-0.607636531090557));
#54401=CARTESIAN_POINT('Ctrl Pts',(0.645898588102162,-0.283393545566738,
-0.591779020514614));
#54402=CARTESIAN_POINT('Ctrl Pts',(0.702805318729989,0.0596789053693757,
-0.57592150993867));
#54403=CARTESIAN_POINT('Ctrl Pts',(0.588866307489121,0.388243943526985,
-0.560063999362727));
#54404=CARTESIAN_POINT('Ctrl Pts',(0.331779117822002,0.622430321207524,
-0.544206488786783));
#54405=CARTESIAN_POINT('Ctrl Pts',(-0.00596063381383579,0.705309406307461,
-0.52834897821084));
#54406=CARTESIAN_POINT('Ctrl Pts',(-0.34225140821695,0.616734028050019,
-0.512491467634896));
#54407=CARTESIAN_POINT('Ctrl Pts',(-0.595343899704099,0.378236075574855,
-0.496633957058954));
#54408=CARTESIAN_POINT('Ctrl Pts',(-0.703713567528586,0.0477922865914934,
-0.480776446483009));
#54409=CARTESIAN_POINT('Ctrl Pts',(-0.641016706253422,-0.294269383533106,
-0.464918935907065));
#54410=CARTESIAN_POINT('Ctrl Pts',(-0.422494366982188,-0.564796775530692,
-0.449061425331123));
#54411=CARTESIAN_POINT('Ctrl Pts',(-0.101267392955972,-0.698027078919814,
-0.433203914755179));
#54412=CARTESIAN_POINT('Ctrl Pts',(0.244576786450544,-0.661573188172743,
-0.417346404179235));
#54413=CARTESIAN_POINT('Ctrl Pts',(0.530966517512247,-0.464296720931165,
-0.401488893603292));
#54414=CARTESIAN_POINT('Ctrl Pts',(0.68828299573105,-0.1541538373096,-0.385631383027349));
#54415=CARTESIAN_POINT('Ctrl Pts',(0.678283980079609,0.193462477415893,
-0.369773872451405));
#54416=CARTESIAN_POINT('Ctrl Pts',(0.503400142512799,0.494049779148767,
-0.353916361875461));
#54417=CARTESIAN_POINT('Ctrl Pts',(0.206144193604109,0.674537959812384,
-0.338058851299519));
#54418=CARTESIAN_POINT('Ctrl Pts',(-0.141223581330571,0.691051943005463,
-0.322201340723575));
#54419=CARTESIAN_POINT('Ctrl Pts',(-0.454261155256553,0.539577325634538,
-0.306343830147631));
#54420=CARTESIAN_POINT('Ctrl Pts',(-0.65687187079242,0.256936244576825,
-0.29048631957169));
#54421=CARTESIAN_POINT('Ctrl Pts',(-0.699802856556483,-0.0881637600130705,
-0.274628808995744));
#54422=CARTESIAN_POINT('Ctrl Pts',(-0.572617975996934,-0.411831935255785,
-0.258771298419802));
#54423=CARTESIAN_POINT('Ctrl Pts',(-0.306234735283331,-0.635387420227233,
-0.242913787843858));
#54424=CARTESIAN_POINT('Ctrl Pts',(0.0345914406976117,-0.704485853085711,
-0.227056277267915));
#54425=CARTESIAN_POINT('Ctrl Pts',(0.367008771067512,-0.602330028183672,
-0.21119876669197));
#54426=CARTESIAN_POINT('Ctrl Pts',(0.610209470489882,-0.353753099832041,
-0.195341256116028));
#54427=CARTESIAN_POINT('Ctrl Pts',(0.705073760608792,-0.0191819564521373,
-0.179483745540084));
#54428=CARTESIAN_POINT('Ctrl Pts',(0.62854066985661,0.320052203509621,-0.16362623496414));
#54429=CARTESIAN_POINT('Ctrl Pts',(0.399215307462047,0.58148440677362,-0.147768724388197));
#54430=CARTESIAN_POINT('Ctrl Pts',(0.0728434763577143,0.701563108700217,
-0.131911213812254));
#54431=CARTESIAN_POINT('Ctrl Pts',(-0.271234459526246,0.651097643395513,
-0.11605370323631));
#54432=CARTESIAN_POINT('Ctrl Pts',(-0.549380630953683,0.442356886629713,
-0.100196192660368));
#54433=CARTESIAN_POINT('Ctrl Pts',(-0.693971520902736,0.126081582258689,
-0.084338682084424));
#54434=CARTESIAN_POINT('Ctrl Pts',(-0.669875267596679,-0.220840084321447,
-0.0684811715084805));
#54435=CARTESIAN_POINT('Ctrl Pts',(-0.482916401293059,-0.514083268386795,
-0.0526236609325368));
#54436=CARTESIAN_POINT('Ctrl Pts',(-0.178607888241887,-0.68234590671203,
-0.0367661503565942));
#54437=CARTESIAN_POINT('Ctrl Pts',(0.169206013737912,-0.684760397665597,
-0.0209086397806501));
#54438=CARTESIAN_POINT('Ctrl Pts',(0.373522557112378,-0.575353242974678,
-0.0103369660633542));
#54439=CARTESIAN_POINT('Ctrl Pts',(0.456477694810146,-0.499550802362297,
-0.00505112920470641));
#54440=CARTESIAN_POINT('Ctrl Pts',(0.533647856309019,-0.584002718706676,
-0.0710999999999995));
#54441=CARTESIAN_POINT('Ctrl Pts',(0.43666867878175,-0.672619994853351,
-0.0763858368586472));
#54442=CARTESIAN_POINT('Ctrl Pts',(0.3172399677846,-0.736571524390805,-0.0816716737172953));
#54443=CARTESIAN_POINT('Ctrl Pts',(0.189756640842203,-0.768076843419576,
-0.0869575105759432));
#54444=CARTESIAN_POINT('Ctrl Pts',(0.0622733138997992,-0.79958216244835,
-0.0922433474345914));
#54445=CARTESIAN_POINT('Ctrl Pts',(-0.073264628987864,-0.798641270968439,
-0.09752918429324));
#54446=CARTESIAN_POINT('Ctrl Pts',(-0.200325867973879,-0.765386092166293,
-0.102815021151888));
#54447=CARTESIAN_POINT('Ctrl Pts',(-0.327387106959887,-0.732130913364149,
-0.108100858010536));
#54448=CARTESIAN_POINT('Ctrl Pts',(-0.445971642044243,-0.666561447239783,
-0.113386694869182));
#54449=CARTESIAN_POINT('Ctrl Pts',(-0.541691464665684,-0.576640444310574,
-0.11867253172783));
#54450=CARTESIAN_POINT('Ctrl Pts',(-0.637411287287125,-0.486719441381364,
-0.123958368586478));
#54451=CARTESIAN_POINT('Ctrl Pts',(-0.71026639744564,-0.372446901647311,
-0.129244205445126));
#54452=CARTESIAN_POINT('Ctrl Pts',(-0.751388929617263,-0.24771550581813,
-0.134530042303774));
#54453=CARTESIAN_POINT('Ctrl Pts',(-0.777676231444153,-0.167981800807776,
-0.137908977927949));
#54454=CARTESIAN_POINT('Ctrl Pts',(-0.790996587895958,-0.0839742729858109,
-0.141287913552124));
#54455=CARTESIAN_POINT('Ctrl Pts',(-0.791053554504038,1.52922707510328E-5,
-0.144666849176299));
#54456=CARTESIAN_POINT('Origin',(0.,0.,-0.599));
#54457=CARTESIAN_POINT('',(0.23094010767585,-0.4,-0.599));
#54458=CARTESIAN_POINT('',(-0.230940107675851,-0.4,-0.599));
#54459=CARTESIAN_POINT('',(0.115470053837925,-0.4,-0.599));
#54460=CARTESIAN_POINT('Origin',(0.,0.,-0.599));
#54461=CARTESIAN_POINT('Origin',(0.,0.,-0.599));
#54462=CARTESIAN_POINT('',(-0.461880215351701,1.11022302462516E-16,-0.599));
#54463=CARTESIAN_POINT('',(-0.288675134594813,-0.3,-0.599));
#54464=CARTESIAN_POINT('Origin',(0.,0.,-0.599));
#54465=CARTESIAN_POINT('Origin',(0.,0.,-0.599));
#54466=CARTESIAN_POINT('',(-0.23094010767585,0.4,-0.599));
#54467=CARTESIAN_POINT('',(-0.404145188432738,0.1,-0.599));
#54468=CARTESIAN_POINT('Origin',(0.,0.,-0.599));
#54469=CARTESIAN_POINT('Origin',(0.,0.,-0.599));
#54470=CARTESIAN_POINT('',(0.23094010767585,0.4,-0.599));
#54471=CARTESIAN_POINT('',(-0.115470053837925,0.4,-0.599));
#54472=CARTESIAN_POINT('Origin',(0.,0.,-0.599));
#54473=CARTESIAN_POINT('Origin',(0.,0.,-0.599));
#54474=CARTESIAN_POINT('',(0.461880215351701,0.,-0.599));
#54475=CARTESIAN_POINT('',(0.288675134594813,0.3,-0.599));
#54476=CARTESIAN_POINT('Origin',(0.,0.,-0.599));
#54477=CARTESIAN_POINT('Origin',(0.,0.,-0.599));
#54478=CARTESIAN_POINT('',(0.404145188432738,-0.1,-0.599));
#54479=CARTESIAN_POINT('Origin',(0.,0.,-0.599));
#54480=CARTESIAN_POINT('Origin',(0.,0.,-0.73806406460551));
#54481=CARTESIAN_POINT('',(0.,0.,-0.87712812921102));
#54482=CARTESIAN_POINT('',(-0.460219541126976,-5.63606387946214E-17,-0.6));
#54483=CARTESIAN_POINT('',(-0.23094010767585,-2.82820063659975E-17,-0.73806406460551));
#54484=CARTESIAN_POINT('',(-0.460210453731243,-0.00289211196316049,-0.6));
#54485=CARTESIAN_POINT('Origin',(0.,0.,-0.6));
#54486=CARTESIAN_POINT('Ctrl Pts',(-0.4618802153517,-6.93889390390722E-16,
-0.599));
#54487=CARTESIAN_POINT('Ctrl Pts',(-0.461043830945924,-0.00144866028546382,
-0.599503641468823));
#54488=CARTESIAN_POINT('Ctrl Pts',(-0.460210453731243,-0.00289211196316079,
-0.6));
#54489=CARTESIAN_POINT('',(-0.232609869296308,-0.397107888036839,-0.6));
#54490=CARTESIAN_POINT('Ctrl Pts',(-0.232609869296308,-0.397107888036839,
-0.6));
#54491=CARTESIAN_POINT('Ctrl Pts',(-0.231776492081632,-0.398551339714529,
-0.599503641468825));
#54492=CARTESIAN_POINT('Ctrl Pts',(-0.230940107675851,-0.399999999999999,
-0.599));
#54493=CARTESIAN_POINT('',(-0.227600584434936,-0.4,-0.6));
#54494=CARTESIAN_POINT('Origin',(0.,0.,-0.6));
#54495=CARTESIAN_POINT('Ctrl Pts',(-0.23094010767585,-0.4,-0.599));
#54496=CARTESIAN_POINT('Ctrl Pts',(-0.229267338864258,-0.4,-0.599503641468835));
#54497=CARTESIAN_POINT('Ctrl Pts',(-0.227600584434936,-0.4,-0.6));
#54498=CARTESIAN_POINT('',(0.227600584434936,-0.4,-0.6));
#54499=CARTESIAN_POINT('Ctrl Pts',(0.227600584434936,-0.4,-0.6));
#54500=CARTESIAN_POINT('Ctrl Pts',(0.229267338864223,-0.4,-0.599503641468845));
#54501=CARTESIAN_POINT('Ctrl Pts',(0.23094010767585,-0.4,-0.599));
#54502=CARTESIAN_POINT('',(0.232609869296308,-0.397107888036839,-0.6));
#54503=CARTESIAN_POINT('Origin',(0.,0.,-0.6));
#54504=CARTESIAN_POINT('Ctrl Pts',(0.230940107675851,-0.399999999999999,
-0.599));
#54505=CARTESIAN_POINT('Ctrl Pts',(0.231776492081654,-0.39855133971449,
-0.599503641468839));
#54506=CARTESIAN_POINT('Ctrl Pts',(0.232609869296308,-0.397107888036839,
-0.6));
#54507=CARTESIAN_POINT('',(0.460210453731243,-0.0028921119631606,-0.6));
#54508=CARTESIAN_POINT('Ctrl Pts',(0.460210453731243,-0.00289211196316057,
-0.6));
#54509=CARTESIAN_POINT('Ctrl Pts',(0.461043830945901,-0.00144866028550258,
-0.599503641468836));
#54510=CARTESIAN_POINT('Ctrl Pts',(0.4618802153517,-7.21644966006351E-16,
-0.599));
#54511=CARTESIAN_POINT('',(0.460210453731243,0.0028921119631606,-0.6));
#54512=CARTESIAN_POINT('Origin',(0.,0.,-0.6));
#54513=CARTESIAN_POINT('Ctrl Pts',(0.4618802153517,9.15933995315753E-16,
-0.599));
#54514=CARTESIAN_POINT('Ctrl Pts',(0.461043830945894,0.00144866028551485,
-0.59950364146884));
#54515=CARTESIAN_POINT('Ctrl Pts',(0.460210453731243,0.0028921119631606,
-0.6));
#54516=CARTESIAN_POINT('',(0.232609869296308,0.397107888036839,-0.6));
#54517=CARTESIAN_POINT('Ctrl Pts',(0.232609869296308,0.397107888036839,
-0.6));
#54518=CARTESIAN_POINT('Ctrl Pts',(0.231776492081656,0.398551339714487,
-0.59950364146884));
#54519=CARTESIAN_POINT('Ctrl Pts',(0.230940107675851,0.399999999999999,
-0.599));
#54520=CARTESIAN_POINT('',(0.227600584434936,0.4,-0.6));
#54521=CARTESIAN_POINT('Origin',(0.,0.,-0.6));
#54522=CARTESIAN_POINT('Ctrl Pts',(0.23094010767585,0.4,-0.599));
#54523=CARTESIAN_POINT('Ctrl Pts',(0.229267338864267,0.4,-0.599503641468832));
#54524=CARTESIAN_POINT('Ctrl Pts',(0.227600584434936,0.4,-0.6));
#54525=CARTESIAN_POINT('',(-0.227600584434936,0.4,-0.6));
#54526=CARTESIAN_POINT('Ctrl Pts',(-0.227600584434935,0.4,-0.6));
#54527=CARTESIAN_POINT('Ctrl Pts',(-0.22926733886426,0.4,-0.599503641468834));
#54528=CARTESIAN_POINT('Ctrl Pts',(-0.230940107675849,0.4,-0.599));
#54529=CARTESIAN_POINT('',(-0.232609869296308,0.397107888036839,-0.6));
#54530=CARTESIAN_POINT('Origin',(0.,0.,-0.6));
#54531=CARTESIAN_POINT('Ctrl Pts',(-0.230940107675851,0.399999999999999,
-0.599));
#54532=CARTESIAN_POINT('Ctrl Pts',(-0.231776492081655,0.398551339714488,
-0.599503641468839));
#54533=CARTESIAN_POINT('Ctrl Pts',(-0.232609869296308,0.397107888036839,
-0.6));
#54534=CARTESIAN_POINT('',(-0.460210453731243,0.00289211196316071,-0.6));
#54535=CARTESIAN_POINT('Ctrl Pts',(-0.460210453731243,0.00289211196316076,
-0.6));
#54536=CARTESIAN_POINT('Ctrl Pts',(-0.461043830945898,0.00144866028550932,
-0.599503641468838));
#54537=CARTESIAN_POINT('Ctrl Pts',(-0.4618802153517,9.15933995315753E-16,
-0.599));
#54538=CARTESIAN_POINT('Origin',(0.,0.,-0.6));
#54539=CARTESIAN_POINT('Origin',(-0.461880215351701,5.55111512312578E-17,
0.));
#54540=CARTESIAN_POINT('',(-0.23094010767585,0.4,0.));
#54541=CARTESIAN_POINT('',(-0.23094010767585,0.4,0.));
#54542=CARTESIAN_POINT('',(-0.461880215351701,5.6564012731995E-17,0.));
#54543=CARTESIAN_POINT('',(-0.404145188432738,0.1,0.));
#54544=CARTESIAN_POINT('',(-0.461880215351701,5.6564012731995E-17,0.));
#54545=CARTESIAN_POINT('Origin',(-0.461880215351701,5.55111512312578E-17,
0.));
#54546=CARTESIAN_POINT('',(-0.461880215351701,5.55111512312578E-17,-0.6));
#54547=CARTESIAN_POINT('',(-0.461880215351701,5.6564012731995E-17,0.));
#54548=CARTESIAN_POINT('',(-0.23094010767585,0.4,-0.6));
#54549=CARTESIAN_POINT('Origin',(-0.23094010767585,0.4,0.));
#54550=CARTESIAN_POINT('',(0.23094010767585,0.4,0.));
#54551=CARTESIAN_POINT('',(0.23094010767585,0.4,0.));
#54552=CARTESIAN_POINT('',(-0.115470053837925,0.4,0.));
#54553=CARTESIAN_POINT('Origin',(-0.23094010767585,0.4,0.));
#54554=CARTESIAN_POINT('',(0.23094010767585,0.4,-0.6));
#54555=CARTESIAN_POINT('',(0.23094010767585,0.4,-0.6));
#54556=CARTESIAN_POINT('',(0.23094010767585,0.4,0.));
#54557=CARTESIAN_POINT('Origin',(-0.23094010767585,0.4,0.));
#54558=CARTESIAN_POINT('',(-0.23094010767585,0.4,-0.6));
#54559=CARTESIAN_POINT('',(-0.23094010767585,0.4,0.));
#54560=CARTESIAN_POINT('',(0.23094010767585,0.4,-0.6));
#54561=CARTESIAN_POINT('Origin',(-0.230940107675851,-0.4,0.));
#54562=CARTESIAN_POINT('',(-0.230940107675851,-0.4,0.));
#54563=CARTESIAN_POINT('',(-0.288675134594813,-0.3,0.));
#54564=CARTESIAN_POINT('',(-0.230940107675851,-0.4,0.));
#54565=CARTESIAN_POINT('Origin',(-0.230940107675851,-0.4,0.));
#54566=CARTESIAN_POINT('',(-0.230940107675851,-0.4,-0.6));
#54567=CARTESIAN_POINT('',(-0.230940107675851,-0.4,0.));
#54568=CARTESIAN_POINT('',(-0.461880215351701,5.6564012731995E-17,-0.6));
#54569=CARTESIAN_POINT('Origin',(0.23094010767585,0.4,0.));
#54570=CARTESIAN_POINT('',(0.461880215351701,0.,0.));
#54571=CARTESIAN_POINT('',(0.461880215351701,0.,0.));
#54572=CARTESIAN_POINT('',(0.288675134594813,0.3,0.));
#54573=CARTESIAN_POINT('Origin',(0.23094010767585,0.4,0.));
#54574=CARTESIAN_POINT('',(0.461880215351701,0.,-0.6));
#54575=CARTESIAN_POINT('',(0.461880215351701,0.,-0.6));
#54576=CARTESIAN_POINT('',(0.461880215351701,0.,0.));
#54577=CARTESIAN_POINT('Origin',(0.23094010767585,0.4,0.));
#54578=CARTESIAN_POINT('',(0.461880215351701,0.,-0.6));
#54579=CARTESIAN_POINT('Origin',(0.,0.,-0.6));
#54580=CARTESIAN_POINT('',(-0.23094010767585,0.4,-0.6));
#54581=CARTESIAN_POINT('Origin',(0.,0.,-0.6));
#54582=CARTESIAN_POINT('Origin',(0.,0.,-0.6));
#54583=CARTESIAN_POINT('',(0.23094010767585,-0.4,-0.6));
#54584=CARTESIAN_POINT('Origin',(0.,0.,-0.6));
#54585=CARTESIAN_POINT('',(0.23094010767585,-0.4,-0.6));
#54586=CARTESIAN_POINT('',(-0.230940107675851,-0.4,-0.6));
#54587=CARTESIAN_POINT('',(0.23094010767585,-0.4,-0.6));
#54588=CARTESIAN_POINT('Origin',(0.,0.,-0.6));
#54589=CARTESIAN_POINT('',(-0.230940107675851,-0.4,-0.6));
#54590=CARTESIAN_POINT('Origin',(0.,0.,-0.6));
#54591=CARTESIAN_POINT('',(-0.461880215351701,5.6564012731995E-17,-0.6));
#54592=CARTESIAN_POINT('Origin',(0.461880215351701,0.,0.));
#54593=CARTESIAN_POINT('',(0.23094010767585,-0.4,0.));
#54594=CARTESIAN_POINT('',(0.23094010767585,-0.4,0.));
#54595=CARTESIAN_POINT('',(0.404145188432738,-0.1,0.));
#54596=CARTESIAN_POINT('Origin',(0.461880215351701,0.,0.));
#54597=CARTESIAN_POINT('',(0.23094010767585,-0.4,0.));
#54598=CARTESIAN_POINT('Origin',(0.461880215351701,0.,0.));
#54599=CARTESIAN_POINT('Origin',(0.23094010767585,-0.4,0.));
#54600=CARTESIAN_POINT('Origin',(0.23094010767585,-0.4,0.));
#54601=CARTESIAN_POINT('',(0.115470053837925,-0.4,0.));
#54602=CARTESIAN_POINT('Origin',(-0.461880215351701,5.55111512312578E-17,
0.));
#54603=CARTESIAN_POINT('Origin',(-0.230940107675851,-0.4,0.));
#54604=CARTESIAN_POINT('Origin',(0.23094010767585,-0.4,0.));
#54605=CARTESIAN_POINT('Origin',(0.6,0.,-6.));
#54606=CARTESIAN_POINT('',(-0.6,-7.34788079488412E-17,-6.));
#54607=CARTESIAN_POINT('Origin',(0.,0.,-6.));
#54608=CARTESIAN_POINT('Origin',(0.,0.,-5.9));
#54609=CARTESIAN_POINT('',(-0.7,-8.57252759403147E-17,-5.9));
#54610=CARTESIAN_POINT('Origin',(0.,0.,-2.94));
#54611=CARTESIAN_POINT('Origin',(0.,0.,-0.0711000000000004));
#54612=CARTESIAN_POINT('Origin',(0.,0.,-0.04));
#54613=CARTESIAN_POINT('',(-0.72,-8.81745695386094E-17,-6.93889390390723E-18));
#54614=CARTESIAN_POINT('Origin',(0.,0.,0.));
#54615=CARTESIAN_POINT('',(-0.76,-9.30731567351988E-17,-0.04));
#54616=CARTESIAN_POINT('Origin',(0.,0.,0.));
#70732=UNCERTAINTY_MEASURE_WITH_UNIT(LENGTH_MEASURE(0.001),#70758,
'DISTANCE_ACCURACY_VALUE',
'Maximum model space distance between geometric entities at asserted c
onnectivities');
#70740=UNCERTAINTY_MEASURE_WITH_UNIT(LENGTH_MEASURE(0.001),#70758,
'DISTANCE_ACCURACY_VALUE',
'Maximum model space distance between geometric entities at asserted c
onnectivities');
#70749=(
GEOMETRIC_REPRESENTATION_CONTEXT(3)
GLOBAL_UNCERTAINTY_ASSIGNED_CONTEXT((#70732))
GLOBAL_UNIT_ASSIGNED_CONTEXT((#70758,#70760,#70761))
REPRESENTATION_CONTEXT('','3D')
);
#70757=(
GEOMETRIC_REPRESENTATION_CONTEXT(3)
GLOBAL_UNCERTAINTY_ASSIGNED_CONTEXT((#70740))
GLOBAL_UNIT_ASSIGNED_CONTEXT((#70758,#70760,#70761))
REPRESENTATION_CONTEXT('','3D')
);
#70758=(
LENGTH_UNIT()
NAMED_UNIT(*)
SI_UNIT(.CENTI.,.METRE.)
);
#70760=(
NAMED_UNIT(*)
PLANE_ANGLE_UNIT()
SI_UNIT($,.RADIAN.)
);
#70761=(
NAMED_UNIT(*)
SI_UNIT($,.STERADIAN.)
SOLID_ANGLE_UNIT()
);
#70770=SHAPE_DEFINITION_REPRESENTATION(#70786,#70825);
#70786=PRODUCT_DEFINITION_SHAPE('',$,#70842);
#70825=SHAPE_REPRESENTATION('',(#27547),#70749);
#70833=PRODUCT_DEFINITION_CONTEXT('part definition',#70883,'design');
#70842=PRODUCT_DEFINITION('2026-10-19-02-55-56-496',
'11_ISO_4026_M16x60_Gib_Adjust_Set_Screw',#70858,#70833);
#70858=PRODUCT_DEFINITION_FORMATION('',$,#70893);
#70883=APPLICATION_CONTEXT(
'Core Data for Automotive Mechanical Design Process');
#70884=PRODUCT_CONTEXT('part definition',#70883,'mechanical');
#70893=PRODUCT('2026-10-19-02-55-56-496',
'11_ISO_4026_M16x60_Gib_Adjust_Set_Screw',$,(#70884));
#71048=COLOUR_RGB('Black',0.12,0.14,0.17);
#71049=FILL_AREA_STYLE_COLOUR('',#71048);
#71050=FILL_AREA_STYLE('',(#71049));
#71051=SURFACE_STYLE_FILL_AREA(#71050);
#71052=SURFACE_SIDE_STYLE('',(#71051));
#71053=SURFACE_STYLE_USAGE(.BOTH.,#71052);
#71054=PRESENTATION_STYLE_ASSIGNMENT((#71053));
ENDSEC;
END-ISO-10303-21;
